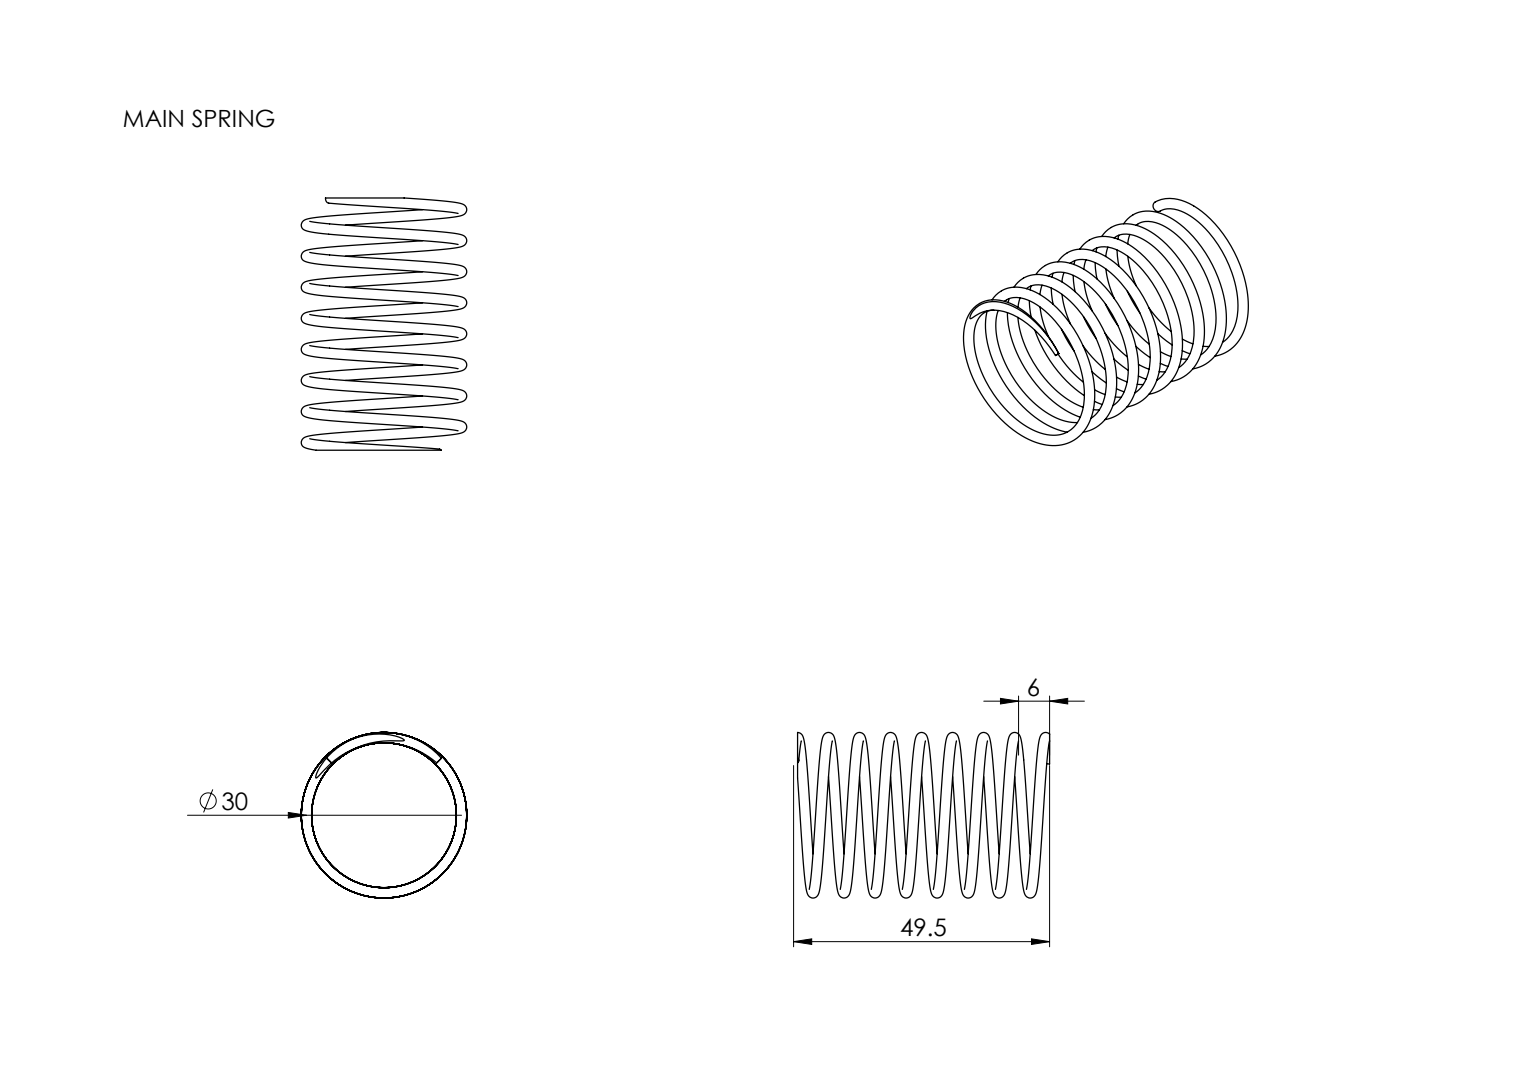
ISO-10303-21;
HEADER;
FILE_DESCRIPTION (('STEP AP214'),
    '1' );
FILE_NAME ('main spring.step',
    '2026-10-08T13:22:57',
    ( '' ),
    ( '' ),
    'SwSTEP 2.0',
    'SolidWorks 2026',
    '' );
FILE_SCHEMA (( 'AUTOMOTIVE_DESIGN' ));
ENDSEC;

DATA;
#2=CARTESIAN_POINT ( 'NONE',  ( 8.512513224245308763, 13.54758718765259040, 13.28571428571429003 ) ) ;
#5=CARTESIAN_POINT ( 'NONE',  ( -14.28433602490915000, 1.478298951650542481, 25.35310228751642470 ) ) ;
#11=CARTESIAN_POINT ( 'NONE',  ( -11.92174236212692051, -7.340858601238089420, 8.718326283912148256 ) ) ;
#12=CARTESIAN_POINT ( 'NONE',  ( 13.17239914596754424, -4.743843029824685864, 18.57546914105500235 ) ) ;
#15=CARTESIAN_POINT ( 'NONE',  ( 15.44746603149413922, 5.543385399275817527, 15.92453085894499409 ) ) ;
#16=COLOUR_RGB ( '', 0.40784314, 0.44705882, 0.49803922) ;
#20=CARTESIAN_POINT ( 'NONE',  ( 11.31370849898482334, -11.31370849898469366, 45.00000000000000711 ) ) ;
#25=CARTESIAN_POINT ( 'NONE',  ( -8.731428362939189114, 13.89598863503036341, 36.21428571428573662 ) ) ;
#28=CARTESIAN_POINT ( 'NONE',  ( -11.22385875690717327, 11.40355824106234550, 28.00404056962643651 ) ) ;
#30=CARTESIAN_POINT ( 'NONE',  ( -1.837501619626328297, 16.30827793483733856, 12.64285714285714235 ) ) ;
#35=CARTESIAN_POINT ( 'NONE',  ( -13.92619789766827054, -1.441234910513399470, 45.14689771248358596 ) ) ;
#36=CARTESIAN_POINT ( 'NONE',  ( 8.512513224245308763, 13.54758718765259040, 19.28571428571428825 ) ) ;
#38=CARTESIAN_POINT ( 'NONE',  ( -7.639999817571786700, 12.15899005565156266, 36.21428571428572951 ) ) ;
#39=CARTESIAN_POINT ( 'NONE',  ( 9.809645194534072132, -9.989344678689256796, 31.00404056962644006 ) ) ;
#43=CARTESIAN_POINT ( 'NONE',  ( 1.441234910513245149, 13.92619789766829008, 50.85310228751642825 ) ) ;
#46=CARTESIAN_POINT ( 'NONE',  ( 11.60466159355861926, 11.60466159355874716, 13.50000000000000355 ) ) ;
#48=CARTESIAN_POINT ( 'NONE',  ( -13.96533075980324234, 8.621071003556515677, 19.78167371608784819 ) ) ;
#53=FILL_AREA_STYLE_COLOUR ( '', #3926 ) ;
#56=CARTESIAN_POINT ( 'NONE',  ( 1.791431617652837316, 15.89939535829188877, 12.85714285714285943 ) ) ;
#59=CARTESIAN_POINT ( 'NONE',  ( 1.441234910513245149, 13.92619789766829008, 26.85310228751642470 ) ) ;
#63=CARTESIAN_POINT ( 'NONE',  ( 13.17239914596754424, -4.743843029824685864, 12.57546914105500768 ) ) ;
#64=CARTESIAN_POINT ( 'NONE',  ( -1.478298951650703019, 14.28433602490913579, 10.64689771248357886 ) ) ;
#68=CARTESIAN_POINT ( 'NONE',  ( 15.89939535829187278, 1.791431617653015174, 44.14285714285714590 ) ) ;
#77=CARTESIAN_POINT ( 'NONE',  ( -5.543385399275643444, -15.44746603149420494, 38.07546914105502367 ) ) ;
#79=CARTESIAN_POINT ( 'NONE',  ( -13.54758718765249625, -8.512513224245459753, 34.71428571428571530 ) ) ;
#80=CARTESIAN_POINT ( 'NONE',  ( 2.336471713481377055, 15.82515143223400145, 48.73000000000002530 ) ) ;
#82=SURFACE_STYLE_USAGE ( .BOTH. , #1640 ) ;
#85=CARTESIAN_POINT ( 'NONE',  ( -1.693770420379220099, -13.89774397934251837, 43.86118342676930126 ) ) ;
#86=CARTESIAN_POINT ( 'NONE',  ( 16.30827793483735633, -1.837501619626142890, 20.35714285714286476 ) ) ;
#87=CARTESIAN_POINT ( 'NONE',  ( -4.742819248065500481, -13.55419868402813499, 34.07142857142857650 ) ) ;
#88=CARTESIAN_POINT ( 'NONE',  ( -5.164528828830334817, 15.14410076328347543, -1.567388001802134223 ) ) ;
#89=CARTESIAN_POINT ( 'NONE',  ( -14.26974319298268767, 1.607813917172874918, 5.357142857142856762 ) ) ;
#93=CARTESIAN_POINT ( 'NONE',  ( -11.85413878919593422, -7.448449071214776396, 4.714285714285712636 ) ) ;
#96=CARTESIAN_POINT ( 'NONE',  ( -8.512513224245306986, -13.54758718765259218, 16.28571428571428470 ) ) ;
#97=CARTESIAN_POINT ( 'NONE',  ( -16.32287076676382398, 1.707986654103809343, 43.35310228751642825 ) ) ;
#101=CARTESIAN_POINT ( 'NONE',  ( 4.742819248065502258, 13.55419868402813499, 1.071428571428570065 ) ) ;
#104=CARTESIAN_POINT ( 'NONE',  ( -10.06191849875405531, -10.24623928997363542, 12.49595943037356349 ) ) ;
#107=CARTESIAN_POINT ( 'NONE',  ( 7.750357176954296712, -12.08964793087877787, 41.21024514465928235 ) ) ;
#112=CARTESIAN_POINT ( 'NONE',  ( -7.556039541191334585, -11.78653521626503320, 2.289754855340722539 ) ) ;
#114=CARTESIAN_POINT ( 'NONE',  ( 7.556039541191335474, 11.78653521626503320, 11.28975485534071943 ) ) ;
#118=CARTESIAN_POINT ( 'NONE',  ( 11.60466159355862104, 11.60466159355875071, 37.50000000000002842 ) ) ;
#124=CARTESIAN_POINT ( 'NONE',  ( 16.29368510291089223, -1.967016585148476882, 30.36118342676929771 ) ) ;
#126=CARTESIAN_POINT ( 'NONE',  ( -11.22385875690717327, 11.40355824106234550, 34.00404056962644006 ) ) ;
#128=CARTESIAN_POINT ( 'NONE',  ( 8.731428362939190890, -13.89598863503036164, 33.21428571428571530 ) ) ;
#130=CARTESIAN_POINT ( 'NONE',  ( 11.60466159355862104, 11.60466159355875071, 1.500000000000003553 ) ) ;
#133=( NAMED_UNIT ( * ) PLANE_ANGLE_UNIT ( ) SI_UNIT ( $, .RADIAN. ) );
#136=CARTESIAN_POINT ( 'NONE',  ( 5.164528828830335705, -15.14410076328347543, 1.432611998197868219 ) ) ;
#137=CARTESIAN_POINT ( 'NONE',  ( -1.791431617652833763, -15.89939535829188877, 21.85714285714286120 ) ) ;
#138=CARTESIAN_POINT ( 'NONE',  ( -11.85413878919593422, -7.448449071214776396, 34.71428571428571530 ) ) ;
#139=CARTESIAN_POINT ( 'NONE',  ( -9.809645194534070356, 9.989344678689256796, 46.00404056962644006 ) ) ;
#140=CARTESIAN_POINT ( 'NONE',  ( -7.639999817571787588, 12.15899005565156266, 12.21428571428571885 ) ) ;
#144=CARTESIAN_POINT ( 'NONE',  ( -11.78653521626494793, -7.556039541191465148, 48.71024514465926814 ) ) ;
#148=CARTESIAN_POINT ( 'NONE',  ( 1.791431617652837316, 15.89939535829188877, 18.85714285714285765 ) ) ;
#149=CARTESIAN_POINT ( 'NONE',  ( -15.14410076328353227, 5.164528828830164287, 31.56738800180213644 ) ) ;
#153=FILL_AREA_STYLE ('',( #53 ) ) ;
#155=CARTESIAN_POINT ( 'NONE',  ( -1.441234910513241818, -13.92619789766829008, 11.85310228751642470 ) ) ;
#158=CARTESIAN_POINT ( 'NONE',  ( 7.340858601237956194, 11.92174236212700045, 45.28167371608785174 ) ) ;
#163=CARTESIAN_POINT ( 'NONE',  ( 4.865839792409144771, 13.51115193377589740, 17.07546914105500591 ) ) ;
#165=CARTESIAN_POINT ( 'NONE',  ( -11.92174236212692051, -7.340858601238089420, 8.718326283912148256 ) ) ;
#168=CARTESIAN_POINT ( 'NONE',  ( -5.404401153735176599, 15.06016580658422477, 14.42453085894499232 ) ) ;
#176=CARTESIAN_POINT ( 'NONE',  ( 8.621071003556677326, -13.96533075980314287, 31.21832628391215536 ) ) ;
#179=CARTESIAN_POINT ( 'NONE',  ( 8.620103694221997515, 13.47998361472160767, 29.28975485534071765 ) ) ;
#184=CARTESIAN_POINT ( 'NONE',  ( -15.89939535829186923, -1.791431617653016062, 29.14285714285714235 ) ) ;
#185=CARTESIAN_POINT ( 'NONE',  ( -1.732852372895761661, 14.17511762181074353, 2.529641460854714575E-15 ) ) ;
#186=CARTESIAN_POINT ( 'NONE',  ( -5.420364854931999155, -15.49051278174644253, 22.07142857142858006 ) ) ;
#194=CARTESIAN_POINT ( 'NONE',  ( 12.08964793087886314, -7.750357176954162597, 42.78975485534072476 ) ) ;
#195=CARTESIAN_POINT ( 'NONE',  ( 8.731428362939190890, -13.89598863503036164, 9.214285714285717077 ) ) ;
#197=CARTESIAN_POINT ( 'NONE',  ( 4.503970704919991519, -13.25633410266674517, 43.43261199819787066 ) ) ;
#198=CARTESIAN_POINT ( 'NONE',  ( -1.567502665446231180, -13.91197093850540334, 9.857142857142855874 ) ) ;
#202=CARTESIAN_POINT ( 'NONE',  ( 4.742819248065503146, 13.55419868402813677, 7.071428571428569398 ) ) ;
#205=CARTESIAN_POINT ( 'NONE',  ( -9.899494936611716867, 9.899494936611610285, 0.000000000000000000 ) ) ;
#207=CARTESIAN_POINT ( 'NONE',  ( 15.10213328493390783, -5.284464991282587398, 14.57142857142856940 ) ) ;
#208=CARTESIAN_POINT ( 'NONE',  ( 5.404401153735178376, -15.06016580658422477, 35.42453085894499765 ) ) ;
#215=CARTESIAN_POINT ( 'NONE',  ( 4.743843029824831525, -13.17239914596749095, 41.42453085894499765 ) ) ;
#219=CARTESIAN_POINT ( 'NONE',  ( -4.503970704919988854, 13.25633410266674517, 22.43261199819786356 ) ) ;
#220=CARTESIAN_POINT ( 'NONE',  ( -13.92619789766827054, -1.441234910513399470, 15.14689771248357708 ) ) ;
#223=CARTESIAN_POINT ( 'NONE',  ( -11.40355824106246807, 11.22385875690704715, 7.995959430373565269 ) ) ;
#229=CARTESIAN_POINT ( 'NONE',  ( 1.917699372585825790, 15.88516839912900203, 34.86118342676929416 ) ) ;
#230=CARTESIAN_POINT ( 'NONE',  ( -14.26974319298268767, 1.607813917172874918, 29.35714285714285765 ) ) ;
#232=CARTESIAN_POINT ( 'NONE',  ( 5.543385399275644332, 15.44746603149420494, 41.07546914105501656 ) ) ;
#234=AXIS2_PLACEMENT_3D ( 'NONE', #895, #1048, #264 ) ;
#235=CARTESIAN_POINT ( 'NONE',  ( 1.791431617652837316, 15.89939535829188877, 24.85714285714285765 ) ) ;
#236=CARTESIAN_POINT ( 'NONE',  ( -0.4153140463578967601, 14.34878908348401971, 2.773985284965652638E-17 ) ) ;
#237=CARTESIAN_POINT ( 'NONE',  ( -1.837501619626328297, 16.30827793483733856, 18.64285714285715656 ) ) ;
#241=CARTESIAN_POINT ( 'NONE',  ( 11.31370849898482334, -11.31370849898469366, 39.00000000000000000 ) ) ;
#243=CARTESIAN_POINT ( 'NONE',  ( 15.91362231745475597, 1.665163862720026255, 0.1468977124835755543 ) ) ;
#244=CARTESIAN_POINT ( 'NONE',  ( 13.54758718765249803, 8.512513224245457977, 31.71428571428571530 ) ) ;
#245=CARTESIAN_POINT ( 'NONE',  ( 0.000000000000000000, 0.000000000000000000, 0.000000000000000000 ) ) ;
#246=CARTESIAN_POINT ( 'NONE',  ( 7.529642458189280241, -12.22833218042435099, 43.21832628391217668 ) ) ;
#247=CARTESIAN_POINT ( 'NONE',  ( -13.91197093850538380, -1.567502665446387278, 17.14285714285713880 ) ) ;
#251=CARTESIAN_POINT ( 'NONE',  ( 10.15407889436379030, 10.15407889436390576, 19.50000000000000355 ) ) ;
#255=CARTESIAN_POINT ( 'NONE',  ( 5.420364854932000931, 15.49051278174644075, 13.07142857142857117 ) ) ;
#256=CARTESIAN_POINT ( 'NONE',  ( 1.665163862719847732, 15.91362231745477374, 38.85310228751641404 ) ) ;
#260=CARTESIAN_POINT ( 'NONE',  ( 10.15407889436379030, 10.15407889436390221, 7.500000000000004441 ) ) ;
#262=CARTESIAN_POINT ( 'NONE',  ( -7.340858601237953529, -11.92174236212700222, 24.28167371608785530 ) ) ;
#264=DIRECTION ( 'NONE',  ( 0.7071067811865432429, 0.7071067811865519026, 0.000000000000000000 ) ) ;
#265=CARTESIAN_POINT ( 'NONE',  ( 12.22833218042443271, -7.529642458189144349, 34.78167371608785885 ) ) ;
#271=CARTESIAN_POINT ( 'NONE',  ( 13.59724543428031573, 4.619798703722006294, 23.93261199819786711 ) ) ;
#275=CARTESIAN_POINT ( 'NONE',  ( 15.44746603149413922, 5.543385399275817527, 3.924530858944990541 ) ) ;
#281=CARTESIAN_POINT ( 'NONE',  ( -11.22385875690717327, 11.40355824106234550, 34.00404056962644006 ) ) ;
#282=CARTESIAN_POINT ( 'NONE',  ( -13.55419868402807992, -4.742819248065651472, 34.92857142857145192 ) ) ;
#284=CARTESIAN_POINT ( 'NONE',  ( -4.742819248065502258, -13.55419868402813677, 34.07142857142859071 ) ) ;
#287=CARTESIAN_POINT ( 'NONE',  ( -5.420364854931999155, -15.49051278174644253, 28.07142857142857295 ) ) ;
#288=CARTESIAN_POINT ( 'NONE',  ( -3.668565799300981034, 13.66277435358085235, 2.529641460854714969E-15 ) ) ;
#289=CARTESIAN_POINT ( 'NONE',  ( -8.512513224245306986, -13.54758718765259218, 10.28571428571428648 ) ) ;
#294=CARTESIAN_POINT ( 'NONE',  ( -8.621071003556675549, 13.96533075980314642, 16.21832628391214470 ) ) ;
#295=CARTESIAN_POINT ( 'NONE',  ( 13.89598863503046111, -8.731428362939032795, 32.78571428571430602 ) ) ;
#298=CARTESIAN_POINT ( 'NONE',  ( -5.543385399275643444, -15.44746603149420494, 8.075469141055007682 ) ) ;
#299=CARTESIAN_POINT ( 'NONE',  ( -14.26974319298268767, 1.607813917172874918, 11.35714285714285943 ) ) ;
#303=CARTESIAN_POINT ( 'NONE',  ( -10.15407889436378852, -10.15407889436390576, 10.50000000000000533 ) ) ;
#305=CARTESIAN_POINT ( 'NONE',  ( 15.89939535829187278, 1.791431617653015174, 32.14285714285714590 ) ) ;
#306=CARTESIAN_POINT ( 'NONE',  ( 11.51250119794888249, 11.69682198916847682, 33.49595943037355994 ) ) ;
#309=CARTESIAN_POINT ( 'NONE',  ( -1.567502665446231180, -13.91197093850540334, 9.857142857142855874 ) ) ;
#312=CARTESIAN_POINT ( 'NONE',  ( 13.89774397934249706, 1.693770420379375308, 22.13881657323070939 ) ) ;
#315=CARTESIAN_POINT ( 'NONE',  ( 4.743843029824831525, -13.17239914596749095, 35.42453085894499765 ) ) ;
#320=CARTESIAN_POINT ( 'NONE',  ( -11.40355824106246807, 11.22385875690704715, 43.99595943037355994 ) ) ;
#322=CARTESIAN_POINT ( 'NONE',  ( -12.95959046474881227, 7.269551181504937176, 48.73000000000000398 ) ) ;
#323=CARTESIAN_POINT ( 'NONE',  ( 15.89939535829187278, 1.791431617653015174, 20.14285714285714235 ) ) ;
#324=CARTESIAN_POINT ( 'NONE',  ( 16.32287076676382043, -1.707986654103810897, 16.35310228751641759 ) ) ;
#332=CARTESIAN_POINT ( 'NONE',  ( 13.82664651025767100, -8.841785722321541030, 36.78975485534072476 ) ) ;
#333=CARTESIAN_POINT ( 'NONE',  ( 7.448449071214646722, 11.85413878919601594, 37.28571428571429180 ) ) ;
#334=CARTESIAN_POINT ( 'NONE',  ( -9.899494936611716867, 9.899494936611610285, 42.00000000000000000 ) ) ;
#337=CARTESIAN_POINT ( 'NONE',  ( -11.60466159355861926, -11.60466159355875249, 40.50000000000000711 ) ) ;
#338=CARTESIAN_POINT ( 'NONE',  ( -5.853818627049699685, 14.80933238498958282, -1.389475189636273717E-15 ) ) ;
#340=CARTESIAN_POINT ( 'NONE',  ( -15.89939535829186923, -1.791431617653016062, 23.14285714285714590 ) ) ;
#344=CARTESIAN_POINT ( 'NONE',  ( -11.69682198916834892, -11.51250119794901394, 8.504040569626438284 ) ) ;
#346=CARTESIAN_POINT ( 'NONE',  ( 15.49051278174638036, 5.420364854932175014, 25.92857142857142705 ) ) ;
#350=CARTESIAN_POINT ( 'NONE',  ( -1.707986654103994528, 16.32287076676380266, 10.64689771248357886 ) ) ;
#351=CARTESIAN_POINT ( 'NONE',  ( 13.91197093850538380, 1.567502665446386390, 26.14285714285714590 ) ) ;
#352=CARTESIAN_POINT ( 'NONE',  ( 16.30827793483735633, -1.837501619626142890, 8.357142857142855874 ) ) ;
#355=CARTESIAN_POINT ( 'NONE',  ( -13.91197093850538380, -1.567502665446387278, 17.14285714285713880 ) ) ;
#359=CARTESIAN_POINT ( 'NONE',  ( 11.31370849898482334, -11.31370849898469366, 27.00000000000000355 ) ) ;
#360=CARTESIAN_POINT ( 'NONE',  ( 1.665163862719847732, 15.91362231745477374, 50.85310228751642825 ) ) ;
#362=CARTESIAN_POINT ( 'NONE',  ( -13.55419868402807992, -4.742819248065651472, 10.92857142857143060 ) ) ;
#363=CARTESIAN_POINT ( 'NONE',  ( 11.78653521626494793, 7.556039541191463371, 33.71024514465927524 ) ) ;
#368=CARTESIAN_POINT ( 'NONE',  ( -1.737328882695368115, 14.25515036105620581, 50.63881657323071295 ) ) ;
#369=AXIS2_PLACEMENT_3D ( 'NONE', #442, #2961, #1373 ) ;
#373=CARTESIAN_POINT ( 'NONE',  ( -12.08964793087886314, 7.750357176954159932, 21.78975485534072476 ) ) ;
#375=CARTESIAN_POINT ( 'NONE',  ( 10.24623928997352884, 10.06191849875416899, 23.50404056962643295 ) ) ;
#377=CARTESIAN_POINT ( 'NONE',  ( 8.404922754268618235, 13.61519076058357491, 45.28167371608785174 ) ) ;
#378=EDGE_LOOP ( 'NONE', ( #1327, #9826 ) ) ;
#379=CARTESIAN_POINT ( 'NONE',  ( -11.25295468363732709, 9.057666965552700233, 48.73000000000003951 ) ) ;
#385=CARTESIAN_POINT ( 'NONE',  ( 4.742819248065503146, 13.55419868402813677, 25.07142857142858361 ) ) ;
#387=CARTESIAN_POINT ( 'NONE',  ( 4.742819248065503146, 13.55419868402813677, 43.07142857142858361 ) ) ;
#389=CARTESIAN_POINT ( 'NONE',  ( -5.284464991282755264, 15.10213328493384743, 42.42857142857143060 ) ) ;
#391=CARTESIAN_POINT ( 'NONE',  ( -11.60466159355861926, -11.60466159355875249, 10.50000000000000533 ) ) ;
#393=PRODUCT_DEFINITION_SHAPE ( 'NONE', 'NONE',  #8011 ) ;
#399=CARTESIAN_POINT ( 'NONE',  ( 1.917699372585825790, 15.88516839912900203, 4.861183426769296823 ) ) ;
#400=CARTESIAN_POINT ( 'NONE',  ( -8.731428362939189114, 13.89598863503036341, 36.21428571428573662 ) ) ;
#403=CARTESIAN_POINT ( 'NONE',  ( 5.543385399275644332, 15.44746603149420494, 11.07546914105500768 ) ) ;
#404=CARTESIAN_POINT ( 'NONE',  ( 7.448449071214646722, 11.85413878919601594, 19.28571428571428825 ) ) ;
#406=CARTESIAN_POINT ( 'NONE',  ( -13.89598863503046111, 8.731428362939027465, 47.78571428571430602 ) ) ;
#408=CARTESIAN_POINT ( 'NONE',  ( -12.15899005565164792, 7.639999817571651697, 17.78571428571428115 ) ) ;
#409=CARTESIAN_POINT ( 'NONE',  ( -11.60466159355861748, -11.60466159355874893, 28.50000000000000000 ) ) ;
#410=CARTESIAN_POINT ( 'NONE',  ( -16.32287076676382398, 1.707986654103809343, 49.35310228751642114 ) ) ;
#412=CARTESIAN_POINT ( 'NONE',  ( 4.742819248065502258, 13.55419868402813499, 7.071428571428569398 ) ) ;
#414=CARTESIAN_POINT ( 'NONE',  ( 13.89774397934249706, 1.693770420379375308, 28.13881657323070939 ) ) ;
#419=CARTESIAN_POINT ( 'NONE',  ( 7.340858601237956194, 11.92174236212700045, 51.28167371608785174 ) ) ;
#423=CARTESIAN_POINT ( 'NONE',  ( 4.865839792409144771, 13.51115193377589740, 29.07546914105501301 ) ) ;
#425=CARTESIAN_POINT ( 'NONE',  ( -16.32287076676382398, 1.707986654103809343, 43.35310228751642825 ) ) ;
#426=CARTESIAN_POINT ( 'NONE',  ( -5.462592421889175043, 15.04626098580285998, 48.73000000000003951 ) ) ;
#427=CARTESIAN_POINT ( 'NONE',  ( 5.420364854932001819, 15.49051278174644430, 25.07142857142858361 ) ) ;
#430=CARTESIAN_POINT ( 'NONE',  ( -9.989344678689363377, 9.809645194533960222, 13.99595943037356527 ) ) ;
#435=CARTESIAN_POINT ( 'NONE',  ( 16.29368510291089223, -1.967016585148476882, 36.36118342676930126 ) ) ;
#436=CARTESIAN_POINT ( 'NONE',  ( -9.899494936611716867, 9.899494936611610285, 24.00000000000000000 ) ) ;
#437=CARTESIAN_POINT ( 'NONE',  ( -4.623906867372410190, 13.21436662431711895, 42.42857142857143060 ) ) ;
#439=CARTESIAN_POINT ( 'NONE',  ( -13.89598863503046111, 8.731428362939027465, 47.78571428571430602 ) ) ;
#441=CARTESIAN_POINT ( 'NONE',  ( -8.731428362939189114, 13.89598863503036341, 36.21428571428573662 ) ) ;
#442=CARTESIAN_POINT ( 'NONE',  ( 0.000000000000000000, 18.00000000000000000, 0.000000000000000000 ) ) ;
#447=CARTESIAN_POINT ( 'NONE',  ( -5.164528828830334817, 15.14410076328347543, 4.432611998197859116 ) ) ;
#448=CARTESIAN_POINT ( 'NONE',  ( 8.512513224245308763, 13.54758718765259040, 25.28571428571428470 ) ) ;
#450=CARTESIAN_POINT ( 'NONE',  ( -15.53355953199861794, -5.297344310588530725, 2.932611998197868886 ) ) ;
#452=CARTESIAN_POINT ( 'NONE',  ( 14.26974319298268767, -1.607813917172876916, 26.35714285714285765 ) ) ;
#453=CARTESIAN_POINT ( 'NONE',  ( 1.791431617652837316, 15.89939535829188877, 6.857142857142860315 ) ) ;
#454=CARTESIAN_POINT ( 'NONE',  ( 1.837501619626330074, -16.30827793483733501, 39.64285714285716722 ) ) ;
#456=CARTESIAN_POINT ( 'NONE',  ( 9.899494936611718643, -9.899494936611608509, 15.00000000000000000 ) ) ;
#460=CARTESIAN_POINT ( 'NONE',  ( 15.89939535829187278, 1.791431617653015174, 38.14285714285714590 ) ) ;
#461=CARTESIAN_POINT ( 'NONE',  ( 8.404922754268618235, 13.61519076058357491, 45.28167371608785174 ) ) ;
#464=CARTESIAN_POINT ( 'NONE',  ( 13.55419868402807992, 4.742819248065649695, 7.928571428571430602 ) ) ;
#466=CARTESIAN_POINT ( 'NONE',  ( 4.743843029824831525, -13.17239914596749095, 23.42453085894499409 ) ) ;
#474=CARTESIAN_POINT ( 'NONE',  ( 13.96533075980324234, -8.621071003556521006, 40.78167371608785885 ) ) ;
#475=CARTESIAN_POINT ( 'NONE',  ( -10.53772368660228231, 9.764597359209851390, 48.73000000000002530 ) ) ;
#476=CARTESIAN_POINT ( 'NONE',  ( 11.31370849898482334, -11.31370849898469366, 21.00000000000000355 ) ) ;
#478=CARTESIAN_POINT ( 'NONE',  ( -9.989344678689363377, 9.809645194533960222, 19.99595943037356349 ) ) ;
#482=CARTESIAN_POINT ( 'NONE',  ( 15.53355953199861794, 5.297344310588528060, 41.93261199819787066 ) ) ;
#483=CARTESIAN_POINT ( 'NONE',  ( 12.15899005565164792, -7.639999817571655250, 44.78571428571428470 ) ) ;
#484=CARTESIAN_POINT ( 'NONE',  ( -7.448449071214644945, -11.85413878919601771, 34.28571428571428470 ) ) ;
#486=CARTESIAN_POINT ( 'NONE',  ( -8.841785722321695573, 13.82664651025757152, 2.210245144659280569 ) ) ;
#488=CARTESIAN_POINT ( 'NONE',  ( -15.49051278174638036, -5.420364854932175902, 28.92857142857143771 ) ) ;
#496=CARTESIAN_POINT ( 'NONE',  ( -16.29368510291090288, 1.967016585148476215, 15.36118342676929771 ) ) ;
#497=CARTESIAN_POINT ( 'NONE',  ( 15.89939535829187278, 1.791431617653015174, 38.14285714285714590 ) ) ;
#498=CARTESIAN_POINT ( 'NONE',  ( -15.53355953199861794, -5.297344310588530725, 8.932611998197868886 ) ) ;
#500=CARTESIAN_POINT ( 'NONE',  ( -13.91197093850538380, -1.567502665446387278, 23.14285714285714590 ) ) ;
#501=CARTESIAN_POINT ( 'NONE',  ( 1.837501619626330074, -16.30827793483733501, 9.642857142857147679 ) ) ;
#502=CARTESIAN_POINT ( 'NONE',  ( 1.791431617652837316, 15.89939535829188877, 48.85714285714286120 ) ) ;
#506=CARTESIAN_POINT ( 'NONE',  ( 5.420364854932000931, 15.49051278174644075, 31.07142857142857295 ) ) ;
#509=CARTESIAN_POINT ( 'NONE',  ( -1.967016585148659846, 16.29368510291087091, 50.63881657323071295 ) ) ;
#511=CARTESIAN_POINT ( 'NONE',  ( -15.10213328493390961, 5.284464991282586510, 5.571428571428574728 ) ) ;
#513=CARTESIAN_POINT ( 'NONE',  ( 11.85413878919593422, 7.448449071214774619, 31.71428571428571530 ) ) ;
#516=CARTESIAN_POINT ( 'NONE',  ( 9.989344678689365153, -9.809645194533958446, 34.99595943037355994 ) ) ;
#519=CARTESIAN_POINT ( 'NONE',  ( -13.96533075980324234, 8.621071003556515677, 7.781673716087849968 ) ) ;
#522=CARTESIAN_POINT ( 'NONE',  ( 11.78653521626494793, 7.556039541191463371, 45.71024514465928235 ) ) ;
#526=CARTESIAN_POINT ( 'NONE',  ( -4.865839792409144771, -13.51115193377589740, 26.07546914105500235 ) ) ;
#528=CARTESIAN_POINT ( 'NONE',  ( 16.32287076676382043, -1.707986654103810897, 40.35310228751642825 ) ) ;
#530=CARTESIAN_POINT ( 'NONE',  ( -8.057929360137700669, 13.68023991280794149, 48.73000000000005372 ) ) ;
#533=CARTESIAN_POINT ( 'NONE',  ( 4.619798703721856192, 13.59724543428036725, 21.06738800180213644 ) ) ;
#537=CARTESIAN_POINT ( 'NONE',  ( -1.707986654103994528, 16.32287076676380266, 40.64689771248358596 ) ) ;
#538=CARTESIAN_POINT ( 'NONE',  ( -14.26974319298268767, 1.607813917172874918, 41.35714285714286120 ) ) ;
#539=CARTESIAN_POINT ( 'NONE',  ( -13.17239914596754424, 4.743843029824683200, 3.575469141055005462 ) ) ;
#541=CARTESIAN_POINT ( 'NONE',  ( -8.512513224245306986, -13.54758718765259218, 40.28571428571428470 ) ) ;
#542=CARTESIAN_POINT ( 'NONE',  ( -11.31370849898482156, 11.31370849898469544, 0.000000000000000000 ) ) ;
#543=CARTESIAN_POINT ( 'NONE',  ( 13.54758718765249803, 8.512513224245457977, 25.71428571428571885 ) ) ;
#551=CARTESIAN_POINT ( 'NONE',  ( 5.543385399275644332, 15.44746603149420494, 17.07546914105500591 ) ) ;
#552=CARTESIAN_POINT ( 'NONE',  ( 11.31370849898482334, -11.31370849898469366, 45.00000000000000711 ) ) ;
#553=CARTESIAN_POINT ( 'NONE',  ( -8.620103694221995738, -13.47998361472161299, 26.28975485534072831 ) ) ;
#554=CARTESIAN_POINT ( 'NONE',  ( 4.742819248065503146, 13.55419868402813677, 19.07142857142856940 ) ) ;
#555=CARTESIAN_POINT ( 'NONE',  ( -13.89598863503046111, 8.731428362939027465, 5.785714285714282035 ) ) ;
#556=CARTESIAN_POINT ( 'NONE',  ( -13.89598863503046111, 8.731428362939027465, 41.78571428571430602 ) ) ;
#560=CARTESIAN_POINT ( 'NONE',  ( 1.837501619626329630, -16.30827793483733501, 39.64285714285715301 ) ) ;
#562=CARTESIAN_POINT ( 'NONE',  ( 15.44746603149413922, 5.543385399275817527, 45.92453085894500475 ) ) ;
#564=CARTESIAN_POINT ( 'NONE',  ( 15.10213328493390783, -5.284464991282587398, 2.571428571428571619 ) ) ;
#565=CARTESIAN_POINT ( 'NONE',  ( 15.10213328493390783, -5.284464991282587398, 8.571428571428569398 ) ) ;
#567=CARTESIAN_POINT ( 'NONE',  ( -13.91197093850538380, -1.567502665446387278, 23.14285714285714590 ) ) ;
#569=CARTESIAN_POINT ( 'NONE',  ( 13.51115193377584589, 4.865839792409294873, 45.92453085894500475 ) ) ;
#573=CARTESIAN_POINT ( 'NONE',  ( 1.665163862719847732, 15.91362231745477374, 20.85310228751641759 ) ) ;
#576=CARTESIAN_POINT ( 'NONE',  ( 1.441234910513245149, 13.92619789766829008, 50.85310228751642825 ) ) ;
#582=CARTESIAN_POINT ( 'NONE',  ( 5.404401153735178376, -15.06016580658422477, 47.42453085894499765 ) ) ;
#584=CARTESIAN_POINT ( 'NONE',  ( 5.284464991282756152, -15.10213328493384743, 27.42857142857143060 ) ) ;
#587=CARTESIAN_POINT ( 'NONE',  ( -7.750357176954294935, 12.08964793087877787, 20.21024514465928235 ) ) ;
#591=CARTESIAN_POINT ( 'NONE',  ( 13.82664651025767100, -8.841785722321541030, 42.78975485534072476 ) ) ;
#592=CARTESIAN_POINT ( 'NONE',  ( -4.742819248065502258, -13.55419868402813677, 46.07142857142856940 ) ) ;
#593=CARTESIAN_POINT ( 'NONE',  ( 13.21436662431716869, -4.623906867372263640, 44.57142857142857650 ) ) ;
#595=CARTESIAN_POINT ( 'NONE',  ( -5.404401153735176599, 15.06016580658422477, 8.424530858944992318 ) ) ;
#597=CARTESIAN_POINT ( 'NONE',  ( -13.54758718765249625, -8.512513224245459753, 28.71428571428571530 ) ) ;
#604=CARTESIAN_POINT ( 'NONE',  ( 8.731428362939190890, -13.89598863503036164, 45.21428571428572951 ) ) ;
#606=CARTESIAN_POINT ( 'NONE',  ( -11.22385875690717327, 11.40355824106234550, 16.00404056962643651 ) ) ;
#608=CARTESIAN_POINT ( 'NONE',  ( -1.607813917173034124, 14.26974319298267524, 30.64285714285715301 ) ) ;
#610=CARTESIAN_POINT ( 'NONE',  ( 11.60466159355862104, 11.60466159355875071, 13.50000000000000178 ) ) ;
#611=CARTESIAN_POINT ( 'NONE',  ( -11.31370849898482156, 11.31370849898469544, 48.00000000000000000 ) ) ;
#615=CARTESIAN_POINT ( 'NONE',  ( -5.284464991282755264, 15.10213328493384743, 48.42857142857143060 ) ) ;
#618=CARTESIAN_POINT ( 'NONE',  ( 13.89598863503046111, -8.731428362939032795, 8.785714285714293581 ) ) ;
#619=CARTESIAN_POINT ( 'NONE',  ( -5.284464991282755264, 15.10213328493384743, 0.4285714285714309346 ) ) ;
#621=CARTESIAN_POINT ( 'NONE',  ( 7.639999817571788476, -12.15899005565156266, 21.21428571428571530 ) ) ;
#622=CARTESIAN_POINT ( 'NONE',  ( 1.478298951650704351, -14.28433602490913579, 25.64689771248357886 ) ) ;
#624=CARTESIAN_POINT ( 'NONE',  ( -7.750357176954294935, 12.08964793087877787, 44.21024514465928235 ) ) ;
#627=CARTESIAN_POINT ( 'NONE',  ( 8.841785722321695573, -13.82664651025757152, 17.21024514465927879 ) ) ;
#628=CARTESIAN_POINT ( 'NONE',  ( -8.731428362939187338, 13.89598863503036164, 0.2142857142857168273 ) ) ;
#630=CARTESIAN_POINT ( 'NONE',  ( -16.32287076676382398, 1.707986654103809343, 19.35310228751642825 ) ) ;
#634=CARTESIAN_POINT ( 'NONE',  ( 14.25515036105622535, -1.737328882695210241, 30.36118342676929771 ) ) ;
#636=CARTESIAN_POINT ( 'NONE',  ( -13.51115193377584589, -4.865839792409295761, 6.924530858944994982 ) ) ;
#638=CARTESIAN_POINT ( 'NONE',  ( -15.10213328493390961, 5.284464991282586510, 29.57142857142857650 ) ) ;
#641=CARTESIAN_POINT ( 'NONE',  ( 7.750357176954296712, -12.08964793087877787, 11.21024514465928235 ) ) ;
#645=CARTESIAN_POINT ( 'NONE',  ( 9.899494936611718643, -9.899494936611608509, 45.00000000000000711 ) ) ;
#646=CARTESIAN_POINT ( 'NONE',  ( -7.556039541191334585, -11.78653521626503320, 2.289754855340722539 ) ) ;
#648=CARTESIAN_POINT ( 'NONE',  ( -15.44746603149413922, -5.543385399275820191, 12.92453085894499587 ) ) ;
#650=CARTESIAN_POINT ( 'NONE',  ( -16.30827793483735988, 1.837501619626141780, 29.35714285714285765 ) ) ;
#657=CARTESIAN_POINT ( 'NONE',  ( -1.837501619626328297, 16.30827793483733856, 48.64285714285716011 ) ) ;
#659=CARTESIAN_POINT ( 'NONE',  ( -8.621071003556675549, 13.96533075980314642, 16.21832628391214470 ) ) ;
#660=CARTESIAN_POINT ( 'NONE',  ( -1.791431617652833763, -15.89939535829188877, 15.85714285714286120 ) ) ;
#665=CARTESIAN_POINT ( 'NONE',  ( -15.89939535829186923, -1.791431617653016062, 41.14285714285714590 ) ) ;
#668=CARTESIAN_POINT ( 'NONE',  ( 8.512513224245308763, 13.54758718765259040, 1.285714285714285809 ) ) ;
#669=CARTESIAN_POINT ( 'NONE',  ( -13.89598863503046111, 8.731428362939027465, 5.785714285714282035 ) ) ;
#670=CARTESIAN_POINT ( 'NONE',  ( -1.567502665446231180, -13.91197093850540334, 27.85714285714285765 ) ) ;
#671=CARTESIAN_POINT ( 'NONE',  ( 7.556039541191335474, 11.78653521626503320, 29.28975485534071765 ) ) ;
#673=ORIENTED_EDGE ( 'NONE', *, *, #6657, .T. ) ;
#674=CARTESIAN_POINT ( 'NONE',  ( -7.340858601237953529, -11.92174236212700222, 42.28167371608785174 ) ) ;
#678=CARTESIAN_POINT ( 'NONE',  ( 15.14410076328353227, -5.164528828830166063, 22.56738800180214000 ) ) ;
#680=CARTESIAN_POINT ( 'NONE',  ( -5.420364854931998266, -15.49051278174643898, 4.071428571428569398 ) ) ;
#682=CARTESIAN_POINT ( 'NONE',  ( -15.44746603149413922, -5.543385399275820191, 24.92453085894499765 ) ) ;
#686=CARTESIAN_POINT ( 'NONE',  ( -4.503970704919988854, 13.25633410266674517, 46.43261199819787066 ) ) ;
#691=CARTESIAN_POINT ( 'NONE',  ( -13.89774397934249706, -1.693770420379375974, 7.138816573230711171 ) ) ;
#693=CARTESIAN_POINT ( 'NONE',  ( -11.31370849898482156, 11.31370849898469544, 30.00000000000000355 ) ) ;
#696=CARTESIAN_POINT ( 'NONE',  ( -13.51115193377584589, -4.865839792409295761, 30.92453085894499765 ) ) ;
#700=CARTESIAN_POINT ( 'NONE',  ( 4.503970704919991519, -13.25633410266674517, 7.432611998197861780 ) ) ;
#701=CARTESIAN_POINT ( 'NONE',  ( 1.693770420379222319, 13.89774397934251837, -1.138816573230706286 ) ) ;
#703=CARTESIAN_POINT ( 'NONE',  ( -11.40355824106246807, 11.22385875690704715, 13.99595943037356527 ) ) ;
#705=CARTESIAN_POINT ( 'NONE',  ( 13.54758718765249803, 8.512513224245457977, 37.71428571428571530 ) ) ;
#711=CARTESIAN_POINT ( 'NONE',  ( 11.31370849898482334, -11.31370849898469366, 39.00000000000000000 ) ) ;
#712=CARTESIAN_POINT ( 'NONE',  ( -5.164528828830334817, 15.14410076328347543, 16.43261199819786356 ) ) ;
#713=CARTESIAN_POINT ( 'NONE',  ( -11.60466159355861926, -11.60466159355875249, 22.50000000000000000 ) ) ;
#718=CARTESIAN_POINT ( 'NONE',  ( -13.89598863503045933, 8.731428362939027465, 47.78571428571429891 ) ) ;
#721=CARTESIAN_POINT ( 'NONE',  ( 5.284464991282756152, -15.10213328493384743, 3.428571428571426605 ) ) ;
#722=CARTESIAN_POINT ( 'NONE',  ( -8.731428362939189114, 13.89598863503036341, 0.2142857142857168273 ) ) ;
#723=CARTESIAN_POINT ( 'NONE',  ( 7.448449071214646722, 11.85413878919601594, 31.28571428571428470 ) ) ;
#724=CARTESIAN_POINT ( 'NONE',  ( 12.08964793087886314, -7.750357176954162597, 36.78975485534072476 ) ) ;
#727=CARTESIAN_POINT ( 'NONE',  ( 13.25633410266679313, -4.503970704919842305, 40.56738800180214355 ) ) ;
#730=CARTESIAN_POINT ( 'NONE',  ( -11.51250119794888072, -11.69682198916848037, 24.49595943037356705 ) ) ;
#731=CARTESIAN_POINT ( 'NONE',  ( 1.791431617652837316, 15.89939535829188877, 0.8571428571428549859 ) ) ;
#733=CARTESIAN_POINT ( 'NONE',  ( 13.47998361472151529, 8.620103694222146729, 21.71024514465928235 ) ) ;
#739=CARTESIAN_POINT ( 'NONE',  ( 11.22385875690704715, 11.40355824106246985, 51.49595943037355994 ) ) ;
#742=CARTESIAN_POINT ( 'NONE',  ( 13.89598863503046111, -8.731428362939032795, 26.78571428571429536 ) ) ;
#747=CARTESIAN_POINT ( 'NONE',  ( 10.13893307789800957, 12.50873118924980609, 47.39553751340654486 ) ) ;
#748=CARTESIAN_POINT ( 'NONE',  ( -14.25515036105622890, 1.737328882695209575, 9.361183426769292382 ) ) ;
#749=CARTESIAN_POINT ( 'NONE',  ( 10.24623928997352884, 10.06191849875416899, -0.4959594303735606058 ) ) ;
#751=CARTESIAN_POINT ( 'NONE',  ( 11.51250119794888249, 11.69682198916847682, 3.495959430373559940 ) ) ;
#753=CARTESIAN_POINT ( 'NONE',  ( 8.512513224245308763, 13.54758718765259040, 43.28571428571429180 ) ) ;
#759=CARTESIAN_POINT ( 'NONE',  ( -8.620103694221995738, -13.47998361472161299, 20.28975485534072121 ) ) ;
#761=CARTESIAN_POINT ( 'NONE',  ( 11.22385875690717683, -11.40355824106234373, 19.00404056962642940 ) ) ;
#762=CARTESIAN_POINT ( 'NONE',  ( 6.903294689124716221, 14.32703841502055830, 48.72999999999998266 ) ) ;
#764=CARTESIAN_POINT ( 'NONE',  ( -15.49051278174637858, -5.420364854932175014, 46.92857142857143060 ) ) ;
#767=CARTESIAN_POINT ( 'NONE',  ( -1.791431617652833763, -15.89939535829188877, 9.857142857142855874 ) ) ;
#768=CARTESIAN_POINT ( 'NONE',  ( 13.91197093850538380, 1.567502665446386390, 32.14285714285714590 ) ) ;
#770=CARTESIAN_POINT ( 'NONE',  ( -13.17239914596754424, 4.743843029824683200, 33.57546914105500946 ) ) ;
#773=CARTESIAN_POINT ( 'NONE',  ( 14.26974319298268767, -1.607813917172876916, 2.357142857142856762 ) ) ;
#776=CARTESIAN_POINT ( 'NONE',  ( -1.665163862719845067, -15.91362231745477374, 23.85310228751642825 ) ) ;
#777=CARTESIAN_POINT ( 'NONE',  ( 5.284464991282756152, -15.10213328493384743, 3.428571428571426605 ) ) ;
#778=CARTESIAN_POINT ( 'NONE',  ( -15.88516839912898071, -1.917699372586004980, 19.13881657323070584 ) ) ;
#783=CARTESIAN_POINT ( 'NONE',  ( -1.791431617652833763, -15.89939535829188877, 33.85714285714285410 ) ) ;
#785=CARTESIAN_POINT ( 'NONE',  ( 7.750357176954296712, -12.08964793087877787, 5.210245144659280569 ) ) ;
#787=CARTESIAN_POINT ( 'NONE',  ( 15.49051278174638036, 5.420364854932175014, 13.92857142857143238 ) ) ;
#793=CARTESIAN_POINT ( 'NONE',  ( 9.809645194534072132, -9.989344678689256796, 7.004040569626434731 ) ) ;
#794=CARTESIAN_POINT ( 'NONE',  ( 13.59724543428031573, 4.619798703722006294, 17.93261199819786711 ) ) ;
#796=CARTESIAN_POINT ( 'NONE',  ( -11.40355824106246807, 11.22385875690704715, 7.995959430373565269 ) ) ;
#798=CARTESIAN_POINT ( 'NONE',  ( 1.791431617652837316, 15.89939535829188877, 42.85714285714285410 ) ) ;
#804=CARTESIAN_POINT ( 'NONE',  ( -15.49051278174638036, -5.420364854932175902, 34.92857142857145192 ) ) ;
#807=CARTESIAN_POINT ( 'NONE',  ( 15.91362231745475597, 1.665163862720026255, 36.14689771248357886 ) ) ;
#809=CARTESIAN_POINT ( 'NONE',  ( 5.420364854932001819, 15.49051278174644430, 19.07142857142856940 ) ) ;
#811=CARTESIAN_POINT ( 'NONE',  ( -1.791431617652833763, -15.89939535829188877, 3.857142857142857650 ) ) ;
#815=CARTESIAN_POINT ( 'NONE',  ( -9.809645194534070356, 9.989344678689256796, 46.00404056962644006 ) ) ;
#816=CARTESIAN_POINT ( 'NONE',  ( 16.30827793483735633, -1.837501619626142890, 14.35714285714285587 ) ) ;
#817=CARTESIAN_POINT ( 'NONE',  ( -7.448449071214644945, -11.85413878919601771, 40.28571428571428470 ) ) ;
#818=CARTESIAN_POINT ( 'NONE',  ( 10.24623928997352884, 10.06191849875416899, 29.50404056962643295 ) ) ;
#822=CARTESIAN_POINT ( 'NONE',  ( -9.989344678689363377, 9.809645194533960222, 49.99595943037357415 ) ) ;
#824=CARTESIAN_POINT ( 'NONE',  ( -8.841785722321695573, 13.82664651025757152, 32.21024514465928235 ) ) ;
#825=CARTESIAN_POINT ( 'NONE',  ( -11.60466159355861748, -11.60466159355874893, 22.50000000000000355 ) ) ;
#827=CARTESIAN_POINT ( 'NONE',  ( -5.297344310588352201, -15.53355953199867301, 18.06738800180213644 ) ) ;
#831=SURFACE_STYLE_USAGE ( .BOTH. , #8689 ) ;
#835=CARTESIAN_POINT ( 'NONE',  ( -13.51115193377584589, -4.865839792409295761, 18.92453085894499409 ) ) ;
#845=CARTESIAN_POINT ( 'NONE',  ( 13.59724543428031573, 4.619798703722006294, 11.93261199819786178 ) ) ;
#846=CARTESIAN_POINT ( 'NONE',  ( -7.556039541191334585, -11.78653521626503320, 8.289754855340721207 ) ) ;
#852=CARTESIAN_POINT ( 'NONE',  ( 5.420364854932001819, 15.49051278174644430, 43.07142857142858361 ) ) ;
#858=CARTESIAN_POINT ( 'NONE',  ( 8.621071003556677326, -13.96533075980314287, 25.21832628391215181 ) ) ;
#861=CARTESIAN_POINT ( 'NONE',  ( 1.707986654103998303, -16.32287076676380266, 31.64689771248358241 ) ) ;
#864=CARTESIAN_POINT ( 'NONE',  ( -11.60466159355861926, -11.60466159355875249, 28.50000000000001066 ) ) ;
#871=CARTESIAN_POINT ( 'NONE',  ( -1.478298951650703019, 14.28433602490913579, 40.64689771248358596 ) ) ;
#872=CARTESIAN_POINT ( 'NONE',  ( -5.420364854931999155, -15.49051278174644253, 16.07142857142857650 ) ) ;
#874=CARTESIAN_POINT ( 'NONE',  ( -12.15899005565164792, 7.639999817571650809, 35.78571428571429180 ) ) ;
#875=CARTESIAN_POINT ( 'NONE',  ( 11.92174236212692229, 7.340858601238088532, 41.71832628391215536 ) ) ;
#876=CARTESIAN_POINT ( 'NONE',  ( -7.529642458189277576, 12.22833218042435455, 34.21832628391215536 ) ) ;
#880=CARTESIAN_POINT ( 'NONE',  ( -1.567502665446231180, -13.91197093850540334, 3.857142857142857650 ) ) ;
#884=CARTESIAN_POINT ( 'NONE',  ( 1.837501619626329630, -16.30827793483733501, 21.64285714285714590 ) ) ;
#886=CARTESIAN_POINT ( 'NONE',  ( -13.47998361472151174, -8.620103694222146729, 42.71024514465928235 ) ) ;
#893=CARTESIAN_POINT ( 'NONE',  ( 13.89774397934249706, 1.693770420379375308, 10.13881657323070762 ) ) ;
#895=CARTESIAN_POINT ( 'NONE',  ( 10.60660171779815464, 10.60660171779826833, 49.50000000000000000 ) ) ;
#896=CARTESIAN_POINT ( 'NONE',  ( 12.22833218042443271, -7.529642458189144349, 28.78167371608785174 ) ) ;
#900=CARTESIAN_POINT ( 'NONE',  ( -13.59724543428031573, -4.619798703722008959, 2.932611998197868886 ) ) ;
#901=CARTESIAN_POINT ( 'NONE',  ( 7.556039541191335474, 11.78653521626503320, 17.28975485534072121 ) ) ;
#904=DIRECTION ( 'NONE',  ( -0.7071067811865431318, -0.7071067811865519026, 0.000000000000000000 ) ) ;
#905=CARTESIAN_POINT ( 'NONE',  ( 1.837501619626330074, -16.30827793483733501, 39.64285714285716722 ) ) ;
#910=CARTESIAN_POINT ( 'NONE',  ( 15.53355953199861794, 5.297344310588528060, 29.93261199819786356 ) ) ;
#912=CARTESIAN_POINT ( 'NONE',  ( -15.91362231745475597, -1.665163862720028254, 27.14689771248358241 ) ) ;
#914=CARTESIAN_POINT ( 'NONE',  ( 8.512513224245308763, 13.54758718765259040, 25.28571428571428470 ) ) ;
#916=CARTESIAN_POINT ( 'NONE',  ( -15.10213328493390961, 5.284464991282586510, 5.571428571428574728 ) ) ;
#921=CARTESIAN_POINT ( 'NONE',  ( -13.61519076058348254, -8.404922754268771001, 2.718326283912150476 ) ) ;
#922=CARTESIAN_POINT ( 'NONE',  ( 5.284464991282756152, -15.10213328493384743, 21.42857142857142705 ) ) ;
#923=CARTESIAN_POINT ( 'NONE',  ( -4.742819248065500481, -13.55419868402813499, 40.07142857142857650 ) ) ;
#924=CARTESIAN_POINT ( 'NONE',  ( 9.809645194534072132, -9.989344678689256796, 37.00404056962644006 ) ) ;
#925=CARTESIAN_POINT ( 'NONE',  ( 1.567502665446232957, 13.91197093850540156, 12.85714285714285943 ) ) ;
#929=CARTESIAN_POINT ( 'NONE',  ( -10.06191849875405531, -10.24623928997363542, 48.49595943037355994 ) ) ;
#933=CARTESIAN_POINT ( 'NONE',  ( 13.89598863503045933, -8.731428362939032795, 14.78571428571429180 ) ) ;
#934=CARTESIAN_POINT ( 'NONE',  ( -11.40355824106246807, 11.22385875690704715, 37.99595943037355994 ) ) ;
#937=CARTESIAN_POINT ( 'NONE',  ( 13.91197093850538380, 1.567502665446386390, 2.142857142857140573 ) ) ;
#939=ADVANCED_BREP_SHAPE_REPRESENTATION ( '', ( #7077, #3995 ), #5075 ) ;
#941=CARTESIAN_POINT ( 'NONE',  ( 14.28433602490915000, -1.478298951650544479, 10.35310228751642292 ) ) ;
#944=CARTESIAN_POINT ( 'NONE',  ( 11.60466159355862104, 11.60466159355875071, 37.50000000000002842 ) ) ;
#945=CARTESIAN_POINT ( 'NONE',  ( 11.78653521626494793, 7.556039541191463371, 33.71024514465927524 ) ) ;
#949=CARTESIAN_POINT ( 'NONE',  ( 12.08964793087886314, -7.750357176954162597, 18.78975485534072121 ) ) ;
#950=CARTESIAN_POINT ( 'NONE',  ( -4.865839792409144771, -13.51115193377589740, 8.075469141055007682 ) ) ;
#953=CARTESIAN_POINT ( 'NONE',  ( 8.404922754268618235, 13.61519076058357491, 3.281673716087854409 ) ) ;
#959=CARTESIAN_POINT ( 'NONE',  ( -8.621071003556675549, 13.96533075980314642, 28.21832628391215181 ) ) ;
#961=CARTESIAN_POINT ( 'NONE',  ( 8.621071003556677326, -13.96533075980314287, 31.21832628391215536 ) ) ;
#963=CARTESIAN_POINT ( 'NONE',  ( 8.512513224245308763, 13.54758718765259040, 37.28571428571429180 ) ) ;
#964=CARTESIAN_POINT ( 'NONE',  ( 3.284785595323101770, 14.94556295727555906, 6.336793937239290789E-15 ) ) ;
#965=CARTESIAN_POINT ( 'NONE',  ( 1.837501619626330074, -16.30827793483733501, 3.642857142857144126 ) ) ;
#971=CARTESIAN_POINT ( 'NONE',  ( 1.693770420379222319, 13.89774397934251837, 40.86118342676929416 ) ) ;
#972=CARTESIAN_POINT ( 'NONE',  ( 1.791431617652837316, 15.89939535829188877, 12.85714285714285943 ) ) ;
#973=CARTESIAN_POINT ( 'NONE',  ( 11.85413878919593422, 7.448449071214774619, 43.71428571428572241 ) ) ;
#974=CARTESIAN_POINT ( 'NONE',  ( 4.865839792409144771, 13.51115193377589740, 47.07546914105501656 ) ) ;
#975=CARTESIAN_POINT ( 'NONE',  ( 7.448449071214646722, 11.85413878919601594, 13.28571428571429003 ) ) ;
#979=CARTESIAN_POINT ( 'NONE',  ( 11.85413878919593422, 7.448449071214774619, 7.714285714285715301 ) ) ;
#982=CARTESIAN_POINT ( 'NONE',  ( -5.284464991282755264, 15.10213328493384743, 12.42857142857142705 ) ) ;
#983=CARTESIAN_POINT ( 'NONE',  ( -15.44746603149413922, -5.543385399275820191, 36.92453085894499765 ) ) ;
#986=CARTESIAN_POINT ( 'NONE',  ( 1.607813917173037899, -14.26974319298267169, 3.642857142857143238 ) ) ;
#988=CARTESIAN_POINT ( 'NONE',  ( -13.25633410266679313, 4.503970704919840529, 13.56738800180213822 ) ) ;
#990=CARTESIAN_POINT ( 'NONE',  ( -13.89598863503046111, 8.731428362939027465, 11.78571428571428115 ) ) ;
#996=CARTESIAN_POINT ( 'NONE',  ( -13.17239914596754424, 4.743843029824683200, 21.57546914105500946 ) ) ;
#998=CARTESIAN_POINT ( 'NONE',  ( 14.25515036105622535, -1.737328882695210241, 12.36118342676929771 ) ) ;
#1001=CARTESIAN_POINT ( 'NONE',  ( 8.404922754268618235, 13.61519076058357491, 15.28167371608785174 ) ) ;
#1009=CARTESIAN_POINT ( 'NONE',  ( 15.06016580658428694, -5.404401153735007846, 36.57546914105501656 ) ) ;
#1010=CARTESIAN_POINT ( 'NONE',  ( 13.55419868402807992, 4.742819248065648807, 25.92857142857142705 ) ) ;
#1011=CARTESIAN_POINT ( 'NONE',  ( -1.707986654103994528, 16.32287076676380266, 40.64689771248358596 ) ) ;
#1015=CARTESIAN_POINT ( 'NONE',  ( -15.10213328493390961, 5.284464991282586510, 35.57142857142857650 ) ) ;
#1016=CARTESIAN_POINT ( 'NONE',  ( -8.918407633172652282, 10.81660888964814049, -5.255698201876050631E-17 ) ) ;
#1017=CARTESIAN_POINT ( 'NONE',  ( -16.30827793483735988, 1.837501619626141780, 11.35714285714285943 ) ) ;
#1023=CARTESIAN_POINT ( 'NONE',  ( 13.17239914596754424, -4.743843029824685864, 42.57546914105501656 ) ) ;
#1024=CARTESIAN_POINT ( 'NONE',  ( -11.31370849898482156, 11.31370849898469544, 36.00000000000000711 ) ) ;
#1025=CARTESIAN_POINT ( 'NONE',  ( -11.85413878919593422, -7.448449071214776396, 46.71428571428571530 ) ) ;
#1026=CARTESIAN_POINT ( 'NONE',  ( 13.59724543428031573, 4.619798703722006294, 35.93261199819787066 ) ) ;
#1029=CARTESIAN_POINT ( 'NONE',  ( 7.639999817571789364, -12.15899005565156266, 15.21428571428571530 ) ) ;
#1033=CARTESIAN_POINT ( 'NONE',  ( 4.623906867372411078, -13.21436662431711717, 21.42857142857142705 ) ) ;
#1034=VECTOR ( 'NONE', #9669, 1000.000000000000114 ) ;
#1038=CARTESIAN_POINT ( 'NONE',  ( -13.54758718765249625, -8.512513224245459753, 22.71428571428571530 ) ) ;
#1039=CARTESIAN_POINT ( 'NONE',  ( -8.404922754268618235, -13.61519076058357491, 36.28167371608785174 ) ) ;
#1042=CARTESIAN_POINT ( 'NONE',  ( 4.742819248065502258, 13.55419868402813499, 13.07142857142857117 ) ) ;
#1043=CARTESIAN_POINT ( 'NONE',  ( -13.89774397934249706, -1.693770420379375974, 13.13881657323070584 ) ) ;
#1048=DIRECTION ( 'NONE',  ( -0.7056782240951974261, 0.7056782240951879892, -0.06353336191096842223 ) ) ;
#1049=CARTESIAN_POINT ( 'NONE',  ( 1.737328882695370558, -14.25515036105620581, 41.63881657323070584 ) ) ;
#1053=CARTESIAN_POINT ( 'NONE',  ( -7.556039541191334585, -11.78653521626503320, 14.28975485534072298 ) ) ;
#1056=CARTESIAN_POINT ( 'NONE',  ( -4.865839792409144771, -13.51115193377589740, 20.07546914105500591 ) ) ;
#1058=CARTESIAN_POINT ( 'NONE',  ( 15.88516839912898071, 1.917699372586004092, 16.13881657323070584 ) ) ;
#1065=CARTESIAN_POINT ( 'NONE',  ( -1.567502665446231180, -13.91197093850540334, 27.85714285714285765 ) ) ;
#1066=CARTESIAN_POINT ( 'NONE',  ( -13.55419868402807992, -4.742819248065651472, 34.92857142857145192 ) ) ;
#1069=CARTESIAN_POINT ( 'NONE',  ( 3.272017905259138715, 14.35386563642104107, 8.096169431371285764E-17 ) ) ;
#1071=CARTESIAN_POINT ( 'NONE',  ( -1.791431617652833763, -15.89939535829188877, 21.85714285714286120 ) ) ;
#1077=CARTESIAN_POINT ( 'NONE',  ( 8.620103694221997515, 13.47998361472160767, 11.28975485534071943 ) ) ;
#1078=CARTESIAN_POINT ( 'NONE',  ( -5.284464991282755264, 15.10213328493384743, 30.42857142857143060 ) ) ;
#1080=CARTESIAN_POINT ( 'NONE',  ( -1.917699372585823570, -15.88516839912900558, 7.861183426769288829 ) ) ;
#1081=CARTESIAN_POINT ( 'NONE',  ( 10.15407889436379030, 10.15407889436390576, 7.500000000000005329 ) ) ;
#1085=CARTESIAN_POINT ( 'NONE',  ( -14.26974319298268767, 1.607813917172874918, 23.35714285714286476 ) ) ;
#1087=CARTESIAN_POINT ( 'NONE',  ( 5.420364854932000931, 15.49051278174644075, 25.07142857142857650 ) ) ;
#1088=CARTESIAN_POINT ( 'NONE',  ( -15.88516839912898071, -1.917699372586004980, 37.13881657323070584 ) ) ;
#1090=CARTESIAN_POINT ( 'NONE',  ( -1.607813917173034124, 14.26974319298267346, 6.642857142857143238 ) ) ;
#1093=CARTESIAN_POINT ( 'NONE',  ( 4.619798703721856192, 13.59724543428036725, 33.06738800180213644 ) ) ;
#1096=CARTESIAN_POINT ( 'NONE',  ( 13.89774397934249706, 1.693770420379375308, 34.13881657323070584 ) ) ;
#1100=CARTESIAN_POINT ( 'NONE',  ( -9.809645194534070356, 9.989344678689256796, 22.00404056962643651 ) ) ;
#1102=CARTESIAN_POINT ( 'NONE',  ( -9.809645194534070356, 9.989344678689256796, 28.00404056962643651 ) ) ;
#1104=CARTESIAN_POINT ( 'NONE',  ( -13.96533075980324234, 8.621071003556515677, 43.78167371608784464 ) ) ;
#1105=CARTESIAN_POINT ( 'NONE',  ( -0.9960085134059654122, 15.98222653422240747, 48.73000000000000398 ) ) ;
#1106=CARTESIAN_POINT ( 'NONE',  ( 13.54758718765249803, 8.512513224245457977, 19.71428571428571175 ) ) ;
#1107=CARTESIAN_POINT ( 'NONE',  ( 11.51250119794888249, 11.69682198916847682, 9.495959430373563492 ) ) ;
#1113=CARTESIAN_POINT ( 'NONE',  ( -1.607813917173034124, 14.26974319298267524, 36.64285714285714590 ) ) ;
#1115=CARTESIAN_POINT ( 'NONE',  ( 13.21436662431716869, -4.623906867372263640, 38.57142857142857650 ) ) ;
#1117=CARTESIAN_POINT ( 'NONE',  ( 11.31370849898469899, 11.31370849898481978, 49.50000000000000711 ) ) ;
#1119=CARTESIAN_POINT ( 'NONE',  ( -5.420364854931999155, -15.49051278174644253, 10.07142857142856940 ) ) ;
#1124=CARTESIAN_POINT ( 'NONE',  ( 8.731428362939190890, -13.89598863503036164, 27.21428571428572241 ) ) ;
#1125=CARTESIAN_POINT ( 'NONE',  ( -8.621071003556675549, 13.96533075980314642, 10.21832628391215358 ) ) ;
#1126=CARTESIAN_POINT ( 'NONE',  ( -14.26974319298268767, 1.607813917172874918, 29.35714285714285765 ) ) ;
#1130=CARTESIAN_POINT ( 'NONE',  ( 11.85413878919593422, 7.448449071214774619, 19.71428571428571175 ) ) ;
#1132=PRODUCT_DEFINITION_FORMATION_WITH_SPECIFIED_SOURCE ( 'ANY', '', #9151, .NOT_KNOWN. ) ;
#1133=CARTESIAN_POINT ( 'NONE',  ( -13.54758718765249625, -8.512513224245459753, 34.71428571428571530 ) ) ;
#1134=CARTESIAN_POINT ( 'NONE',  ( -1.967016585148659846, 16.29368510291087091, 44.63881657323071295 ) ) ;
#1136=CARTESIAN_POINT ( 'NONE',  ( -7.639999817571786700, 12.15899005565156266, 12.21428571428571708 ) ) ;
#1138=CARTESIAN_POINT ( 'NONE',  ( -12.22833218042443271, 7.529642458189139909, 25.78167371608785530 ) ) ;
#1140=CARTESIAN_POINT ( 'NONE',  ( 6.188763155949558836, 12.71101015088858510, 48.72999999999996135 ) ) ;
#1141=CARTESIAN_POINT ( 'NONE',  ( 13.89774397934249706, 1.693770420379375308, 40.13881657323070584 ) ) ;
#1145=CARTESIAN_POINT ( 'NONE',  ( 9.809645194534072132, -9.989344678689256796, 13.00404056962644006 ) ) ;
#1148=CARTESIAN_POINT ( 'NONE',  ( 5.297344310588354865, 15.53355953199867301, 39.06738800180213644 ) ) ;
#1149=CARTESIAN_POINT ( 'NONE',  ( -7.316011149999984475, 12.10800216009354813, 48.73000000000000398 ) ) ;
#1150=CARTESIAN_POINT ( 'NONE',  ( -1.791431617652833763, -15.89939535829188877, 21.85714285714286120 ) ) ;
#1151=CARTESIAN_POINT ( 'NONE',  ( 11.40355824106246985, -11.22385875690704538, 10.99595943037356882 ) ) ;
#1157=CARTESIAN_POINT ( 'NONE',  ( -7.639999817571787588, 12.15899005565156266, 36.21428571428573662 ) ) ;
#1158=CARTESIAN_POINT ( 'NONE',  ( 1.567502665446232957, 13.91197093850540156, 42.85714285714285410 ) ) ;
#1161=CARTESIAN_POINT ( 'NONE',  ( 5.420364854932001819, 15.49051278174644430, 43.07142857142858361 ) ) ;
#1164=CARTESIAN_POINT ( 'NONE',  ( 11.31370849898482334, -11.31370849898469366, 15.00000000000000000 ) ) ;
#1168=CARTESIAN_POINT ( 'NONE',  ( -13.82664651025767100, 8.841785722321537477, 3.789754855340718542 ) ) ;
#1170=CARTESIAN_POINT ( 'NONE',  ( -8.731428362939189114, 13.89598863503036341, 30.21428571428572596 ) ) ;
#1173=CARTESIAN_POINT ( 'NONE',  ( -1.707986654103994528, 16.32287076676380266, 4.646897712483579745 ) ) ;
#1174=CARTESIAN_POINT ( 'NONE',  ( 10.15407889436379030, 10.15407889436390576, 25.50000000000000711 ) ) ;
#1176=CARTESIAN_POINT ( 'NONE',  ( 15.89939535829187278, 1.791431617653015174, 2.142857142857140573 ) ) ;
#1179=CARTESIAN_POINT ( 'NONE',  ( 14.26974319298268767, -1.607813917172876916, 20.35714285714286476 ) ) ;
#1181=CARTESIAN_POINT ( 'NONE',  ( -8.731428362939187338, 13.89598863503036164, 36.21428571428572951 ) ) ;
#1182=CARTESIAN_POINT ( 'NONE',  ( -8.404922754268618235, -13.61519076058357491, 48.28167371608785174 ) ) ;
#1184=CARTESIAN_POINT ( 'NONE',  ( -9.899494936611716867, 9.899494936611610285, 5.999999999999998224 ) ) ;
#1186=CARTESIAN_POINT ( 'NONE',  ( 7.340858601237956194, 11.92174236212700045, 21.28167371608785530 ) ) ;
#1190=CARTESIAN_POINT ( 'NONE',  ( 14.26974319298268767, -1.607813917172876916, 2.357142857142856762 ) ) ;
#1194=CARTESIAN_POINT ( 'NONE',  ( 10.24623928997352884, 10.06191849875416899, 35.50404056962644006 ) ) ;
#1195=CARTESIAN_POINT ( 'NONE',  ( 1.693770420379222319, 13.89774397934251837, 28.86118342676929416 ) ) ;
#1197=CARTESIAN_POINT ( 'NONE',  ( 16.32287076676382043, -1.707986654103810897, 34.35310228751642825 ) ) ;
#1199=CARTESIAN_POINT ( 'NONE',  ( -2.956870951528623337, 13.71658267976582835, 48.73000000000004661 ) ) ;
#1200=CARTESIAN_POINT ( 'NONE',  ( -5.284464991282755264, 15.10213328493384743, 24.42857142857143060 ) ) ;
#1202=CARTESIAN_POINT ( 'NONE',  ( 4.743843029824831525, -13.17239914596749095, 17.42453085894499409 ) ) ;
#1207=CARTESIAN_POINT ( 'NONE',  ( 11.85413878919593422, 7.448449071214774619, 25.71428571428571885 ) ) ;
#1208=CARTESIAN_POINT ( 'NONE',  ( 1.607813917173038121, -14.26974319298267346, 33.64285714285715301 ) ) ;
#1209=ORIENTED_EDGE ( 'NONE', *, *, #6503, .T. ) ;
#1210=CARTESIAN_POINT ( 'NONE',  ( -15.89939535829186923, -1.791431617653016062, 41.14285714285714590 ) ) ;
#1212=CARTESIAN_POINT ( 'NONE',  ( 15.49051278174638036, 5.420364854932175014, 19.92857142857143771 ) ) ;
#1221=CARTESIAN_POINT ( 'NONE',  ( 13.61519076058348254, 8.404922754268771001, 5.718326283912152697 ) ) ;
#1222=CARTESIAN_POINT ( 'NONE',  ( -15.10213328493390961, 5.284464991282586510, 23.57142857142857650 ) ) ;
#1225=CARTESIAN_POINT ( 'NONE',  ( 15.06016580658428694, -5.404401153735007846, 12.57546914105500768 ) ) ;
#1226=CARTESIAN_POINT ( 'NONE',  ( -13.21436662431716869, 4.623906867372262752, 23.57142857142857650 ) ) ;
#1227=CARTESIAN_POINT ( 'NONE',  ( -15.49051278174638036, -5.420364854932175902, 4.928571428571430602 ) ) ;
#1228=CARTESIAN_POINT ( 'NONE',  ( -1.791431617652833763, -15.89939535829188877, 39.85714285714286120 ) ) ;
#1230=CARTESIAN_POINT ( 'NONE',  ( 10.15407889436379030, 10.15407889436390576, 13.50000000000000178 ) ) ;
#1231=CARTESIAN_POINT ( 'NONE',  ( -15.89939535829186923, -1.791431617653016062, 35.14285714285713880 ) ) ;
#1232=CARTESIAN_POINT ( 'NONE',  ( 9.989344678689365153, -9.809645194533958446, 4.995959430373563492 ) ) ;
#1234=CARTESIAN_POINT ( 'NONE',  ( 1.567502665446232957, 13.91197093850540156, 12.85714285714285943 ) ) ;
#1235=ADVANCED_FACE ( 'NONE', ( #3964 ), #2048, .T. ) ;
#1236=CARTESIAN_POINT ( 'NONE',  ( -14.28433602490915000, 1.478298951650542481, 25.35310228751642470 ) ) ;
#1240=CARTESIAN_POINT ( 'NONE',  ( -4.743843029824828861, 13.17239914596749450, 50.42453085894499765 ) ) ;
#1244=CARTESIAN_POINT ( 'NONE',  ( -12.08964793087886314, 7.750357176954159932, 27.78975485534072121 ) ) ;
#1246=CARTESIAN_POINT ( 'NONE',  ( -5.404401153735176599, 15.06016580658422477, 44.42453085894499765 ) ) ;
#1249=CARTESIAN_POINT ( 'NONE',  ( -1.441234910513241818, -13.92619789766829008, 11.85310228751642470 ) ) ;
#1253=CARTESIAN_POINT ( 'NONE',  ( -9.809645194534070356, 9.989344678689256796, -1.995959430373561272 ) ) ;
#1254=CARTESIAN_POINT ( 'NONE',  ( 13.55419868402807992, 4.742819248065648807, 37.92857142857143060 ) ) ;
#1256=CARTESIAN_POINT ( 'NONE',  ( 10.03895970123120307, 12.58845729673829972, 49.39149694378009769 ) ) ;
#1257=CARTESIAN_POINT ( 'NONE',  ( -5.232950123192864567, 15.02148939460208332, -1.389475189636305469E-15 ) ) ;
#1258=CARTESIAN_POINT ( 'NONE',  ( -1.791431617652833763, -15.89939535829188877, 27.85714285714285765 ) ) ;
#1266=CARTESIAN_POINT ( 'NONE',  ( 5.543385399275644332, 15.44746603149420494, 5.075469141055008571 ) ) ;
#1267=CARTESIAN_POINT ( 'NONE',  ( 8.731428362939190890, -13.89598863503036164, 39.21428571428571530 ) ) ;
#1269=CARTESIAN_POINT ( 'NONE',  ( 8.621071003556677326, -13.96533075980314287, 1.218326283912148922 ) ) ;
#1270=CARTESIAN_POINT ( 'NONE',  ( -4.742819248065502258, -13.55419868402813677, 28.07142857142857295 ) ) ;
#1271=CARTESIAN_POINT ( 'NONE',  ( -15.89939535829186923, -1.791431617653016062, 5.142857142857143238 ) ) ;
#1272=CARTESIAN_POINT ( 'NONE',  ( -13.54758718765249625, -8.512513224245459753, 46.71428571428571530 ) ) ;
#1278=CARTESIAN_POINT ( 'NONE',  ( 1.791431617652837316, 15.89939535829188877, 30.85714285714286120 ) ) ;
#1280=CARTESIAN_POINT ( 'NONE',  ( -4.619798703721853528, -13.59724543428036725, 6.067388001802139996 ) ) ;
#1283=CARTESIAN_POINT ( 'NONE',  ( 10.15407889436379030, 10.15407889436390221, 31.50000000000000711 ) ) ;
#1284=CARTESIAN_POINT ( 'NONE',  ( -13.25633410266679313, 4.503970704919840529, 37.56738800180213644 ) ) ;
#1286=ORIENTED_EDGE ( 'NONE', *, *, #4236, .T. ) ;
#1290=CARTESIAN_POINT ( 'NONE',  ( 13.89774397934249706, 1.693770420379375308, 46.13881657323070584 ) ) ;
#1295=CARTESIAN_POINT ( 'NONE',  ( -9.809645194534070356, 9.989344678689256796, 28.00404056962643651 ) ) ;
#1299=CARTESIAN_POINT ( 'NONE',  ( 8.404922754268618235, 13.61519076058357491, 33.28167371608784464 ) ) ;
#1301=CARTESIAN_POINT ( 'NONE',  ( -13.05196022747598050, 7.990434241189387166, 48.73000000000000398 ) ) ;
#1303=CARTESIAN_POINT ( 'NONE',  ( -7.340858601237953529, -11.92174236212700222, 18.28167371608785174 ) ) ;
#1307=CARTESIAN_POINT ( 'NONE',  ( 7.639999817571789364, -12.15899005565156266, 45.21428571428572951 ) ) ;
#1308=CARTESIAN_POINT ( 'NONE',  ( 7.556039541191335474, 11.78653521626503320, -0.7102451446592792372 ) ) ;
#1310=CARTESIAN_POINT ( 'NONE',  ( 15.89939535829187278, 1.791431617653015174, 44.14285714285714590 ) ) ;
#1312=CARTESIAN_POINT ( 'NONE',  ( -10.35053069349207178, 12.21555809740962495, 4.615094676506451939E-15 ) ) ;
#1313=CARTESIAN_POINT ( 'NONE',  ( 11.31370849898482334, -11.31370849898469366, 27.00000000000000355 ) ) ;
#1321=CARTESIAN_POINT ( 'NONE',  ( -1.791431617652833763, -15.89939535829188877, 45.85714285714286120 ) ) ;
#1322=CARTESIAN_POINT ( 'NONE',  ( 1.707986654103998303, -16.32287076676380266, 25.64689771248357886 ) ) ;
#1324=CARTESIAN_POINT ( 'NONE',  ( 11.85413878919593422, 7.448449071214774619, 19.71428571428571175 ) ) ;
#1325=CARTESIAN_POINT ( 'NONE',  ( 16.30827793483735633, -1.837501619626142890, 2.357142857142856762 ) ) ;
#1326=CARTESIAN_POINT ( 'NONE',  ( 13.54758718765249803, 8.512513224245457977, 43.71428571428572241 ) ) ;
#1327=ORIENTED_EDGE ( 'NONE', *, *, #2410, .F. ) ;
#1334=CARTESIAN_POINT ( 'NONE',  ( -13.25633410266679313, 4.503970704919840529, 7.567388001802139108 ) ) ;
#1336=CARTESIAN_POINT ( 'NONE',  ( -15.10213328493390961, 5.284464991282586510, 5.571428571428574728 ) ) ;
#1337=CARTESIAN_POINT ( 'NONE',  ( 15.89939535829187278, 1.791431617653015174, 8.142857142857145902 ) ) ;
#1339=CARTESIAN_POINT ( 'NONE',  ( -13.91197093850538380, -1.567502665446387278, 29.14285714285714235 ) ) ;
#1344=CARTESIAN_POINT ( 'NONE',  ( -14.28433602490915000, 1.478298951650542481, 37.35310228751641404 ) ) ;
#1347=CARTESIAN_POINT ( 'NONE',  ( 15.14410076328353227, -5.164528828830166063, 28.56738800180213644 ) ) ;
#1349=CARTESIAN_POINT ( 'NONE',  ( 4.743843029824831525, -13.17239914596749095, 47.42453085894499765 ) ) ;
#1354=CARTESIAN_POINT ( 'NONE',  ( -13.17239914596754424, 4.743843029824683200, 27.57546914105500946 ) ) ;
#1356=CARTESIAN_POINT ( 'NONE',  ( 12.22833218042443271, -7.529642458189144349, 4.781673716087850856 ) ) ;
#1361=CARTESIAN_POINT ( 'NONE',  ( 7.750357176954296712, -12.08964793087877787, 23.21024514465928235 ) ) ;
#1365=CARTESIAN_POINT ( 'NONE',  ( -1.607813917173034124, 14.26974319298267524, 42.64285714285715301 ) ) ;
#1367=CARTESIAN_POINT ( 'NONE',  ( 9.809645194534072132, -9.989344678689256796, 1.004040569626440726 ) ) ;
#1369=CARTESIAN_POINT ( 'NONE',  ( 8.841785722321695573, -13.82664651025757152, 5.210245144659280569 ) ) ;
#1372=CARTESIAN_POINT ( 'NONE',  ( 1.837501619626330074, -16.30827793483733501, 33.64285714285715301 ) ) ;
#1373=DIRECTION ( 'NONE',  ( -1.000000000000000000, 0.000000000000000000, 0.000000000000000000 ) ) ;
#1375=( BOUNDED_CURVE ( )  B_SPLINE_CURVE ( 2, ( #9572, #5575, #8738, #7185, #7232, #101, #8849, #1658, #3254, #4860, #937, #5680, #9523, #8642, #1759, #4910, #1562, #986, #3361, #6496, #4708, #7857, #3557, #9775, #3510, #4386, #1860, #7537, #1184, #5058, #7486, #1090, #4334, #412, #5010, #260, #5824, #464, #5921, #4281, #5106, #3407, #6685, #2677, #7336, #7433, #309, #3603, #9047, #8204, #9870, #362, #9097, #5773, #4187, #2775, #8157, #1136, #6735, #6640, #1234, #1042, #2010, #8947, #9000, #2583, #1807, #6543, #4231, #9722, #5726, #6591, #7382, #3449, #8894, #5164, #2626, #1910, #9824, #2726, #5869, #1958, #8258, #8316, #4961, #8113, #2265, #7702, #2932, #6074, #9355, #5412, #4551, #8522, #10069, #4441, #1396, #7648, #2059, #621, #9973, #9202, #9305, #9250, #8412, #3870, #8471, #2985, #567, #3713, #2830, #3768, #2112, #5255, #2880, #7587, #2219, #6959, #1494, #1446, #6178, #4596, #6902, #6130, #10121, #5365, #6022, #5212, #7749, #8571, #670, #3823, #6797, #2170, #9152, #6849, #1339, #4647, #4493, #10019, #3038, #8362, #9925, #5313, #5974, #7801, #723, #1283, #513, #3659, #768, #4696, #1747, #1549, #4845, #2464, #9462, #10224, #2365, #87, #7169, #6279, #138, #6229, #3195, #5517, #7946, #874, #7121, #38, #9511, #5614, #2417, #3290, #6331, #3134, #3972, #4071, #9615, #5666, #5466, #8677, #1597, #3242, #6380, #7892, #4747, #923, #817, #5563, #9559, #8725, #1646, #4896, #6432, #4026, #2517, #8834, #4793, #7995, #8782, #1700, #7219, #8044, #973, #7013, #10171, #3085, #9405, #7843, #8628, #2316, #3916, #7061, #2760, #3348, #8097, #7322, #1025, #5909, #8144, #9034, #2614, #2713, #1945, #6529, #1794, #7370, #1998 ),
 .UNSPECIFIED., .F., .F. ) 
 B_SPLINE_CURVE_WITH_KNOTS ( ( 3, 2, 2, 2, 2, 2, 2, 2, 2, 2, 2, 2, 2, 2, 2, 2, 2, 2, 2, 2, 2, 2, 2, 2, 2, 2, 2, 2, 2, 2, 2, 2, 2, 2, 2, 2, 2, 2, 2, 2, 2, 2, 2, 2, 2, 2, 2, 2, 2, 2, 2, 2, 2, 2, 2, 2, 2, 2, 2, 2, 2, 2, 2, 2, 2, 2, 2, 2, 2, 2, 2, 2, 2, 2, 2, 2, 2, 2, 2, 2, 2, 2, 2, 2, 2, 2, 2, 2, 2, 2, 2, 2, 2, 2, 2, 2, 2, 2, 2, 2, 2, 2, 2, 2, 2, 2, 2, 2, 2, 2, 2, 2, 2, 2, 3 ),
 ( 0.000000000000000000, 0.007936507936507936067, 0.01587301587301587213, 0.02380952380952380820, 0.03174603174603174427, 0.03968253968253968034, 0.04761904761904761640, 0.05555555555555555247, 0.06349206349206348854, 0.07142857142857142461, 0.07936507936507936067, 0.08730158730158729674, 0.09523809523809523281, 0.1031746031746031689, 0.1111111111111111049, 0.1190476190476190410, 0.1269841269841269771, 0.1349206349206349131, 0.1428571428571428492, 0.1507936507936508130, 0.1587301587301587213, 0.1666666666666666574, 0.1746031746031745935, 0.1825396825396825295, 0.1904761904761904656, 0.1984126984126984017, 0.2063492063492063378, 0.2142857142857142738, 0.2222222222222222099, 0.2301587301587301460, 0.2380952380952380820, 0.2460317460317460181, 0.2539682539682539542, 0.2619047619047619180, 0.2698412698412698263, 0.2777777777777777901, 0.2857142857142856984, 0.2936507936507936622, 0.3015873015873016261, 0.3095238095238095344, 0.3174603174603174427, 0.3253968253968254065, 0.3333333333333333148, 0.3412698412698412787, 0.3492063492063491870, 0.3571428571428571508, 0.3650793650793650591, 0.3730158730158730229, 0.3809523809523809312, 0.3888888888888889506, 0.3968253968253968034, 0.4047619047619047117, 0.4126984126984126755, 0.4206349206349206393, 0.4285714285714285476, 0.4365079365079365115, 0.4444444444444444198, 0.4523809523809523836, 0.4603174603174602919, 0.4682539682539682557, 0.4761904761904761640, 0.4841269841269841279, 0.4920634920634920362, 0.5000000000000000000, 0.5079365079365079083, 0.5158730158730159276, 0.5238095238095238360, 0.5317460317460317443, 0.5396825396825396526, 0.5476190476190476719, 0.5555555555555555802, 0.5634920634920634885, 0.5714285714285713969, 0.5793650793650794162, 0.5873015873015873245, 0.5952380952380952328, 0.6031746031746032521, 0.6111111111111111605, 0.6190476190476190688, 0.6269841269841269771, 0.6349206349206348854, 0.6428571428571429047, 0.6507936507936508130, 0.6587301587301587213, 0.6666666666666666297, 0.6746031746031747600, 0.6825396825396825573, 0.6904761904761904656, 0.6984126984126983739, 0.7063492063492063933, 0.7142857142857143016, 0.7222222222222222099, 0.7301587301587301182, 0.7380952380952381375, 0.7460317460317460458, 0.7539682539682539542, 0.7619047619047618625, 0.7698412698412698818, 0.7777777777777779011, 0.7857142857142856984, 0.7936507936507936067, 0.8015873015873016261, 0.8095238095238094234, 0.8174603174603174427, 0.8253968253968253510, 0.8333333333333333703, 0.8412698412698412787, 0.8492063492063491870, 0.8571428571428570953, 0.8650793650793651146, 0.8730158730158730229, 0.8809523809523809312, 0.8888888888888888395, 0.8968253968253968589, 0.9023904529665215390 ),
 .UNSPECIFIED. ) 
 CURVE ( )  GEOMETRIC_REPRESENTATION_ITEM ( )  RATIONAL_B_SPLINE_CURVE ( ( 1.000000000000000000, 0.9749279121818236193, 1.000000000000000000, 0.9749279121818236193, 1.000000000000000000, 0.9749279121818236193, 1.000000000000000000, 0.9749279121818236193, 1.000000000000000000, 0.9749279121818236193, 1.000000000000000000, 0.9749279121818236193, 1.000000000000000000, 0.9749279121818236193, 1.000000000000000000, 0.9749279121818236193, 1.000000000000000000, 0.9749279121818236193, 1.000000000000000000, 0.9749279121818236193, 1.000000000000000000, 0.9749279121818236193, 1.000000000000000000, 0.9749279121818236193, 1.000000000000000000, 0.9749279121818236193, 1.000000000000000000, 0.9749279121818236193, 1.000000000000000000, 0.9749279121818236193, 1.000000000000000000, 0.9749279121818236193, 1.000000000000000000, 0.9749279121818236193, 1.000000000000000000, 0.9749279121818236193, 1.000000000000000000, 0.9749279121818236193, 1.000000000000000000, 0.9749279121818236193, 1.000000000000000000, 0.9749279121818236193, 1.000000000000000000, 0.9749279121818236193, 1.000000000000000000, 0.9749279121818236193, 1.000000000000000000, 0.9749279121818236193, 1.000000000000000000, 0.9749279121818236193, 1.000000000000000000, 0.9749279121818236193, 1.000000000000000000, 0.9749279121818236193, 1.000000000000000000, 0.9749279121818236193, 1.000000000000000000, 0.9749279121818236193, 1.000000000000000000, 0.9749279121818236193, 1.000000000000000000, 0.9749279121818236193, 1.000000000000000000, 0.9749279121818236193, 1.000000000000000000, 0.9749279121818236193, 1.000000000000000000, 0.9749279121818236193, 1.000000000000000000, 0.9749279121818236193, 1.000000000000000000, 0.9749279121818236193, 1.000000000000000000, 0.9749279121818236193, 1.000000000000000000, 0.9749279121818236193, 1.000000000000000000, 0.9749279121818236193, 1.000000000000000000, 0.9749279121818236193, 1.000000000000000000, 0.9749279121818236193, 1.000000000000000000, 0.9749279121818236193, 1.000000000000000000, 0.9749279121818236193, 1.000000000000000000, 0.9749279121818236193, 1.000000000000000000, 0.9749279121818236193, 1.000000000000000000, 0.9749279121818236193, 1.000000000000000000, 0.9749279121818236193, 1.000000000000000000, 0.9749279121818236193, 1.000000000000000000, 0.9749279121818236193, 1.000000000000000000, 0.9749279121818236193, 1.000000000000000000, 0.9749279121818236193, 1.000000000000000000, 0.9749279121818236193, 1.000000000000000000, 0.9749279121818236193, 1.000000000000000000, 0.9749279121818236193, 1.000000000000000000, 0.9749279121818236193, 1.000000000000000000, 0.9749279121818236193, 1.000000000000000000, 0.9749279121818236193, 1.000000000000000000, 0.9749279121818236193, 1.000000000000000000, 0.9749279121818236193, 1.000000000000000000, 0.9749279121818236193, 1.000000000000000000, 0.9749279121818236193, 1.000000000000000000, 0.9749279121818236193, 1.000000000000000000, 0.9749279121818236193, 1.000000000000000000, 0.9749279121818236193, 1.000000000000000000, 0.9749279121818236193, 1.000000000000000000, 0.9749279121818236193, 1.000000000000000000, 0.9749279121818236193, 1.000000000000000000, 0.9749279121818236193, 1.000000000000000000, 0.9749279121818236193, 1.000000000000000000, 0.9749279121818236193, 1.000000000000000000, 0.9749279121818236193, 1.000000000000000000, 0.9749279121818236193, 1.000000000000000000, 0.9749279121818236193, 1.000000000000000000, 0.9749279121818236193, 1.000000000000000000, 0.9749279121818236193, 1.000000000000000000, 0.9749279121818236193, 1.000000000000000000, 0.9749279121818236193, 1.000000000000000000, 0.9749279121818236193, 1.000000000000000000, 0.9749279121818236193, 1.000000000000000000, 0.9749279121818236193, 1.000000000000000000, 0.9749279121818236193, 1.000000000000000000, 0.9749279121818236193, 1.000000000000000000, 0.9749279121818236193, 1.000000000000000000, 0.9749279121818236193, 1.000000000000000000, 0.9749279121818236193, 1.000000000000000000, 0.9749279121818236193, 1.000000000000000000, 0.9749279121818236193, 1.000000000000000000, 0.9749279121818236193, 1.000000000000000000, 0.9749279121818236193, 1.000000000000000000, 0.9749279121818236193, 1.000000000000000000, 0.9749279121818236193, 1.000000000000000000, 0.9749279121818236193, 1.000000000000000000, 0.9749279121818236193, 1.000000000000000000, 0.9749279121818236193, 1.000000000000000000, 0.9749279121818236193, 1.000000000000000000, 0.9749279121818236193, 1.000000000000000000, 0.9749279121818236193, 1.000000000000000000, 0.9749279121818236193, 1.000000000000000000, 0.9749279121818236193, 1.000000000000000000, 0.9749279121818236193, 1.000000000000000000, 0.9749279121818236193, 1.000000000000000000, 0.9749279121818236193, 1.000000000000000000, 0.9749279121818236193, 1.000000000000000000, 0.9749279121818236193, 1.000000000000000000, 0.9749279121818236193, 1.000000000000000000, 0.9749279121818236193, 1.000000000000000000, 0.9749279121818236193, 1.000000000000000000, 0.9749279121818236193, 1.000000000000000000, 0.9749279121818236193, 1.000000000000000000, 0.9749279121818236193, 1.000000000000000000, 0.9749279121818236193, 1.000000000000000000, 0.9749279121818236193, 1.000000000000000000, 0.9749279121818236193, 1.000000000000000000, 0.9824195253882965773, 0.9894938054834332419 ) ) 
 REPRESENTATION_ITEM ( '' )  );
#1380=CARTESIAN_POINT ( 'NONE',  ( 11.22385875690717683, -11.40355824106234373, 19.00404056962642940 ) ) ;
#1381=CARTESIAN_POINT ( 'NONE',  ( 13.54758718765249803, 8.512513224245457977, 43.71428571428572241 ) ) ;
#1382=CARTESIAN_POINT ( 'NONE',  ( 8.620103694221997515, 13.47998361472160767, 17.28975485534072121 ) ) ;
#1383=CARTESIAN_POINT ( 'NONE',  ( 4.742819248065503146, 13.55419868402813677, 31.07142857142857295 ) ) ;
#1384=CARTESIAN_POINT ( 'NONE',  ( -5.420364854931999155, -15.49051278174644253, 16.07142857142857650 ) ) ;
#1385=CARTESIAN_POINT ( 'NONE',  ( -8.512513224245306986, -13.54758718765259218, 46.28571428571429180 ) ) ;
#1389=CARTESIAN_POINT ( 'NONE',  ( 5.284464991282756152, -15.10213328493384743, 45.42857142857143060 ) ) ;
#1391=CARTESIAN_POINT ( 'NONE',  ( -1.737328882695368115, 14.25515036105620581, 8.638816573230704066 ) ) ;
#1393=CARTESIAN_POINT ( 'NONE',  ( -11.31370849898482156, 11.31370849898469544, 0.000000000000000000 ) ) ;
#1394=CARTESIAN_POINT ( 'NONE',  ( 16.30827793483735633, -1.837501619626142890, 2.357142857142856762 ) ) ;
#1396=CARTESIAN_POINT ( 'NONE',  ( 13.21436662431716869, -4.623906867372263640, 20.57142857142857295 ) ) ;
#1398=CARTESIAN_POINT ( 'NONE',  ( 9.989344678689365153, -9.809645194533958446, 46.99595943037356705 ) ) ;
#1402=CARTESIAN_POINT ( 'NONE',  ( -1.665163862719845067, -15.91362231745477374, 17.85310228751642114 ) ) ;
#1403=CARTESIAN_POINT ( 'NONE',  ( -5.284464991282755264, 15.10213328493384743, 0.4285714285714309346 ) ) ;
#1405=CARTESIAN_POINT ( 'NONE',  ( 9.989344678689365153, -9.809645194533958446, 46.99595943037356705 ) ) ;
#1409=CARTESIAN_POINT ( 'NONE',  ( -7.529642458189277576, 12.22833218042435455, 28.21832628391215181 ) ) ;
#1411=CARTESIAN_POINT ( 'NONE',  ( -1.441234910513241818, -13.92619789766829008, 5.853102287516418478 ) ) ;
#1412=B_SPLINE_CURVE_WITH_KNOTS ( 'NONE', 3,
 ( #2256, #5357, #8715, #3863, #80, #9297, #2408, #7003, #762, #6949, #2211, #7055, #6170, #6122, #10216, #6321 ),
 .UNSPECIFIED., .F., .F.,
 ( 4, 2, 2, 2, 2, 2, 2, 4 ),
 ( 0.04369022279437502487, 0.04534324305125501248, 0.04699626330813499314, 0.05030230382189496835, 0.05195532407877494901, 0.05360834433565493662, 0.05526136459253491728, 0.05691438484941489795 ),
 .UNSPECIFIED. ) ;
#1415=CARTESIAN_POINT ( 'NONE',  ( 11.31370849898482334, -11.31370849898469366, 27.00000000000000355 ) ) ;
#1417=CARTESIAN_POINT ( 'NONE',  ( 10.06191849875406064, 10.24623928997363187, 15.49595943037356882 ) ) ;
#1421=CARTESIAN_POINT ( 'NONE',  ( 10.15407889436379030, 10.15407889436390576, 43.50000000000000711 ) ) ;
#1422=CARTESIAN_POINT ( 'NONE',  ( -4.865839792409144771, -13.51115193377589740, 2.075469141055009015 ) ) ;
#1424=CARTESIAN_POINT ( 'NONE',  ( -5.297344310588352201, -15.53355953199867301, 12.06738800180214000 ) ) ;
#1426=CARTESIAN_POINT ( 'NONE',  ( 1.837501619626330074, -16.30827793483733501, 27.64285714285714590 ) ) ;
#1432=CARTESIAN_POINT ( 'NONE',  ( -5.420364854931999155, -15.49051278174644253, 46.07142857142856940 ) ) ;
#1434=CARTESIAN_POINT ( 'NONE',  ( 15.53355953199861794, 5.297344310588528060, 23.93261199819786711 ) ) ;
#1439=CARTESIAN_POINT ( 'NONE',  ( 15.10213328493390783, -5.284464991282587398, 44.57142857142857650 ) ) ;
#1440=( NAMED_UNIT ( * ) SI_UNIT ( $, .STERADIAN. ) SOLID_ANGLE_UNIT ( ) );
#1443=CARTESIAN_POINT ( 'NONE',  ( 1.837501619626330074, -16.30827793483733501, 3.642857142857144126 ) ) ;
#1444=CARTESIAN_POINT ( 'NONE',  ( -1.917699372585823570, -15.88516839912900558, 43.86118342676930126 ) ) ;
#1446=CARTESIAN_POINT ( 'NONE',  ( 10.15407889436379030, 10.15407889436390221, 25.50000000000000355 ) ) ;
#1447=CARTESIAN_POINT ( 'NONE',  ( 4.503970704919991519, -13.25633410266674517, 31.43261199819787421 ) ) ;
#1450=CARTESIAN_POINT ( 'NONE',  ( 9.989344678689365153, -9.809645194533958446, 40.99595943037355994 ) ) ;
#1453=CARTESIAN_POINT ( 'NONE',  ( 11.40355824106246985, -11.22385875690704538, 22.99595943037356705 ) ) ;
#1456=CARTESIAN_POINT ( 'NONE',  ( -1.665163862719845067, -15.91362231745477374, 23.85310228751642825 ) ) ;
#1460=CARTESIAN_POINT ( 'NONE',  ( -14.25515036105622890, 1.737328882695209575, 45.36118342676930837 ) ) ;
#1462=CARTESIAN_POINT ( 'NONE',  ( -9.989344678689363377, 9.809645194533960222, 1.995959430373561272 ) ) ;
#1465=CARTESIAN_POINT ( 'NONE',  ( 4.743843029824831525, -13.17239914596749095, 29.42453085894499765 ) ) ;
#1469=CARTESIAN_POINT ( 'NONE',  ( -5.164528828830334817, 15.14410076328347543, 40.43261199819787066 ) ) ;
#1470=CARTESIAN_POINT ( 'NONE',  ( 1.607813917173038121, -14.26974319298267346, 39.64285714285716722 ) ) ;
#1471=CARTESIAN_POINT ( 'NONE',  ( -1.478298951650703019, 14.28433602490913579, 4.646897712483579745 ) ) ;
#1474=CARTESIAN_POINT ( 'NONE',  ( -15.14410076328353227, 5.164528828830164287, 13.56738800180213822 ) ) ;
#1477=CARTESIAN_POINT ( 'NONE',  ( 15.10213328493390783, -5.284464991282587398, 38.57142857142857650 ) ) ;
#1483=CARTESIAN_POINT ( 'NONE',  ( -15.89939535829186923, -1.791431617653016062, 41.14285714285714590 ) ) ;
#1484=CARTESIAN_POINT ( 'NONE',  ( -16.29368510291090288, 1.967016585148476215, 15.36118342676929771 ) ) ;
#1485=CARTESIAN_POINT ( 'NONE',  ( 15.49051278174638036, 5.420364854932175014, 19.92857142857143771 ) ) ;
#1488=CARTESIAN_POINT ( 'NONE',  ( -16.30827793483735988, 1.837501619626141558, 47.35714285714286120 ) ) ;
#1492=CARTESIAN_POINT ( 'NONE',  ( 5.164528828830335705, -15.14410076328347543, 43.43261199819787066 ) ) ;
#1494=CARTESIAN_POINT ( 'NONE',  ( 7.448449071214646722, 11.85413878919601594, 25.28571428571428470 ) ) ;
#1498=CARTESIAN_POINT ( 'NONE',  ( -7.750357176954294935, 12.08964793087877787, 38.21024514465928235 ) ) ;
#1501=CARTESIAN_POINT ( 'NONE',  ( -1.967016585148659846, 16.29368510291087091, 26.63881657323070939 ) ) ;
#1502=CARTESIAN_POINT ( 'NONE',  ( 13.89598863503045933, -8.731428362939032795, 2.785714285714283367 ) ) ;
#1503=CARTESIAN_POINT ( 'NONE',  ( 5.404401153735178376, -15.06016580658422477, 17.42453085894499409 ) ) ;
#1511=CARTESIAN_POINT ( 'NONE',  ( -1.737328882695368115, 14.25515036105620581, 8.638816573230704066 ) ) ;
#1515=CARTESIAN_POINT ( 'NONE',  ( 13.54758718765249803, 8.512513224245457977, 31.71428571428571530 ) ) ;
#1518=CARTESIAN_POINT ( 'NONE',  ( 7.340858601237956194, 11.92174236212700045, 27.28167371608785174 ) ) ;
#1522=CARTESIAN_POINT ( 'NONE',  ( 5.543385399275644332, 15.44746603149420494, 47.07546914105501656 ) ) ;
#1523=CARTESIAN_POINT ( 'NONE',  ( 10.24623928997352884, 10.06191849875416899, 5.504040569626439172 ) ) ;
#1524=CARTESIAN_POINT ( 'NONE',  ( -12.08964793087886314, 7.750357176954159932, 3.789754855340718542 ) ) ;
#1528=CARTESIAN_POINT ( 'NONE',  ( -8.512513224245306986, -13.54758718765259218, 40.28571428571428470 ) ) ;
#1533=CARTESIAN_POINT ( 'NONE',  ( -16.30827793483735988, 1.837501619626141780, 35.35714285714285410 ) ) ;
#1536=CARTESIAN_POINT ( 'NONE',  ( -5.543385399275643444, -15.44746603149420494, 20.07546914105500591 ) ) ;
#1538=CARTESIAN_POINT ( 'NONE',  ( -13.82664651025767100, 8.841785722321537477, 21.78975485534072476 ) ) ;
#1539=CARTESIAN_POINT ( 'NONE',  ( 11.60466159355862104, 11.60466159355875071, 19.50000000000000355 ) ) ;
#1543=CARTESIAN_POINT ( 'NONE',  ( 13.89598863503045933, -8.731428362939032795, 38.78571428571429180 ) ) ;
#1546=CARTESIAN_POINT ( 'NONE',  ( -8.512513224245306986, -13.54758718765259218, 4.285714285714288252 ) ) ;
#1547=CARTESIAN_POINT ( 'NONE',  ( -11.60466159355861926, -11.60466159355875249, 4.500000000000005329 ) ) ;
#1549=CARTESIAN_POINT ( 'NONE',  ( 12.15899005565164792, -7.639999817571654361, 32.78571428571429180 ) ) ;
#1550=CARTESIAN_POINT ( 'NONE',  ( -10.24623928997352351, -10.06191849875416899, 32.50404056962644006 ) ) ;
#1554=CARTESIAN_POINT ( 'NONE',  ( -4.742819248065502258, -13.55419868402813677, 4.071428571428569398 ) ) ;
#1557=CARTESIAN_POINT ( 'NONE',  ( -5.404401153735176599, 15.06016580658422477, 26.42453085894499765 ) ) ;
#1558=CARTESIAN_POINT ( 'NONE',  ( 13.54758718765249803, 8.512513224245457977, 1.714285714285716855 ) ) ;
#1559=CARTESIAN_POINT ( 'NONE',  ( -5.297344310588352201, -15.53355953199867301, 30.06738800180214355 ) ) ;
#1562=CARTESIAN_POINT ( 'NONE',  ( 4.623906867372411078, -13.21436662431711717, 3.428571428571426605 ) ) ;
#1564=CARTESIAN_POINT ( 'NONE',  ( 8.731428362939190890, -13.89598863503036164, 33.21428571428571530 ) ) ;
#1566=CARTESIAN_POINT ( 'NONE',  ( -11.40355824106246807, 11.22385875690704715, 49.99595943037357415 ) ) ;
#1568=CARTESIAN_POINT ( 'NONE',  ( 5.420364854932001819, 15.49051278174644430, 13.07142857142857295 ) ) ;
#1570=CARTESIAN_POINT ( 'NONE',  ( -4.743843029824828861, 13.17239914596749450, 26.42453085894499765 ) ) ;
#1574=CARTESIAN_POINT ( 'NONE',  ( 10.24623928997352884, 10.06191849875416899, -0.4959594303735606058 ) ) ;
#1575=CARTESIAN_POINT ( 'NONE',  ( 1.693770420379222319, 13.89774397934251837, 16.86118342676929061 ) ) ;
#1578=CARTESIAN_POINT ( 'NONE',  ( 8.512513224245308763, 13.54758718765259040, 37.28571428571429180 ) ) ;
#1583=CARTESIAN_POINT ( 'NONE',  ( -15.89939535829186923, -1.791431617653016062, 35.14285714285713880 ) ) ;
#1585=CARTESIAN_POINT ( 'NONE',  ( -13.61519076058348254, -8.404922754268771001, 32.71832628391215536 ) ) ;
#1587=CARTESIAN_POINT ( 'NONE',  ( 15.53355953199861794, 5.297344310588528060, 29.93261199819786356 ) ) ;
#1588=CARTESIAN_POINT ( 'NONE',  ( -13.54758718765249625, -8.512513224245459753, 16.71428571428571530 ) ) ;
#1590=CARTESIAN_POINT ( 'NONE',  ( 5.284464991282756152, -15.10213328493384743, 3.428571428571426605 ) ) ;
#1594=CARTESIAN_POINT ( 'NONE',  ( 10.24623928997352884, 10.06191849875416899, 41.50404056962644006 ) ) ;
#1595=CARTESIAN_POINT ( 'NONE',  ( 15.49051278174638036, 5.420364854932175014, 13.92857142857143238 ) ) ;
#1597=CARTESIAN_POINT ( 'NONE',  ( 9.899494936611718643, -9.899494936611608509, 39.00000000000000000 ) ) ;
#1599=CARTESIAN_POINT ( 'NONE',  ( -13.17239914596754424, 4.743843029824683200, 39.57546914105500946 ) ) ;
#1603=CARTESIAN_POINT ( 'NONE',  ( -1.567502665446231180, -13.91197093850540334, 9.857142857142855874 ) ) ;
#1605=CARTESIAN_POINT ( 'NONE',  ( -13.96533075980324234, 8.621071003556515677, 31.78167371608784819 ) ) ;
#1606=CARTESIAN_POINT ( 'NONE',  ( 16.30827793483735633, -1.837501619626142890, 20.35714285714285765 ) ) ;
#1607=CARTESIAN_POINT ( 'NONE',  ( 1.967016585148662289, -16.29368510291087091, 23.63881657323070939 ) ) ;
#1611=( LENGTH_UNIT ( ) NAMED_UNIT ( * ) SI_UNIT ( .MILLI., .METRE. ) );
#1612=CARTESIAN_POINT ( 'NONE',  ( 1.837501619626330074, -16.30827793483733501, 33.64285714285715301 ) ) ;
#1615=CARTESIAN_POINT ( 'NONE',  ( -8.512513224245306986, -13.54758718765259218, 10.28571428571428648 ) ) ;
#1617=CARTESIAN_POINT ( 'NONE',  ( -4.743843029824828861, 13.17239914596749450, 32.42453085894499054 ) ) ;
#1621=CARTESIAN_POINT ( 'NONE',  ( -11.92174236212692051, -7.340858601238089420, 2.718326283912150476 ) ) ;
#1625=CARTESIAN_POINT ( 'NONE',  ( 10.03895970123120307, 12.58845729673829972, 49.39149694378009769 ) ) ;
#1632=CARTESIAN_POINT ( 'NONE',  ( -15.06016580658428694, 5.404401153735006957, 27.57546914105500946 ) ) ;
#1634=CARTESIAN_POINT ( 'NONE',  ( -1.707986654103994528, 16.32287076676380266, 28.64689771248357886 ) ) ;
#1636=CARTESIAN_POINT ( 'NONE',  ( -5.284464991282755264, 15.10213328493384743, 30.42857142857143060 ) ) ;
#1638=CARTESIAN_POINT ( 'NONE',  ( -5.284464991282755264, 15.10213328493384743, 6.428571428571429713 ) ) ;
#1640=SURFACE_SIDE_STYLE ('',( #8718 ) ) ;
#1644=CARTESIAN_POINT ( 'NONE',  ( -1.917699372585823570, -15.88516839912900558, 1.861183426769295490 ) ) ;
#1645=CARTESIAN_POINT ( 'NONE',  ( -11.31370849898482156, 11.31370849898469544, 18.00000000000000355 ) ) ;
#1646=CARTESIAN_POINT ( 'NONE',  ( -13.91197093850538380, -1.567502665446387278, 41.14285714285714590 ) ) ;
#1647=CARTESIAN_POINT ( 'NONE',  ( -10.24623928997352351, -10.06191849875416899, 38.50404056962644006 ) ) ;
#1648=CARTESIAN_POINT ( 'NONE',  ( -4.503970704919988854, 13.25633410266674517, 34.43261199819786356 ) ) ;
#1652=CARTESIAN_POINT ( 'NONE',  ( 4.623906867372411078, -13.21436662431711717, 3.428571428571426605 ) ) ;
#1654=CARTESIAN_POINT ( 'NONE',  ( -11.31370849898482156, 11.31370849898469544, 11.99999999999999645 ) ) ;
#1655=CARTESIAN_POINT ( 'NONE',  ( -1.665163862719845067, -15.91362231745477374, 41.85310228751642825 ) ) ;
#1658=CARTESIAN_POINT ( 'NONE',  ( 10.15407889436379030, 10.15407889436390221, 1.500000000000003553 ) ) ;
#1659=ADVANCED_FACE ( 'NONE', ( #2101 ), #7385, .T. ) ;
#1664=CARTESIAN_POINT ( 'NONE',  ( 4.743843029824831525, -13.17239914596749095, 11.42453085894499587 ) ) ;
#1667=CARTESIAN_POINT ( 'NONE',  ( -1.441234910513241818, -13.92619789766829008, 23.85310228751642825 ) ) ;
#1674=CARTESIAN_POINT ( 'NONE',  ( 13.17239914596754424, -4.743843029824685864, 0.5754691410550027975 ) ) ;
#1675=CARTESIAN_POINT ( 'NONE',  ( -1.693770420379220099, -13.89774397934251837, 7.861183426769288829 ) ) ;
#1681=CARTESIAN_POINT ( 'NONE',  ( -16.30827793483735988, 1.837501619626141780, 41.35714285714286120 ) ) ;
#1688=CARTESIAN_POINT ( 'NONE',  ( 8.620103694221997515, 13.47998361472160767, 29.28975485534071765 ) ) ;
#1691=CARTESIAN_POINT ( 'NONE',  ( -5.164528828830334817, 15.14410076328347543, 40.43261199819787066 ) ) ;
#1693=CARTESIAN_POINT ( 'NONE',  ( 5.420364854932001819, 15.49051278174644430, 31.07142857142857295 ) ) ;
#1694=CARTESIAN_POINT ( 'NONE',  ( 3.926188687689436296, 14.48606370741319083, 1.336143574210037107E-16 ) ) ;
#1698=CARTESIAN_POINT ( 'NONE',  ( -15.53355953199861794, -5.297344310588530725, 2.932611998197868886 ) ) ;
#1699=CARTESIAN_POINT ( 'NONE',  ( -13.89598863503046111, 8.731428362939027465, 11.78571428571428115 ) ) ;
#1700=CARTESIAN_POINT ( 'NONE',  ( 4.742819248065502258, 13.55419868402813499, 43.07142857142857650 ) ) ;
#1701=CARTESIAN_POINT ( 'NONE',  ( -13.17239914596754424, 4.743843029824683200, 45.57546914105501656 ) ) ;
#1702=CARTESIAN_POINT ( 'NONE',  ( -10.15407889436378852, -10.15407889436390576, 4.500000000000005329 ) ) ;
#1706=CARTESIAN_POINT ( 'NONE',  ( 1.567502665446232957, 13.91197093850540156, 6.857142857142860315 ) ) ;
#1709=CARTESIAN_POINT ( 'NONE',  ( -15.49051278174637858, -5.420364854932175014, 10.92857142857143060 ) ) ;
#1711=CARTESIAN_POINT ( 'NONE',  ( -8.841785722321695573, 13.82664651025757152, 44.21024514465928235 ) ) ;
#1718=CARTESIAN_POINT ( 'NONE',  ( -4.619798703721853528, -13.59724543428036725, 18.06738800180213644 ) ) ;
#1721=CARTESIAN_POINT ( 'NONE',  ( 1.791431617652837316, 15.89939535829188877, 36.85714285714286120 ) ) ;
#1722=CARTESIAN_POINT ( 'NONE',  ( 1.441234910513245149, 13.92619789766829008, 38.85310228751641404 ) ) ;
#1727=CARTESIAN_POINT ( 'NONE',  ( -13.59724543428031573, -4.619798703722008959, 8.932611998197868886 ) ) ;
#1728=CARTESIAN_POINT ( 'NONE',  ( -7.556039541191334585, -11.78653521626503320, 14.28975485534072298 ) ) ;
#1730=CARTESIAN_POINT ( 'NONE',  ( 1.967016585148662289, -16.29368510291087091, 5.638816573230711171 ) ) ;
#1736=CARTESIAN_POINT ( 'NONE',  ( -15.53355953199861794, -5.297344310588530725, 32.93261199819787777 ) ) ;
#1738=CARTESIAN_POINT ( 'NONE',  ( 15.89939535829187278, 1.791431617653015174, 26.14285714285714590 ) ) ;
#1739=CARTESIAN_POINT ( 'NONE',  ( 3.523512929767037338, 14.36041041362159554, 8.096169431371280833E-17 ) ) ;
#1740=CARTESIAN_POINT ( 'NONE',  ( 11.60466159355862104, 11.60466159355875071, 7.500000000000005329 ) ) ;
#1744=CARTESIAN_POINT ( 'NONE',  ( -11.22385875690717327, 11.40355824106234550, -1.995959430373561272 ) ) ;
#1746=CARTESIAN_POINT ( 'NONE',  ( -1.837501619626328297, 16.30827793483733856, 12.64285714285714235 ) ) ;
#1747=CARTESIAN_POINT ( 'NONE',  ( 13.21436662431716869, -4.623906867372263640, 32.57142857142856940 ) ) ;
#1748=CARTESIAN_POINT ( 'NONE',  ( 5.543385399275644332, 15.44746603149420494, -0.9245308589449906522 ) ) ;
#1749=CARTESIAN_POINT ( 'NONE',  ( -4.623906867372410190, 13.21436662431711895, 12.42857142857142705 ) ) ;
#1753=CARTESIAN_POINT ( 'NONE',  ( 7.448449071214646722, 11.85413878919601594, 1.285714285714285809 ) ) ;
#1755=CARTESIAN_POINT ( 'NONE',  ( -11.31370849898482156, 11.31370849898469544, 24.00000000000000000 ) ) ;
#1756=CARTESIAN_POINT ( 'NONE',  ( 15.44746603149413922, 5.543385399275817527, 39.92453085894499054 ) ) ;
#1759=CARTESIAN_POINT ( 'NONE',  ( 9.899494936611718643, -9.899494936611608509, 3.000000000000002665 ) ) ;
#1761=CARTESIAN_POINT ( 'NONE',  ( 7.750357176954296712, -12.08964793087877787, 11.21024514465928235 ) ) ;
#1764=CARTESIAN_POINT ( 'NONE',  ( 7.340858601237956194, 11.92174236212700045, 39.28167371608785174 ) ) ;
#1769=CARTESIAN_POINT ( 'NONE',  ( -4.865839792409144771, -13.51115193377589740, 14.07546914105500768 ) ) ;
#1771=CARTESIAN_POINT ( 'NONE',  ( -9.809645194534070356, 9.989344678689256796, 16.00404056962643651 ) ) ;
#1774=CARTESIAN_POINT ( 'NONE',  ( -1.665163862719845067, -15.91362231745477374, 5.853102287516418478 ) ) ;
#1780=CARTESIAN_POINT ( 'NONE',  ( 11.69682198916835070, 11.51250119794901394, 23.50404056962643295 ) ) ;
#1781=CARTESIAN_POINT ( 'NONE',  ( 4.623906867372411078, -13.21436662431711717, 33.42857142857143060 ) ) ;
#1782=CARTESIAN_POINT ( 'NONE',  ( 16.29368510291089223, -1.967016585148476882, 36.36118342676930126 ) ) ;
#1785=CARTESIAN_POINT ( 'NONE',  ( 11.60466159355862104, 11.60466159355875071, 25.50000000000000711 ) ) ;
#1787=CARTESIAN_POINT ( 'NONE',  ( 1.791431617652837316, 15.89939535829188877, 12.85714285714285943 ) ) ;
#1792=CARTESIAN_POINT ( 'NONE',  ( -1.707986654103994528, 16.32287076676380266, -1.353102287516420921 ) ) ;
#1793=CARTESIAN_POINT ( 'NONE',  ( 1.837501619626330074, -16.30827793483733501, 9.642857142857147679 ) ) ;
#1794=CARTESIAN_POINT ( 'NONE',  ( -4.623906867372410190, 13.21436662431711895, 48.42857142857143060 ) ) ;
#1795=CARTESIAN_POINT ( 'NONE',  ( -7.556039541191334585, -11.78653521626503320, 38.28975485534072476 ) ) ;
#1796=CARTESIAN_POINT ( 'NONE',  ( 13.21436662431716869, -4.623906867372263640, 14.57142857142856940 ) ) ;
#1799=CARTESIAN_POINT ( 'NONE',  ( -9.899494936611716867, 9.899494936611610285, 18.00000000000000355 ) ) ;
#1800=EDGE_LOOP ( 'NONE', ( #7175, #1286 ) ) ;
#1802=CARTESIAN_POINT ( 'NONE',  ( 8.512513224245308763, 13.54758718765259040, 13.28571428571429003 ) ) ;
#1803=CARTESIAN_POINT ( 'NONE',  ( -11.40355824106246807, 11.22385875690704715, 31.99595943037357060 ) ) ;
#1807=CARTESIAN_POINT ( 'NONE',  ( 13.91197093850538380, 1.567502665446386390, 14.14285714285714413 ) ) ;
#1809=CARTESIAN_POINT ( 'NONE',  ( -4.743843029824828861, 13.17239914596749450, 14.42453085894499232 ) ) ;
#1813=CARTESIAN_POINT ( 'NONE',  ( 13.51115193377584589, 4.865839792409294873, 39.92453085894499054 ) ) ;
#1817=CARTESIAN_POINT ( 'NONE',  ( -14.25515036105622890, 1.737328882695209575, 15.36118342676929771 ) ) ;
#1819=CARTESIAN_POINT ( 'NONE',  ( -14.25515036105622890, 1.737328882695209575, 21.36118342676929771 ) ) ;
#1821=CARTESIAN_POINT ( 'NONE',  ( -5.297344310588352201, -15.53355953199867301, 12.06738800180214000 ) ) ;
#1830=CARTESIAN_POINT ( 'NONE',  ( -10.15407889436378852, -10.15407889436390576, 28.50000000000001066 ) ) ;
#1831=CARTESIAN_POINT ( 'NONE',  ( 8.620103694221997515, 13.47998361472160767, 41.28975485534072476 ) ) ;
#1835=CARTESIAN_POINT ( 'NONE',  ( 8.512513224245308763, 13.54758718765259040, 31.28571428571428470 ) ) ;
#1837=CARTESIAN_POINT ( 'NONE',  ( 13.54758718765249803, 8.512513224245457977, 19.71428571428571175 ) ) ;
#1838=EDGE_CURVE ( 'NONE', #7160, #3093, #1412, .T. ) ;
#1845=CARTESIAN_POINT ( 'NONE',  ( 15.06016580658428694, -5.404401153735007846, 12.57546914105500768 ) ) ;
#1846=CARTESIAN_POINT ( 'NONE',  ( -16.30827793483735988, 1.837501619626141780, 29.35714285714285765 ) ) ;
#1848=CARTESIAN_POINT ( 'NONE',  ( 11.22385875690717683, -11.40355824106234373, 1.004040569626440726 ) ) ;
#1850=CARTESIAN_POINT ( 'NONE',  ( -4.742819248065502258, -13.55419868402813677, 16.07142857142857650 ) ) ;
#1854=CARTESIAN_POINT ( 'NONE',  ( 7.639999817571789364, -12.15899005565156266, 21.21428571428571885 ) ) ;
#1856=CARTESIAN_POINT ( 'NONE',  ( 8.512513224245308763, 13.54758718765259040, 31.28571428571428470 ) ) ;
#1857=CARTESIAN_POINT ( 'NONE',  ( 1.665163862719847732, 15.91362231745477374, 32.85310228751642114 ) ) ;
#1860=CARTESIAN_POINT ( 'NONE',  ( -13.21436662431716869, 4.623906867372262752, 5.571428571428574728 ) ) ;
#1862=CARTESIAN_POINT ( 'NONE',  ( -4.619798703721853528, -13.59724543428036725, 24.06738800180213644 ) ) ;
#1867=CARTESIAN_POINT ( 'NONE',  ( -7.340858601237953529, -11.92174236212700222, 36.28167371608785174 ) ) ;
#1872=CARTESIAN_POINT ( 'NONE',  ( -7.556039541191334585, -11.78653521626503320, 20.28975485534072121 ) ) ;
#1876=CARTESIAN_POINT ( 'NONE',  ( -13.47998361472151174, -8.620103694222146729, 42.71024514465928235 ) ) ;
#1878=CARTESIAN_POINT ( 'NONE',  ( -6.655197264005453306, 14.52795920839829513, 48.73000000000004661 ) ) ;
#1879=CARTESIAN_POINT ( 'NONE',  ( -5.284464991282755264, 15.10213328493384743, 18.42857142857143415 ) ) ;
#1880=CARTESIAN_POINT ( 'NONE',  ( 16.32287076676382043, -1.707986654103810897, 10.35310228751642292 ) ) ;
#1886=CARTESIAN_POINT ( 'NONE',  ( 13.21436662431716869, -4.623906867372263640, 26.57142857142857295 ) ) ;
#1887=CARTESIAN_POINT ( 'NONE',  ( 14.26974319298268767, -1.607813917172876916, 32.35714285714286120 ) ) ;
#1890=CARTESIAN_POINT ( 'NONE',  ( -16.30827793483735988, 1.837501619626141780, 47.35714285714286120 ) ) ;
#1892=CARTESIAN_POINT ( 'NONE',  ( -13.54758718765249625, -8.512513224245459753, 10.71428571428571708 ) ) ;
#1896=CARTESIAN_POINT ( 'NONE',  ( 11.22385875690717683, -11.40355824106234373, 7.004040569626434731 ) ) ;
#1897=CARTESIAN_POINT ( 'NONE',  ( -15.49051278174638036, -5.420364854932175902, 22.92857142857142705 ) ) ;
#1899=CARTESIAN_POINT ( 'NONE',  ( 5.164528828830335705, -15.14410076328347543, 1.432611998197868219 ) ) ;
#1900=CARTESIAN_POINT ( 'NONE',  ( -12.15899005565164792, 7.639999817571651697, 11.78571428571428115 ) ) ;
#1904=CARTESIAN_POINT ( 'NONE',  ( -1.567502665446231180, -13.91197093850540334, 15.85714285714286120 ) ) ;
#1906=CARTESIAN_POINT ( 'NONE',  ( -1.791431617652833763, -15.89939535829188877, 33.85714285714285410 ) ) ;
#1907=CARTESIAN_POINT ( 'NONE',  ( 15.14410076328353227, -5.164528828830166063, 46.56738800180214355 ) ) ;
#1910=CARTESIAN_POINT ( 'NONE',  ( -10.15407889436378852, -10.15407889436390398, 16.50000000000000000 ) ) ;
#1911=CARTESIAN_POINT ( 'NONE',  ( 12.22833218042443271, -7.529642458189144349, 22.78167371608784464 ) ) ;
#1915=CARTESIAN_POINT ( 'NONE',  ( 4.619798703721856192, 13.59724543428036725, 39.06738800180213644 ) ) ;
#1919=CARTESIAN_POINT ( 'NONE',  ( -12.08964793087886314, 7.750357176954159932, 15.78975485534072121 ) ) ;
#1920=CARTESIAN_POINT ( 'NONE',  ( -4.503970704919988854, 13.25633410266674517, 28.43261199819786356 ) ) ;
#1922=CARTESIAN_POINT ( 'NONE',  ( -1.665163862719845067, -15.91362231745477374, 35.85310228751641404 ) ) ;
#1923=CARTESIAN_POINT ( 'NONE',  ( -8.870817433266022789, 13.12422867397192583, 48.72999999999998266 ) ) ;
#1924=CARTESIAN_POINT ( 'NONE',  ( 15.10213328493390783, -5.284464991282587398, 20.57142857142857295 ) ) ;
#1925=CARTESIAN_POINT ( 'NONE',  ( -5.297344310588352201, -15.53355953199867301, 6.067388001802139996 ) ) ;
#1931=CARTESIAN_POINT ( 'NONE',  ( -9.899494936611716867, 9.899494936611610285, 36.00000000000000711 ) ) ;
#1934=CARTESIAN_POINT ( 'NONE',  ( -14.26974319298268767, 1.607813917172874918, 35.35714285714285410 ) ) ;
#1936=CARTESIAN_POINT ( 'NONE',  ( 1.665163862719847732, 15.91362231745477374, 2.853102287516426916 ) ) ;
#1938=CARTESIAN_POINT ( 'NONE',  ( 1.837501619626330074, -16.30827793483733501, 21.64285714285714590 ) ) ;
#1942=CARTESIAN_POINT ( 'NONE',  ( 15.53355953199861794, 5.297344310588528060, 5.932611998197868886 ) ) ;
#1943=CARTESIAN_POINT ( 'NONE',  ( -1.791431617652833763, -15.89939535829188877, 33.85714285714285410 ) ) ;
#1945=CARTESIAN_POINT ( 'NONE',  ( -9.899494936611716867, 9.899494936611610285, 48.00000000000000000 ) ) ;
#1946=CARTESIAN_POINT ( 'NONE',  ( -13.82664651025767100, 8.841785722321537477, 9.789754855340722983 ) ) ;
#1947=CARTESIAN_POINT ( 'NONE',  ( 9.899494936611718643, -9.899494936611608509, 27.00000000000000355 ) ) ;
#1948=CARTESIAN_POINT ( 'NONE',  ( -15.49051278174638036, -5.420364854932175902, 10.92857142857142883 ) ) ;
#1951=CARTESIAN_POINT ( 'NONE',  ( 7.448449071214646722, 11.85413878919601594, 19.28571428571428825 ) ) ;
#1953=CARTESIAN_POINT ( 'NONE',  ( 8.512513224245308763, 13.54758718765259040, 25.28571428571428470 ) ) ;
#1954=CARTESIAN_POINT ( 'NONE',  ( 8.841785722321695573, -13.82664651025757152, 47.21024514465928235 ) ) ;
#1958=CARTESIAN_POINT ( 'NONE',  ( -14.26974319298268767, 1.607813917172874696, 17.35714285714286120 ) ) ;
#1960=CARTESIAN_POINT ( 'NONE',  ( 14.28433602490915000, -1.478298951650544479, 34.35310228751642825 ) ) ;
#1967=CARTESIAN_POINT ( 'NONE',  ( -1.478298951650703019, 14.28433602490913579, 22.64689771248357530 ) ) ;
#1969=CARTESIAN_POINT ( 'NONE',  ( -14.25515036105622890, 1.737328882695209575, 27.36118342676929416 ) ) ;
#1971=CARTESIAN_POINT ( 'NONE',  ( -15.44746603149413922, -5.543385399275820191, 42.92453085894499054 ) ) ;
#1972=CARTESIAN_POINT ( 'NONE',  ( -13.10871455524824292, 7.195040570839012162, 48.73000000000001819 ) ) ;
#1973=CARTESIAN_POINT ( 'NONE',  ( -11.31370849898482156, 11.31370849898469544, 24.00000000000000000 ) ) ;
#1975=CARTESIAN_POINT ( 'NONE',  ( 13.89774397934249706, 1.693770420379375308, 10.13881657323070762 ) ) ;
#1980=CARTESIAN_POINT ( 'NONE',  ( -13.21436662431716869, 4.623906867372262752, 29.57142857142857650 ) ) ;
#1981=CARTESIAN_POINT ( 'NONE',  ( 1.567502665446232957, 13.91197093850540156, 36.85714285714286120 ) ) ;
#1986=CARTESIAN_POINT ( 'NONE',  ( 13.89598863503046111, -8.731428362939032795, 20.78571428571429180 ) ) ;
#1992=CARTESIAN_POINT ( 'NONE',  ( 11.69682198916835070, 11.51250119794901394, 5.504040569626439172 ) ) ;
#1994=CARTESIAN_POINT ( 'NONE',  ( -15.89939535829186923, -1.791431617653016062, 29.14285714285714235 ) ) ;
#1998=CARTESIAN_POINT ( 'NONE',  ( -0.3021515714675195863, 13.99673906407701729, 48.73000000000003951 ) ) ;
#1999=CARTESIAN_POINT ( 'NONE',  ( 15.91362231745475597, 1.665163862720026255, 12.14689771248358063 ) ) ;
#2000=CARTESIAN_POINT ( 'NONE',  ( 4.742819248065503146, 13.55419868402813677, 25.07142857142858361 ) ) ;
#2002=CARTESIAN_POINT ( 'NONE',  ( 5.284464991282756152, -15.10213328493384743, 39.42857142857143060 ) ) ;
#2004=CARTESIAN_POINT ( 'NONE',  ( -13.55419868402807992, -4.742819248065651472, 16.92857142857143771 ) ) ;
#2006=CARTESIAN_POINT ( 'NONE',  ( 13.54758718765249803, 8.512513224245457977, 37.71428571428571530 ) ) ;
#2007=CARTESIAN_POINT ( 'NONE',  ( -14.28433602490915000, 1.478298951650542481, 7.353102287516419366 ) ) ;
#2010=CARTESIAN_POINT ( 'NONE',  ( 7.448449071214646722, 11.85413878919601594, 13.28571428571429003 ) ) ;
#2012=CARTESIAN_POINT ( 'NONE',  ( 4.619798703721856192, 13.59724543428036725, 27.06738800180213644 ) ) ;
#2019=CARTESIAN_POINT ( 'NONE',  ( -11.92174236212692051, -7.340858601238089420, 26.71832628391215536 ) ) ;
#2021=CARTESIAN_POINT ( 'NONE',  ( 11.51250119794888249, 11.69682198916847682, 45.49595943037356705 ) ) ;
#2022=CARTESIAN_POINT ( 'NONE',  ( -1.642834855697749452, 15.92644139018836746, 48.73000000000002530 ) ) ;
#2024=CARTESIAN_POINT ( 'NONE',  ( 9.989344678689365153, -9.809645194533958446, 16.99595943037355994 ) ) ;
#2028=CARTESIAN_POINT ( 'NONE',  ( -15.53355953199861794, -5.297344310588530725, 38.93261199819787777 ) ) ;
#2029=CARTESIAN_POINT ( 'NONE',  ( 9.899494936611610285, 9.899494936611718643, 49.50000000000000711 ) ) ;
#2030=CARTESIAN_POINT ( 'NONE',  ( 11.85413878919593422, 7.448449071214774619, 37.71428571428571530 ) ) ;
#2031=ORIENTED_EDGE ( 'NONE', *, *, #3459, .F. ) ;
#2032=CARTESIAN_POINT ( 'NONE',  ( 8.512513224245308763, 13.54758718765259040, 43.28571428571429180 ) ) ;
#2034=CARTESIAN_POINT ( 'NONE',  ( 11.31370849898482334, -11.31370849898469366, 33.00000000000000000 ) ) ;
#2043=CARTESIAN_POINT ( 'NONE',  ( -15.91362231745475597, -1.665163862720028254, 9.146897712483580634 ) ) ;
#2044=CARTESIAN_POINT ( 'NONE',  ( 11.60466159355862104, 11.60466159355875071, 37.50000000000002842 ) ) ;
#2047=CARTESIAN_POINT ( 'NONE',  ( 13.82664651025767100, -8.841785722321541030, 6.789754855340717654 ) ) ;
#2048=( BOUNDED_SURFACE ( )  B_SPLINE_SURFACE ( 3, 2, ( 
 ( #6323, #9552, #9454, #6223, #5660, #7110, #4837, #130, #3282, #8038, #8716, #6271, #7885, #2311, #8619, #4688, #1590, #965, #811, #9504, #2409, #3079, #7163, #5457, #7989, #7835, #916, #2458, #5557, #6425, #1638, #9606, #8827, #4890, #2360, #1740, #4785, #6374, #5510, #4115, #5605, #3910, #10165, #7056, #10218, #8186, #7465, #1119, #289, #391, #1892, #9804, #8236, #1017, #4212, #2658, #9027, #4315, #4167, #5752, #1787, #5899, #3489, #3388, #7364, #3541, #9850, #5085, #8291, #2561, #1164, #8136, #9656, #7314, #6521, #6667, #6476, #3432, #9700, #6569, #8086, #5705, #8873, #9753, #5850, #5804, #2754, #237, #2608, #5143, #8920, #9075, #1837, #1212, #8981, #2708, #7261, #1986, #4992, #6619, #5040, #1938, #1071, #186, #3341, #4939, #4263, #7412, #340, #2908, #6768, #10105, #7623, #5953, #6826, #3799, #3635, #5289, #4576, #8446, #543, #7731, #9226, #6878, #5347, #8340, #1313, #10000, #6109, #1426, #1258, #2857, #9132, #3015, #597, #488, #4468, #650, #6935, #2199, #5392, #9899, #8500, #5235, #6715, #4417, #9953, #6159, #3583, #3692, #6002, #6051, #5192, #2806, #2034, #2142, #2960, #1372, #9336, #7566, #9181, #2245, #2087, #8551, #8390, #4363, #4524, #10048, #7516, #441, #7681, #3743, #9286, #7826, #1578, #118, #705, #5444, #4676, #7783, #1477, #3852, #3270, #3900, #6411, #905, #9385, #7044, #1528, #8753, #2445, #4726, #10153, #1681, #4824, #5591, #7872, #6210, #3174, #8605, #798, #852, #753, #6991, #7199, #5498, #68, #7977, #4052, #9588, #20, #10203, #9441, #3067, #2299, #3117, #6258, #2497, #2348, #8657, #3948, #4624, #9491, #7093, #3223, #6310, #6361, #2396, #5545, #9538, #8704, #1625, #4773 ),
 ( #5646, #7920, #4005, #7152, #4299, #6607, #953, #7301, #6558, #275, #9687, #3665, #6801, #8908, #2697, #4978, #9794, #1730, #1774, #1925, #5839, #3420, #2596, #8074, #3470, #2884, #5738, #519, #223, #7400, #9739, #8967, #3328, #4200, #8173, #1107, #5793, #7594, #9016, #1880, #4926, #8022, #1151, #6509, #8815, #4878, #5073, #1821, #2642, #6464, #4102, #5028, #8861, #7247, #4250, #8224, #9978, #8125, #168, #9643, #2549, #5693, #1001, #4152, #3376, #7352, #1058, #324, #9361, #6185, #6907, #627, #10179, #4555, #1402, #2273, #7807, #3095, #6855, #6235, #3044, #8635, #4703, #8527, #5371, #9412, #5259, #7653, #573, #2325, #7706, #4603, #3925, #7755, #7851, #5420, #678, #3775, #1453, #7020, #2993, #6966, #776, #5321, #8577, #730, #3828, #4654, #10076, #3878, #5475, #8477, #6136, #10128, #1557, #1501, #9312, #2117, #7070, #2225, #6396, #6027, #9207, #8418, #1347, #2179, #4501, #3718, #10027, #2937, #6079, #9257, #2373, #5524, #8683, #3145, #4755, #6286, #3980, #1605, #7130, #824, #7900, #9470, #3528, #2073, #1299, #7608, #5836, #3616, #5124, #1197, #5070, #8377, #5884, #4246, #8276, #5223, #1922, #6699, #2844, #9885, #9063, #5987, #7501, #5179, #6751, #6604, #9836, #4348, #4401, #9939, #9791, #1148, #7398, #4452, #9115, #9013, #2739, #528, #3678, #474, #6811, #8168, #2640, #6653, #5024, #2694, #8221, #5789, #1876, #1971, #4296, #425, #3467, #1104, #320, #2787, #1246, #5936, #8964, #7450, #377, #2021, #8328, #7550, #4563, #3936, #10089, #2283, #9988, #10189, #582, #8430, #7030, #6091, #3001, #8644, #9214, #3728, #2947, #6038, #2894, #2128, #1566, #2186, #4711, #9423, #7666, #5332, #10035, #3105, #739 ),
 ( #1462, #6863, #6145, #3887, #9268, #6244, #6975, #2335, #7860, #5380, #9323, #5486, #5269, #1356, #4511, #785, #8487, #8537, #1411, #4611, #7715, #9371, #7765, #636, #691, #3786, #6916, #3838, #10138, #3052, #5428, #1511, #6196, #8587, #4662, #7813, #4913, #9526, #893, #941, #8851, #8741, #3990, #1761, #1664, #2432, #155, #9675, #4863, #104, #8009, #3157, #1043, #5729, #988, #4041, #4086, #8060, #1809, #7289, #9480, #5578, #7236, #8799, #7962, #4965, #8115, #7187, #3362, #3257, #6497, #6296, #3212, #2383, #5532, #1718, #6398, #6348, #8691, #835, #9575, #4812, #2479, #5633, #3312, #6451, #9630, #2533, #3559, #6688, #1186, #2832, #9102, #7488, #312, #3409, #6736, #1911, #8363, #7338, #466, #5059, #9049, #1862, #262, #5108, #4232, #4188, #8263, #1236, #4388, #1138, #8317, #7539, #5011, #9153, #8949, #2012, #8158, #9825, #5166, #3606, #414, #4335, #8206, #9001, #9928, #2680, #9779, #9872, #5923, #7383, #5976, #2062, #5872, #4283, #3452, #5214, #6544, #7437, #9725, #5825, #2778, #2627, #5777, #1093, #2727, #6595, #363, #3512, #6641, #1960, #4598, #7650, #516, #3875, #9253, #5473, #4442, #7804, #2176, #6133, #9204, #7590, #2222, #1344, #1284, #5368, #8574, #1498, #8475, #5416, #4651, #2113, #6232, #6024, #9359, #5256, #6904, #2270, #727, #7752, #1450, #5318, #6076, #7017, #10024, #6852, #674, #3041, #10176, #8414, #3092, #8524, #9410, #2320, #3771, #624, #3662, #6798, #2881, #4498, #9974, #2934, #10072, #569, #2990, #3715, #3825, #9309, #1398, #6963, #4552, #7703, #10125, #6182, #7897, #929, #144, #7952, #7226, #7127, #3297, #6438, #822, #2422, #2469, #9621, #43, #5522, #2523, #3201, #3976 ),
 ( #6336, #4701, #4127, #5569, #5672, #8840, #1753, #6489, #7176, #4752, #9516, #773, #7066, #8214, #8731, #9667, #1652, #4799, #880, #1554, #4902, #4032, #93, #2575, #3248, #7276, #8001, #6386, #9565, #5620, #8050, #8789, #1706, #202, #4851, #4076, #979, #3354, #8632, #7848, #3922, #3139, #6283, #9467, #2370, #8681, #1603, #2620, #7479, #303, #8150, #9040, #8308, #3503, #8993, #6634, #5717, #9917, #4380, #9862, #2672, #9818, #6678, #1230, #3551, #8104, #4227, #2719, #7427, #6584, #456, #3597, #5818, #2767, #1904, #5916, #8886, #8937, #9089, #2004, #355, #9768, #5004, #408, #1799, #5053, #7531, #7376, #4328, #5863, #1951, #251, #1130, #5100, #8250, #1179, #6729, #5158, #4953, #1854, #1033, #4179, #3444, #7328, #3400, #6535, #8198, #9715, #5765, #1085, #4276, #6516, #436, #7407, #3536, #6662, #3427, #385, #9845, #4160, #1207, #1010, #4307, #7308, #1886, #7459, #2748, #9799, #6613, #7359, #1065, #5892, #4987, #1830, #2703, #8231, #9071, #230, #1980, #3481, #5137, #8285, #8976, #5800, #4358, #5700, #8080, #3383, #7511, #6471, #6564, #9649, #2556, #9694, #8867, #2603, #1781, #5745, #5035, #4934, #8914, #5845, #9023, #282, #4206, #8131, #9745, #2652, #1931, #1157, #8180, #1113, #4257, #5079, #333, #2241, #6047, #2902, #6927, #2798, #5186, #8335, #3794, #9176, #2137, #1470, #5280, #5386, #2955, #8441, #8385, #9221, #4571, #538, #4518, #8546, #2852, #6101, #5341, #1365, #2194, #2082, #8495, #1421, #5997, #7616, #7676, #7725, #5230, #483, #645, #1307, #4459, #6873, #6154, #592, #6821, #3737, #3576, #7776, #4619, #10100, #3687, #10043, #3010, #9330, #6709, #5947, #9995, #9280, #9893, #9127, #2029 ),
 ( #1253, #4411, #7560, #3625, #6762, #9947, #9534, #1574, #7195, #9582, #5641, #3894, #1674, #3166, #9487, #3113, #6406, #3943, #2294, #6304, #112, #10198, #1621, #900, #4769, #7087, #4048, #5540, #3219, #4820, #4670, #7866, #2391, #2441, #7970, #1523, #6253, #8809, #9432, #8748, #5493, #4872, #793, #6356, #700, #3265, #7821, #9380, #2490, #7038, #11, #1727, #10148, #748, #2341, #6985, #3847, #3061, #6205, #8651, #5437, #8598, #4721, #8700, #7915, #845, #4000, #7145, #63, #5585, #1145, #9008, #8123, #2544, #9735, #1769, #1053, #7393, #7296, #4097, #3523, #1817, #9788, #1919, #5067, #5882, #2636, #4147, #8903, #163, #6459, #5688, #4975, #5786, #8069, #4197, #7346, #949, #8960, #3322, #2690, #9638, #8216, #3461, #1872, #4291, #5020, #7448, #2735, #9060, #996, #373, #1100, #4243, #219, #1967, #8017, #8858, #7244, #4923, #3371, #6505, #2592, #2125, #8374, #5329, #9985, #7662, #6087, #9111, #5221, #526, #6861, #8485, #2019, #3614, #9881, #3782, #1354, #1244, #1295, #1409, #7713, #2944, #6143, #423, #4562, #5985, #7497, #5176, #4398, #634, #4344, #4450, #7547, #7601, #5933, #3566, #6696, #3674, #3725, #6808, #6914, #8326, #9164, #2891, #8272, #6033, #6745, #10084, #5265, #3000, #4508, #9319, #5117, #1194, #8881, #1026, #7323, #5564, #3349, #4846, #924, #4794, #8098, #5615, #3835, #7996, #1795, #1647, #3291, #2570, #6433, #8783, #5711, #7220, #4897, #6483, #6194, #9560, #4072, #4122, #9662, #9368, #875, #6973, #4173, #8835, #8726, #2465, #4947, #246, #197, #3395, #7761, #6530, #3243, #4610, #2280, #7947, #2232, #1460, #1701, #4027, #139, #3051, #686, #10135, #9616, #974, #2518, #5378, #7170 ),
 ( #8045, #8534, #88, #6381, #5667, #1748, #7270, #9813, #8351, #8931, #3439, #2666, #5760, #9709, #1848, #1269, #1899, #4428, #9141, #7371, #5048, #9763, #6724, #450, #2714, #8145, #9911, #2818, #3592, #5858, #4221, #1173, #6578, #9035, #9084, #8988, #4998, #5202, #3497, #8302, #5963, #2047, #7576, #8245, #5811, #7420, #1080, #298, #8193, #6627, #5095, #498, #6673, #3645, #2615, #1946, #4323, #1125, #4271, #350, #7473, #403, #3546, #9857, #2762, #5910, #1999, #5152, #1225, #4375, #7526, #7793, #3754, #7740, #8615, #6062, #9344, #8559, #6119, #5401, #5300, #1484, #4633, #9236, #606, #659, #712, #8457, #3702, #3861, #1382, #2152, #10113, #9395, #4586, #10058, #3808, #6782, #761, #5451, #7001, #6888, #6947, #10161, #2307, #3075, #9190, #4535, #3027, #8509, #7689, #1538, #4685, #2968, #9295, #9962, #6219, #2867, #10007, #7832, #6011, #1434, #2209, #5355, #2098, #5243, #6169, #8398, #2254, #1322, #4479, #7633, #553, #6834, #2917, #6420, #912, #2557, #8823, #7207, #28, #3125, #6472, #1634, #8081, #7053, #179, #4780, #8762, #1587, #10213, #4832, #3957, #3907, #7985, #961, #4111, #861, #8031, #7256, #4734, #8868, #8665, #1736, #7881, #9546, #4886, #3336, #126, #4061, #7931, #8712, #9650, #2405, #9499, #3278, #5654, #5701, #807, #1782, #4935, #9598, #2506, #4012, #7159, #6264, #5553, #77, #9451, #2356, #5507, #7101, #3182, #6317, #3230, #6368, #2454, #5599, #1691, #1011, #7309, #232, #1831, #3384, #2604, #4162, #4988, #6517, #9695, #5746, #8915, #10067, #1492, #7700, #1444, #2314, #10017, #3036, #2263, #2984, #9353, #9248, #5411, #8569, #2930, #4547, #4594, #4645, #2168, #7645, #7800, #5311, #6073 ),
 ( #9403, #722, #619, #8520, #3868, #6227, #7011, #2879, #8469, #7748, #2218, #1394, #5465, #8626, #3766, #6900, #3657, #10169, #6794, #3712, #3084, #1547, #5364, #6129, #9303, #4694, #511, #669, #9971, #3822, #6021, #6957, #10120, #5254, #6176, #9200, #2110, #8411, #1337, #4491, #565, #6847, #7060, #195, #5562, #1793, #767, #4121, #8723, #2463, #5516, #3914, #8781, #7891, #7841, #1699, #4895, #8043, #4790, #1746, #972, #8676, #2568, #2363, #5665, #1595, #3241, #816, #7267, #8833, #7944, #6278, #3347, #6481, #9660, #872, #4745, #9558, #3970, #4024, #7218, #7120, #10222, #5709, #1645, #6431, #8880, #3132, #9461, #6379, #36, #7168, #3193, #6329, #9510, #86, #5612, #2416, #4844, #7994, #922, #4070, #137, #9614, #3289, #2516, #4322, #1897, #3545, #5810, #1222, #3590, #9908, #8143, #5907, #7418, #3496, #7369, #448, #8191, #6527, #346, #4373, #4218, #5856, #5150, #9032, #1124, #8300, #9811, #7471, #9082, #8927, #5046, #6625, #6672, #1994, #1846, #3438, #9706, #6723, #1170, #1078, #4269, #7525, #2815, #2759, #5961, #244, #9140, #8986, #7321, #4997, #295, #4945, #4172, #2712, #6576, #1943, #5758, #3393, #2613, #5093, #9855, #8242, #8094, #9759, #2665, #1024, #400, #10112, #6833, #6217, #2150, #4583, #2044, #2253, #2865, #497, #5400, #8396, #5297, #711, #1267, #6010, #5242, #8350, #5200, #4426, #3858, #4475, #6999, #1483, #9961, #7632, #2206, #3806, #6167, #9189, #8557, #9294, #4631, #10160, #4532, #1381, #7791, #7575, #3642, #6780, #3073, #552, #604, #2094, #3751, #1321, #1432, #6886, #10006, #7688, #3025, #9234, #2967, #3699, #2915, #7739, #6943, #10057, #657, #6059, #8454, #6116, #5354, #8507 ) ),
 .UNSPECIFIED., .T., .F., .F. ) 
 B_SPLINE_SURFACE_WITH_KNOTS ( ( 4, 3, 4 ),
 ( 3, 2, 2, 2, 2, 2, 2, 2, 2, 2, 2, 2, 2, 2, 2, 2, 2, 2, 2, 2, 2, 2, 2, 2, 2, 2, 2, 2, 2, 2, 2, 2, 2, 2, 2, 2, 2, 2, 2, 2, 2, 2, 2, 2, 2, 2, 2, 2, 2, 2, 2, 2, 2, 2, 2, 2, 2, 2, 2, 2, 2, 2, 2, 2, 2, 2, 2, 2, 2, 2, 2, 2, 2, 2, 2, 2, 2, 2, 2, 2, 2, 2, 2, 2, 2, 2, 2, 2, 2, 2, 2, 2, 2, 2, 2, 2, 2, 2, 2, 2, 2, 2, 2, 2, 2, 2, 2, 2, 2, 2, 2, 2, 2, 2, 2, 2, 3 ),
 ( 0.000000000000000000, 0.5000000000000000000, 1.000000000000000000 ),
 ( 0.000000000000000000, 0.007936507936507936067, 0.01587301587301587213, 0.02380952380952380820, 0.03174603174603174427, 0.03968253968253968034, 0.04761904761904761640, 0.05555555555555555247, 0.06349206349206348854, 0.07142857142857142461, 0.07936507936507936067, 0.08730158730158729674, 0.09523809523809523281, 0.1031746031746031689, 0.1111111111111111049, 0.1190476190476190410, 0.1269841269841269771, 0.1349206349206349131, 0.1428571428571428492, 0.1507936507936507853, 0.1587301587301587213, 0.1666666666666666574, 0.1746031746031745935, 0.1825396825396825295, 0.1904761904761904656, 0.1984126984126984017, 0.2063492063492063378, 0.2142857142857142738, 0.2222222222222222099, 0.2301587301587301460, 0.2380952380952380820, 0.2460317460317460181, 0.2539682539682539542, 0.2619047619047619180, 0.2698412698412698263, 0.2777777777777777901, 0.2857142857142856984, 0.2936507936507936622, 0.3015873015873015706, 0.3095238095238095344, 0.3174603174603174427, 0.3253968253968254065, 0.3333333333333333148, 0.3412698412698412787, 0.3492063492063491870, 0.3571428571428571508, 0.3650793650793650591, 0.3730158730158730229, 0.3809523809523809312, 0.3888888888888888951, 0.3968253968253968034, 0.4047619047619047672, 0.4126984126984126755, 0.4206349206349206393, 0.4285714285714285476, 0.4365079365079365115, 0.4444444444444444198, 0.4523809523809523836, 0.4603174603174602919, 0.4682539682539682557, 0.4761904761904761640, 0.4841269841269841279, 0.4920634920634920362, 0.5000000000000000000, 0.5079365079365079083, 0.5158730158730159276, 0.5238095238095238360, 0.5317460317460317443, 0.5396825396825396526, 0.5476190476190476719, 0.5555555555555555802, 0.5634920634920634885, 0.5714285714285713969, 0.5793650793650794162, 0.5873015873015873245, 0.5952380952380952328, 0.6031746031746031411, 0.6111111111111111605, 0.6190476190476190688, 0.6269841269841269771, 0.6349206349206348854, 0.6428571428571429047, 0.6507936507936508130, 0.6587301587301587213, 0.6666666666666666297, 0.6746031746031746490, 0.6825396825396825573, 0.6904761904761904656, 0.6984126984126983739, 0.7063492063492063933, 0.7142857142857143016, 0.7222222222222222099, 0.7301587301587301182, 0.7380952380952381375, 0.7460317460317460458, 0.7539682539682539542, 0.7619047619047618625, 0.7698412698412698818, 0.7777777777777777901, 0.7857142857142856984, 0.7936507936507936067, 0.8015873015873016261, 0.8095238095238095344, 0.8174603174603174427, 0.8253968253968253510, 0.8333333333333333703, 0.8412698412698412787, 0.8492063492063491870, 0.8571428571428570953, 0.8650793650793651146, 0.8730158730158730229, 0.8809523809523809312, 0.8888888888888888395, 0.8968253968253968589, 0.9047619047619047672, 0.9126984126984126755, 0.9166666666666666297 ),
 .UNSPECIFIED. ) 
 GEOMETRIC_REPRESENTATION_ITEM ( )  RATIONAL_B_SPLINE_SURFACE ( (
 ( 1.000000000000000000, 0.9749279121818236193, 1.000000000000000000, 0.9749279121818236193, 1.000000000000000000, 0.9749279121818236193, 1.000000000000000000, 0.9749279121818236193, 1.000000000000000000, 0.9749279121818236193, 1.000000000000000000, 0.9749279121818236193, 1.000000000000000000, 0.9749279121818236193, 1.000000000000000000, 0.9749279121818236193, 1.000000000000000000, 0.9749279121818236193, 1.000000000000000000, 0.9749279121818236193, 1.000000000000000000, 0.9749279121818236193, 1.000000000000000000, 0.9749279121818236193, 1.000000000000000000, 0.9749279121818236193, 1.000000000000000000, 0.9749279121818236193, 1.000000000000000000, 0.9749279121818236193, 1.000000000000000000, 0.9749279121818236193, 1.000000000000000000, 0.9749279121818236193, 1.000000000000000000, 0.9749279121818236193, 1.000000000000000000, 0.9749279121818236193, 1.000000000000000000, 0.9749279121818236193, 1.000000000000000000, 0.9749279121818236193, 1.000000000000000000, 0.9749279121818236193, 1.000000000000000000, 0.9749279121818236193, 1.000000000000000000, 0.9749279121818236193, 1.000000000000000000, 0.9749279121818236193, 1.000000000000000000, 0.9749279121818236193, 1.000000000000000000, 0.9749279121818236193, 1.000000000000000000, 0.9749279121818236193, 1.000000000000000000, 0.9749279121818236193, 1.000000000000000000, 0.9749279121818236193, 1.000000000000000000, 0.9749279121818236193, 1.000000000000000000, 0.9749279121818236193, 1.000000000000000000, 0.9749279121818236193, 1.000000000000000000, 0.9749279121818236193, 1.000000000000000000, 0.9749279121818236193, 1.000000000000000000, 0.9749279121818236193, 1.000000000000000000, 0.9749279121818236193, 1.000000000000000000, 0.9749279121818236193, 1.000000000000000000, 0.9749279121818236193, 1.000000000000000000, 0.9749279121818236193, 1.000000000000000000, 0.9749279121818236193, 1.000000000000000000, 0.9749279121818236193, 1.000000000000000000, 0.9749279121818236193, 1.000000000000000000, 0.9749279121818236193, 1.000000000000000000, 0.9749279121818236193, 1.000000000000000000, 0.9749279121818236193, 1.000000000000000000, 0.9749279121818236193, 1.000000000000000000, 0.9749279121818236193, 1.000000000000000000, 0.9749279121818236193, 1.000000000000000000, 0.9749279121818236193, 1.000000000000000000, 0.9749279121818236193, 1.000000000000000000, 0.9749279121818236193, 1.000000000000000000, 0.9749279121818236193, 1.000000000000000000, 0.9749279121818236193, 1.000000000000000000, 0.9749279121818236193, 1.000000000000000000, 0.9749279121818236193, 1.000000000000000000, 0.9749279121818236193, 1.000000000000000000, 0.9749279121818236193, 1.000000000000000000, 0.9749279121818236193, 1.000000000000000000, 0.9749279121818236193, 1.000000000000000000, 0.9749279121818236193, 1.000000000000000000, 0.9749279121818236193, 1.000000000000000000, 0.9749279121818236193, 1.000000000000000000, 0.9749279121818236193, 1.000000000000000000, 0.9749279121818236193, 1.000000000000000000, 0.9749279121818236193, 1.000000000000000000, 0.9749279121818236193, 1.000000000000000000, 0.9749279121818236193, 1.000000000000000000, 0.9749279121818236193, 1.000000000000000000, 0.9749279121818236193, 1.000000000000000000, 0.9749279121818236193, 1.000000000000000000, 0.9749279121818236193, 1.000000000000000000, 0.9749279121818236193, 1.000000000000000000, 0.9749279121818236193, 1.000000000000000000, 0.9749279121818236193, 1.000000000000000000, 0.9749279121818236193, 1.000000000000000000, 0.9749279121818236193, 1.000000000000000000, 0.9749279121818236193, 1.000000000000000000, 0.9749279121818236193, 1.000000000000000000, 0.9749279121818236193, 1.000000000000000000, 0.9749279121818236193, 1.000000000000000000, 0.9749279121818236193, 1.000000000000000000, 0.9749279121818236193, 1.000000000000000000, 0.9749279121818236193, 1.000000000000000000, 0.9749279121818236193, 1.000000000000000000, 0.9749279121818236193, 1.000000000000000000, 0.9749279121818236193, 1.000000000000000000, 0.9749279121818236193, 1.000000000000000000, 0.9749279121818236193, 1.000000000000000000, 0.9749279121818236193, 1.000000000000000000, 0.9749279121818236193, 1.000000000000000000, 0.9749279121818236193, 1.000000000000000000, 0.9749279121818236193, 1.000000000000000000, 0.9749279121818236193, 1.000000000000000000, 0.9749279121818236193, 1.000000000000000000, 0.9749279121818236193, 1.000000000000000000, 0.9749279121818236193, 1.000000000000000000, 0.9749279121818236193, 1.000000000000000000, 0.9749279121818236193, 1.000000000000000000, 0.9749279121818236193, 1.000000000000000000, 0.9749279121818236193, 1.000000000000000000, 0.9749279121818236193, 1.000000000000000000, 0.9749279121818236193, 1.000000000000000000, 0.9749279121818236193, 1.000000000000000000, 0.9749279121818236193, 1.000000000000000000, 0.9749279121818236193, 1.000000000000000000, 0.9749279121818236193, 1.000000000000000000, 0.9749279121818236193, 1.000000000000000000, 0.9749279121818236193, 1.000000000000000000, 0.9749279121818236193, 1.000000000000000000, 0.9749279121818236193, 1.000000000000000000, 0.9749279121818236193, 1.000000000000000000, 0.9749279121818236193, 1.000000000000000000, 0.9749279121818236193, 1.000000000000000000, 0.9749279121818236193, 1.000000000000000000, 0.9874639560909117542, 0.9874639560909117542),
 ( 0.3333333333333333703, 0.3249759707272745768, 0.3333333333333333703, 0.3249759707272745768, 0.3333333333333333703, 0.3249759707272745768, 0.3333333333333333703, 0.3249759707272745768, 0.3333333333333333703, 0.3249759707272745768, 0.3333333333333333703, 0.3249759707272745768, 0.3333333333333333703, 0.3249759707272745768, 0.3333333333333333703, 0.3249759707272745768, 0.3333333333333333703, 0.3249759707272745768, 0.3333333333333333703, 0.3249759707272745768, 0.3333333333333333703, 0.3249759707272745768, 0.3333333333333333703, 0.3249759707272745768, 0.3333333333333333703, 0.3249759707272745768, 0.3333333333333333703, 0.3249759707272745768, 0.3333333333333333703, 0.3249759707272745768, 0.3333333333333333703, 0.3249759707272745768, 0.3333333333333333703, 0.3249759707272745768, 0.3333333333333333703, 0.3249759707272745768, 0.3333333333333333703, 0.3249759707272745768, 0.3333333333333333703, 0.3249759707272745768, 0.3333333333333333703, 0.3249759707272745768, 0.3333333333333333703, 0.3249759707272745768, 0.3333333333333333703, 0.3249759707272745768, 0.3333333333333333703, 0.3249759707272745768, 0.3333333333333333703, 0.3249759707272745768, 0.3333333333333333703, 0.3249759707272745768, 0.3333333333333333703, 0.3249759707272745768, 0.3333333333333333703, 0.3249759707272745768, 0.3333333333333333703, 0.3249759707272745768, 0.3333333333333333703, 0.3249759707272745768, 0.3333333333333333703, 0.3249759707272745768, 0.3333333333333333703, 0.3249759707272745768, 0.3333333333333333703, 0.3249759707272745768, 0.3333333333333333703, 0.3249759707272745768, 0.3333333333333333703, 0.3249759707272745768, 0.3333333333333333703, 0.3249759707272745768, 0.3333333333333333703, 0.3249759707272745768, 0.3333333333333333703, 0.3249759707272745768, 0.3333333333333333703, 0.3249759707272745768, 0.3333333333333333703, 0.3249759707272745768, 0.3333333333333333703, 0.3249759707272745768, 0.3333333333333333703, 0.3249759707272745768, 0.3333333333333333703, 0.3249759707272745768, 0.3333333333333333703, 0.3249759707272745768, 0.3333333333333333703, 0.3249759707272745768, 0.3333333333333333703, 0.3249759707272745768, 0.3333333333333333703, 0.3249759707272745768, 0.3333333333333333703, 0.3249759707272745768, 0.3333333333333333703, 0.3249759707272745768, 0.3333333333333333703, 0.3249759707272745768, 0.3333333333333333703, 0.3249759707272745768, 0.3333333333333333703, 0.3249759707272745768, 0.3333333333333333703, 0.3249759707272745768, 0.3333333333333333703, 0.3249759707272745768, 0.3333333333333333703, 0.3249759707272745768, 0.3333333333333333703, 0.3249759707272745768, 0.3333333333333333703, 0.3249759707272745768, 0.3333333333333333703, 0.3249759707272745768, 0.3333333333333333703, 0.3249759707272745768, 0.3333333333333333703, 0.3249759707272745768, 0.3333333333333333703, 0.3249759707272745768, 0.3333333333333333703, 0.3249759707272745768, 0.3333333333333333703, 0.3249759707272745768, 0.3333333333333333703, 0.3249759707272745768, 0.3333333333333333703, 0.3249759707272745768, 0.3333333333333333703, 0.3249759707272745768, 0.3333333333333333703, 0.3249759707272745768, 0.3333333333333333703, 0.3249759707272745768, 0.3333333333333333703, 0.3249759707272745768, 0.3333333333333333703, 0.3249759707272745768, 0.3333333333333333703, 0.3249759707272745768, 0.3333333333333333703, 0.3249759707272745768, 0.3333333333333333703, 0.3249759707272745768, 0.3333333333333333703, 0.3249759707272745768, 0.3333333333333333703, 0.3249759707272745768, 0.3333333333333333703, 0.3249759707272745768, 0.3333333333333333703, 0.3249759707272745768, 0.3333333333333333703, 0.3249759707272745768, 0.3333333333333333703, 0.3249759707272745768, 0.3333333333333333703, 0.3249759707272745768, 0.3333333333333333703, 0.3249759707272745768, 0.3333333333333333703, 0.3249759707272745768, 0.3333333333333333703, 0.3249759707272745768, 0.3333333333333333703, 0.3249759707272745768, 0.3333333333333333703, 0.3249759707272745768, 0.3333333333333333703, 0.3249759707272745768, 0.3333333333333333703, 0.3249759707272745768, 0.3333333333333333703, 0.3249759707272745768, 0.3333333333333333703, 0.3249759707272745768, 0.3333333333333333703, 0.3249759707272745768, 0.3333333333333333703, 0.3249759707272745768, 0.3333333333333333703, 0.3249759707272745768, 0.3333333333333333703, 0.3249759707272745768, 0.3333333333333333703, 0.3249759707272745768, 0.3333333333333333703, 0.3249759707272745768, 0.3333333333333333703, 0.3249759707272745768, 0.3333333333333333703, 0.3249759707272745768, 0.3333333333333333703, 0.3249759707272745768, 0.3333333333333333703, 0.3249759707272745768, 0.3333333333333333703, 0.3249759707272745768, 0.3333333333333333703, 0.3249759707272745768, 0.3333333333333333703, 0.3249759707272745768, 0.3333333333333333703, 0.3249759707272745768, 0.3333333333333333703, 0.3249759707272745768, 0.3333333333333333703, 0.3249759707272745768, 0.3333333333333333703, 0.3249759707272745768, 0.3333333333333333703, 0.3249759707272745768, 0.3333333333333333703, 0.3249759707272745768, 0.3333333333333333703, 0.3249759707272745768, 0.3333333333333333703, 0.3249759707272745768, 0.3333333333333333703, 0.3249759707272745768, 0.3333333333333333703, 0.3249759707272745768, 0.3333333333333333703, 0.3249759707272745768, 0.3333333333333333703, 0.3249759707272745768, 0.3333333333333333703, 0.3249759707272745768, 0.3333333333333333703, 0.3291546520303039736, 0.3291546520303039736),
 ( 0.3333333333333333703, 0.3249759707272745768, 0.3333333333333333703, 0.3249759707272745768, 0.3333333333333333703, 0.3249759707272745768, 0.3333333333333333703, 0.3249759707272745768, 0.3333333333333333703, 0.3249759707272745768, 0.3333333333333333703, 0.3249759707272745768, 0.3333333333333333703, 0.3249759707272745768, 0.3333333333333333703, 0.3249759707272745768, 0.3333333333333333703, 0.3249759707272745768, 0.3333333333333333703, 0.3249759707272745768, 0.3333333333333333703, 0.3249759707272745768, 0.3333333333333333703, 0.3249759707272745768, 0.3333333333333333703, 0.3249759707272745768, 0.3333333333333333703, 0.3249759707272745768, 0.3333333333333333703, 0.3249759707272745768, 0.3333333333333333703, 0.3249759707272745768, 0.3333333333333333703, 0.3249759707272745768, 0.3333333333333333703, 0.3249759707272745768, 0.3333333333333333703, 0.3249759707272745768, 0.3333333333333333703, 0.3249759707272745768, 0.3333333333333333703, 0.3249759707272745768, 0.3333333333333333703, 0.3249759707272745768, 0.3333333333333333703, 0.3249759707272745768, 0.3333333333333333703, 0.3249759707272745768, 0.3333333333333333703, 0.3249759707272745768, 0.3333333333333333703, 0.3249759707272745768, 0.3333333333333333703, 0.3249759707272745768, 0.3333333333333333703, 0.3249759707272745768, 0.3333333333333333703, 0.3249759707272745768, 0.3333333333333333703, 0.3249759707272745768, 0.3333333333333333703, 0.3249759707272745768, 0.3333333333333333703, 0.3249759707272745768, 0.3333333333333333703, 0.3249759707272745768, 0.3333333333333333703, 0.3249759707272745768, 0.3333333333333333703, 0.3249759707272745768, 0.3333333333333333703, 0.3249759707272745768, 0.3333333333333333703, 0.3249759707272745768, 0.3333333333333333703, 0.3249759707272745768, 0.3333333333333333703, 0.3249759707272745768, 0.3333333333333333703, 0.3249759707272745768, 0.3333333333333333703, 0.3249759707272745768, 0.3333333333333333703, 0.3249759707272745768, 0.3333333333333333703, 0.3249759707272745768, 0.3333333333333333703, 0.3249759707272745768, 0.3333333333333333703, 0.3249759707272745768, 0.3333333333333333703, 0.3249759707272745768, 0.3333333333333333703, 0.3249759707272745768, 0.3333333333333333703, 0.3249759707272745768, 0.3333333333333333703, 0.3249759707272745768, 0.3333333333333333703, 0.3249759707272745768, 0.3333333333333333703, 0.3249759707272745768, 0.3333333333333333703, 0.3249759707272745768, 0.3333333333333333703, 0.3249759707272745768, 0.3333333333333333703, 0.3249759707272745768, 0.3333333333333333703, 0.3249759707272745768, 0.3333333333333333703, 0.3249759707272745768, 0.3333333333333333703, 0.3249759707272745768, 0.3333333333333333703, 0.3249759707272745768, 0.3333333333333333703, 0.3249759707272745768, 0.3333333333333333703, 0.3249759707272745768, 0.3333333333333333703, 0.3249759707272745768, 0.3333333333333333703, 0.3249759707272745768, 0.3333333333333333703, 0.3249759707272745768, 0.3333333333333333703, 0.3249759707272745768, 0.3333333333333333703, 0.3249759707272745768, 0.3333333333333333703, 0.3249759707272745768, 0.3333333333333333703, 0.3249759707272745768, 0.3333333333333333703, 0.3249759707272745768, 0.3333333333333333703, 0.3249759707272745768, 0.3333333333333333703, 0.3249759707272745768, 0.3333333333333333703, 0.3249759707272745768, 0.3333333333333333703, 0.3249759707272745768, 0.3333333333333333703, 0.3249759707272745768, 0.3333333333333333703, 0.3249759707272745768, 0.3333333333333333703, 0.3249759707272745768, 0.3333333333333333703, 0.3249759707272745768, 0.3333333333333333703, 0.3249759707272745768, 0.3333333333333333703, 0.3249759707272745768, 0.3333333333333333703, 0.3249759707272745768, 0.3333333333333333703, 0.3249759707272745768, 0.3333333333333333703, 0.3249759707272745768, 0.3333333333333333703, 0.3249759707272745768, 0.3333333333333333703, 0.3249759707272745768, 0.3333333333333333703, 0.3249759707272745768, 0.3333333333333333703, 0.3249759707272745768, 0.3333333333333333703, 0.3249759707272745768, 0.3333333333333333703, 0.3249759707272745768, 0.3333333333333333703, 0.3249759707272745768, 0.3333333333333333703, 0.3249759707272745768, 0.3333333333333333703, 0.3249759707272745768, 0.3333333333333333703, 0.3249759707272745768, 0.3333333333333333703, 0.3249759707272745768, 0.3333333333333333703, 0.3249759707272745768, 0.3333333333333333703, 0.3249759707272745768, 0.3333333333333333703, 0.3249759707272745768, 0.3333333333333333703, 0.3249759707272745768, 0.3333333333333333703, 0.3249759707272745768, 0.3333333333333333703, 0.3249759707272745768, 0.3333333333333333703, 0.3249759707272745768, 0.3333333333333333703, 0.3249759707272745768, 0.3333333333333333703, 0.3249759707272745768, 0.3333333333333333703, 0.3249759707272745768, 0.3333333333333333703, 0.3249759707272745768, 0.3333333333333333703, 0.3249759707272745768, 0.3333333333333333703, 0.3249759707272745768, 0.3333333333333333703, 0.3249759707272745768, 0.3333333333333333703, 0.3249759707272745768, 0.3333333333333333703, 0.3249759707272745768, 0.3333333333333333703, 0.3249759707272745768, 0.3333333333333333703, 0.3249759707272745768, 0.3333333333333333703, 0.3249759707272745768, 0.3333333333333333703, 0.3249759707272745768, 0.3333333333333333703, 0.3249759707272745768, 0.3333333333333333703, 0.3249759707272745768, 0.3333333333333333703, 0.3249759707272745768, 0.3333333333333333703, 0.3291546520303039736, 0.3291546520303039736),
 ( 1.000000000000000000, 0.9749279121818236193, 1.000000000000000000, 0.9749279121818236193, 1.000000000000000000, 0.9749279121818236193, 1.000000000000000000, 0.9749279121818236193, 1.000000000000000000, 0.9749279121818236193, 1.000000000000000000, 0.9749279121818236193, 1.000000000000000000, 0.9749279121818236193, 1.000000000000000000, 0.9749279121818236193, 1.000000000000000000, 0.9749279121818236193, 1.000000000000000000, 0.9749279121818236193, 1.000000000000000000, 0.9749279121818236193, 1.000000000000000000, 0.9749279121818236193, 1.000000000000000000, 0.9749279121818236193, 1.000000000000000000, 0.9749279121818236193, 1.000000000000000000, 0.9749279121818236193, 1.000000000000000000, 0.9749279121818236193, 1.000000000000000000, 0.9749279121818236193, 1.000000000000000000, 0.9749279121818236193, 1.000000000000000000, 0.9749279121818236193, 1.000000000000000000, 0.9749279121818236193, 1.000000000000000000, 0.9749279121818236193, 1.000000000000000000, 0.9749279121818236193, 1.000000000000000000, 0.9749279121818236193, 1.000000000000000000, 0.9749279121818236193, 1.000000000000000000, 0.9749279121818236193, 1.000000000000000000, 0.9749279121818236193, 1.000000000000000000, 0.9749279121818236193, 1.000000000000000000, 0.9749279121818236193, 1.000000000000000000, 0.9749279121818236193, 1.000000000000000000, 0.9749279121818236193, 1.000000000000000000, 0.9749279121818236193, 1.000000000000000000, 0.9749279121818236193, 1.000000000000000000, 0.9749279121818236193, 1.000000000000000000, 0.9749279121818236193, 1.000000000000000000, 0.9749279121818236193, 1.000000000000000000, 0.9749279121818236193, 1.000000000000000000, 0.9749279121818236193, 1.000000000000000000, 0.9749279121818236193, 1.000000000000000000, 0.9749279121818236193, 1.000000000000000000, 0.9749279121818236193, 1.000000000000000000, 0.9749279121818236193, 1.000000000000000000, 0.9749279121818236193, 1.000000000000000000, 0.9749279121818236193, 1.000000000000000000, 0.9749279121818236193, 1.000000000000000000, 0.9749279121818236193, 1.000000000000000000, 0.9749279121818236193, 1.000000000000000000, 0.9749279121818236193, 1.000000000000000000, 0.9749279121818236193, 1.000000000000000000, 0.9749279121818236193, 1.000000000000000000, 0.9749279121818236193, 1.000000000000000000, 0.9749279121818236193, 1.000000000000000000, 0.9749279121818236193, 1.000000000000000000, 0.9749279121818236193, 1.000000000000000000, 0.9749279121818236193, 1.000000000000000000, 0.9749279121818236193, 1.000000000000000000, 0.9749279121818236193, 1.000000000000000000, 0.9749279121818236193, 1.000000000000000000, 0.9749279121818236193, 1.000000000000000000, 0.9749279121818236193, 1.000000000000000000, 0.9749279121818236193, 1.000000000000000000, 0.9749279121818236193, 1.000000000000000000, 0.9749279121818236193, 1.000000000000000000, 0.9749279121818236193, 1.000000000000000000, 0.9749279121818236193, 1.000000000000000000, 0.9749279121818236193, 1.000000000000000000, 0.9749279121818236193, 1.000000000000000000, 0.9749279121818236193, 1.000000000000000000, 0.9749279121818236193, 1.000000000000000000, 0.9749279121818236193, 1.000000000000000000, 0.9749279121818236193, 1.000000000000000000, 0.9749279121818236193, 1.000000000000000000, 0.9749279121818236193, 1.000000000000000000, 0.9749279121818236193, 1.000000000000000000, 0.9749279121818236193, 1.000000000000000000, 0.9749279121818236193, 1.000000000000000000, 0.9749279121818236193, 1.000000000000000000, 0.9749279121818236193, 1.000000000000000000, 0.9749279121818236193, 1.000000000000000000, 0.9749279121818236193, 1.000000000000000000, 0.9749279121818236193, 1.000000000000000000, 0.9749279121818236193, 1.000000000000000000, 0.9749279121818236193, 1.000000000000000000, 0.9749279121818236193, 1.000000000000000000, 0.9749279121818236193, 1.000000000000000000, 0.9749279121818236193, 1.000000000000000000, 0.9749279121818236193, 1.000000000000000000, 0.9749279121818236193, 1.000000000000000000, 0.9749279121818236193, 1.000000000000000000, 0.9749279121818236193, 1.000000000000000000, 0.9749279121818236193, 1.000000000000000000, 0.9749279121818236193, 1.000000000000000000, 0.9749279121818236193, 1.000000000000000000, 0.9749279121818236193, 1.000000000000000000, 0.9749279121818236193, 1.000000000000000000, 0.9749279121818236193, 1.000000000000000000, 0.9749279121818236193, 1.000000000000000000, 0.9749279121818236193, 1.000000000000000000, 0.9749279121818236193, 1.000000000000000000, 0.9749279121818236193, 1.000000000000000000, 0.9749279121818236193, 1.000000000000000000, 0.9749279121818236193, 1.000000000000000000, 0.9749279121818236193, 1.000000000000000000, 0.9749279121818236193, 1.000000000000000000, 0.9749279121818236193, 1.000000000000000000, 0.9749279121818236193, 1.000000000000000000, 0.9749279121818236193, 1.000000000000000000, 0.9749279121818236193, 1.000000000000000000, 0.9749279121818236193, 1.000000000000000000, 0.9749279121818236193, 1.000000000000000000, 0.9749279121818236193, 1.000000000000000000, 0.9749279121818236193, 1.000000000000000000, 0.9749279121818236193, 1.000000000000000000, 0.9749279121818236193, 1.000000000000000000, 0.9749279121818236193, 1.000000000000000000, 0.9749279121818236193, 1.000000000000000000, 0.9874639560909117542, 0.9874639560909117542),
 ( 0.3333333333333333703, 0.3249759707272745768, 0.3333333333333333703, 0.3249759707272745768, 0.3333333333333333703, 0.3249759707272745768, 0.3333333333333333703, 0.3249759707272745768, 0.3333333333333333703, 0.3249759707272745768, 0.3333333333333333703, 0.3249759707272745768, 0.3333333333333333703, 0.3249759707272745768, 0.3333333333333333703, 0.3249759707272745768, 0.3333333333333333703, 0.3249759707272745768, 0.3333333333333333703, 0.3249759707272745768, 0.3333333333333333703, 0.3249759707272745768, 0.3333333333333333703, 0.3249759707272745768, 0.3333333333333333703, 0.3249759707272745768, 0.3333333333333333703, 0.3249759707272745768, 0.3333333333333333703, 0.3249759707272745768, 0.3333333333333333703, 0.3249759707272745768, 0.3333333333333333703, 0.3249759707272745768, 0.3333333333333333703, 0.3249759707272745768, 0.3333333333333333703, 0.3249759707272745768, 0.3333333333333333703, 0.3249759707272745768, 0.3333333333333333703, 0.3249759707272745768, 0.3333333333333333703, 0.3249759707272745768, 0.3333333333333333703, 0.3249759707272745768, 0.3333333333333333703, 0.3249759707272745768, 0.3333333333333333703, 0.3249759707272745768, 0.3333333333333333703, 0.3249759707272745768, 0.3333333333333333703, 0.3249759707272745768, 0.3333333333333333703, 0.3249759707272745768, 0.3333333333333333703, 0.3249759707272745768, 0.3333333333333333703, 0.3249759707272745768, 0.3333333333333333703, 0.3249759707272745768, 0.3333333333333333703, 0.3249759707272745768, 0.3333333333333333703, 0.3249759707272745768, 0.3333333333333333703, 0.3249759707272745768, 0.3333333333333333703, 0.3249759707272745768, 0.3333333333333333703, 0.3249759707272745768, 0.3333333333333333703, 0.3249759707272745768, 0.3333333333333333703, 0.3249759707272745768, 0.3333333333333333703, 0.3249759707272745768, 0.3333333333333333703, 0.3249759707272745768, 0.3333333333333333703, 0.3249759707272745768, 0.3333333333333333703, 0.3249759707272745768, 0.3333333333333333703, 0.3249759707272745768, 0.3333333333333333703, 0.3249759707272745768, 0.3333333333333333703, 0.3249759707272745768, 0.3333333333333333703, 0.3249759707272745768, 0.3333333333333333703, 0.3249759707272745768, 0.3333333333333333703, 0.3249759707272745768, 0.3333333333333333703, 0.3249759707272745768, 0.3333333333333333703, 0.3249759707272745768, 0.3333333333333333703, 0.3249759707272745768, 0.3333333333333333703, 0.3249759707272745768, 0.3333333333333333703, 0.3249759707272745768, 0.3333333333333333703, 0.3249759707272745768, 0.3333333333333333703, 0.3249759707272745768, 0.3333333333333333703, 0.3249759707272745768, 0.3333333333333333703, 0.3249759707272745768, 0.3333333333333333703, 0.3249759707272745768, 0.3333333333333333703, 0.3249759707272745768, 0.3333333333333333703, 0.3249759707272745768, 0.3333333333333333703, 0.3249759707272745768, 0.3333333333333333703, 0.3249759707272745768, 0.3333333333333333703, 0.3249759707272745768, 0.3333333333333333703, 0.3249759707272745768, 0.3333333333333333703, 0.3249759707272745768, 0.3333333333333333703, 0.3249759707272745768, 0.3333333333333333703, 0.3249759707272745768, 0.3333333333333333703, 0.3249759707272745768, 0.3333333333333333703, 0.3249759707272745768, 0.3333333333333333703, 0.3249759707272745768, 0.3333333333333333703, 0.3249759707272745768, 0.3333333333333333703, 0.3249759707272745768, 0.3333333333333333703, 0.3249759707272745768, 0.3333333333333333703, 0.3249759707272745768, 0.3333333333333333703, 0.3249759707272745768, 0.3333333333333333703, 0.3249759707272745768, 0.3333333333333333703, 0.3249759707272745768, 0.3333333333333333703, 0.3249759707272745768, 0.3333333333333333703, 0.3249759707272745768, 0.3333333333333333703, 0.3249759707272745768, 0.3333333333333333703, 0.3249759707272745768, 0.3333333333333333703, 0.3249759707272745768, 0.3333333333333333703, 0.3249759707272745768, 0.3333333333333333703, 0.3249759707272745768, 0.3333333333333333703, 0.3249759707272745768, 0.3333333333333333703, 0.3249759707272745768, 0.3333333333333333703, 0.3249759707272745768, 0.3333333333333333703, 0.3249759707272745768, 0.3333333333333333703, 0.3249759707272745768, 0.3333333333333333703, 0.3249759707272745768, 0.3333333333333333703, 0.3249759707272745768, 0.3333333333333333703, 0.3249759707272745768, 0.3333333333333333703, 0.3249759707272745768, 0.3333333333333333703, 0.3249759707272745768, 0.3333333333333333703, 0.3249759707272745768, 0.3333333333333333703, 0.3249759707272745768, 0.3333333333333333703, 0.3249759707272745768, 0.3333333333333333703, 0.3249759707272745768, 0.3333333333333333703, 0.3249759707272745768, 0.3333333333333333703, 0.3249759707272745768, 0.3333333333333333703, 0.3249759707272745768, 0.3333333333333333703, 0.3249759707272745768, 0.3333333333333333703, 0.3249759707272745768, 0.3333333333333333703, 0.3249759707272745768, 0.3333333333333333703, 0.3249759707272745768, 0.3333333333333333703, 0.3249759707272745768, 0.3333333333333333703, 0.3249759707272745768, 0.3333333333333333703, 0.3249759707272745768, 0.3333333333333333703, 0.3249759707272745768, 0.3333333333333333703, 0.3249759707272745768, 0.3333333333333333703, 0.3249759707272745768, 0.3333333333333333703, 0.3249759707272745768, 0.3333333333333333703, 0.3249759707272745768, 0.3333333333333333703, 0.3249759707272745768, 0.3333333333333333703, 0.3249759707272745768, 0.3333333333333333703, 0.3291546520303039736, 0.3291546520303039736),
 ( 0.3333333333333333703, 0.3249759707272745768, 0.3333333333333333703, 0.3249759707272745768, 0.3333333333333333703, 0.3249759707272745768, 0.3333333333333333703, 0.3249759707272745768, 0.3333333333333333703, 0.3249759707272745768, 0.3333333333333333703, 0.3249759707272745768, 0.3333333333333333703, 0.3249759707272745768, 0.3333333333333333703, 0.3249759707272745768, 0.3333333333333333703, 0.3249759707272745768, 0.3333333333333333703, 0.3249759707272745768, 0.3333333333333333703, 0.3249759707272745768, 0.3333333333333333703, 0.3249759707272745768, 0.3333333333333333703, 0.3249759707272745768, 0.3333333333333333703, 0.3249759707272745768, 0.3333333333333333703, 0.3249759707272745768, 0.3333333333333333703, 0.3249759707272745768, 0.3333333333333333703, 0.3249759707272745768, 0.3333333333333333703, 0.3249759707272745768, 0.3333333333333333703, 0.3249759707272745768, 0.3333333333333333703, 0.3249759707272745768, 0.3333333333333333703, 0.3249759707272745768, 0.3333333333333333703, 0.3249759707272745768, 0.3333333333333333703, 0.3249759707272745768, 0.3333333333333333703, 0.3249759707272745768, 0.3333333333333333703, 0.3249759707272745768, 0.3333333333333333703, 0.3249759707272745768, 0.3333333333333333703, 0.3249759707272745768, 0.3333333333333333703, 0.3249759707272745768, 0.3333333333333333703, 0.3249759707272745768, 0.3333333333333333703, 0.3249759707272745768, 0.3333333333333333703, 0.3249759707272745768, 0.3333333333333333703, 0.3249759707272745768, 0.3333333333333333703, 0.3249759707272745768, 0.3333333333333333703, 0.3249759707272745768, 0.3333333333333333703, 0.3249759707272745768, 0.3333333333333333703, 0.3249759707272745768, 0.3333333333333333703, 0.3249759707272745768, 0.3333333333333333703, 0.3249759707272745768, 0.3333333333333333703, 0.3249759707272745768, 0.3333333333333333703, 0.3249759707272745768, 0.3333333333333333703, 0.3249759707272745768, 0.3333333333333333703, 0.3249759707272745768, 0.3333333333333333703, 0.3249759707272745768, 0.3333333333333333703, 0.3249759707272745768, 0.3333333333333333703, 0.3249759707272745768, 0.3333333333333333703, 0.3249759707272745768, 0.3333333333333333703, 0.3249759707272745768, 0.3333333333333333703, 0.3249759707272745768, 0.3333333333333333703, 0.3249759707272745768, 0.3333333333333333703, 0.3249759707272745768, 0.3333333333333333703, 0.3249759707272745768, 0.3333333333333333703, 0.3249759707272745768, 0.3333333333333333703, 0.3249759707272745768, 0.3333333333333333703, 0.3249759707272745768, 0.3333333333333333703, 0.3249759707272745768, 0.3333333333333333703, 0.3249759707272745768, 0.3333333333333333703, 0.3249759707272745768, 0.3333333333333333703, 0.3249759707272745768, 0.3333333333333333703, 0.3249759707272745768, 0.3333333333333333703, 0.3249759707272745768, 0.3333333333333333703, 0.3249759707272745768, 0.3333333333333333703, 0.3249759707272745768, 0.3333333333333333703, 0.3249759707272745768, 0.3333333333333333703, 0.3249759707272745768, 0.3333333333333333703, 0.3249759707272745768, 0.3333333333333333703, 0.3249759707272745768, 0.3333333333333333703, 0.3249759707272745768, 0.3333333333333333703, 0.3249759707272745768, 0.3333333333333333703, 0.3249759707272745768, 0.3333333333333333703, 0.3249759707272745768, 0.3333333333333333703, 0.3249759707272745768, 0.3333333333333333703, 0.3249759707272745768, 0.3333333333333333703, 0.3249759707272745768, 0.3333333333333333703, 0.3249759707272745768, 0.3333333333333333703, 0.3249759707272745768, 0.3333333333333333703, 0.3249759707272745768, 0.3333333333333333703, 0.3249759707272745768, 0.3333333333333333703, 0.3249759707272745768, 0.3333333333333333703, 0.3249759707272745768, 0.3333333333333333703, 0.3249759707272745768, 0.3333333333333333703, 0.3249759707272745768, 0.3333333333333333703, 0.3249759707272745768, 0.3333333333333333703, 0.3249759707272745768, 0.3333333333333333703, 0.3249759707272745768, 0.3333333333333333703, 0.3249759707272745768, 0.3333333333333333703, 0.3249759707272745768, 0.3333333333333333703, 0.3249759707272745768, 0.3333333333333333703, 0.3249759707272745768, 0.3333333333333333703, 0.3249759707272745768, 0.3333333333333333703, 0.3249759707272745768, 0.3333333333333333703, 0.3249759707272745768, 0.3333333333333333703, 0.3249759707272745768, 0.3333333333333333703, 0.3249759707272745768, 0.3333333333333333703, 0.3249759707272745768, 0.3333333333333333703, 0.3249759707272745768, 0.3333333333333333703, 0.3249759707272745768, 0.3333333333333333703, 0.3249759707272745768, 0.3333333333333333703, 0.3249759707272745768, 0.3333333333333333703, 0.3249759707272745768, 0.3333333333333333703, 0.3249759707272745768, 0.3333333333333333703, 0.3249759707272745768, 0.3333333333333333703, 0.3249759707272745768, 0.3333333333333333703, 0.3249759707272745768, 0.3333333333333333703, 0.3249759707272745768, 0.3333333333333333703, 0.3249759707272745768, 0.3333333333333333703, 0.3249759707272745768, 0.3333333333333333703, 0.3249759707272745768, 0.3333333333333333703, 0.3249759707272745768, 0.3333333333333333703, 0.3249759707272745768, 0.3333333333333333703, 0.3249759707272745768, 0.3333333333333333703, 0.3249759707272745768, 0.3333333333333333703, 0.3249759707272745768, 0.3333333333333333703, 0.3249759707272745768, 0.3333333333333333703, 0.3249759707272745768, 0.3333333333333333703, 0.3249759707272745768, 0.3333333333333333703, 0.3291546520303039736, 0.3291546520303039736),
 ( 1.000000000000000000, 0.9749279121818236193, 1.000000000000000000, 0.9749279121818236193, 1.000000000000000000, 0.9749279121818236193, 1.000000000000000000, 0.9749279121818236193, 1.000000000000000000, 0.9749279121818236193, 1.000000000000000000, 0.9749279121818236193, 1.000000000000000000, 0.9749279121818236193, 1.000000000000000000, 0.9749279121818236193, 1.000000000000000000, 0.9749279121818236193, 1.000000000000000000, 0.9749279121818236193, 1.000000000000000000, 0.9749279121818236193, 1.000000000000000000, 0.9749279121818236193, 1.000000000000000000, 0.9749279121818236193, 1.000000000000000000, 0.9749279121818236193, 1.000000000000000000, 0.9749279121818236193, 1.000000000000000000, 0.9749279121818236193, 1.000000000000000000, 0.9749279121818236193, 1.000000000000000000, 0.9749279121818236193, 1.000000000000000000, 0.9749279121818236193, 1.000000000000000000, 0.9749279121818236193, 1.000000000000000000, 0.9749279121818236193, 1.000000000000000000, 0.9749279121818236193, 1.000000000000000000, 0.9749279121818236193, 1.000000000000000000, 0.9749279121818236193, 1.000000000000000000, 0.9749279121818236193, 1.000000000000000000, 0.9749279121818236193, 1.000000000000000000, 0.9749279121818236193, 1.000000000000000000, 0.9749279121818236193, 1.000000000000000000, 0.9749279121818236193, 1.000000000000000000, 0.9749279121818236193, 1.000000000000000000, 0.9749279121818236193, 1.000000000000000000, 0.9749279121818236193, 1.000000000000000000, 0.9749279121818236193, 1.000000000000000000, 0.9749279121818236193, 1.000000000000000000, 0.9749279121818236193, 1.000000000000000000, 0.9749279121818236193, 1.000000000000000000, 0.9749279121818236193, 1.000000000000000000, 0.9749279121818236193, 1.000000000000000000, 0.9749279121818236193, 1.000000000000000000, 0.9749279121818236193, 1.000000000000000000, 0.9749279121818236193, 1.000000000000000000, 0.9749279121818236193, 1.000000000000000000, 0.9749279121818236193, 1.000000000000000000, 0.9749279121818236193, 1.000000000000000000, 0.9749279121818236193, 1.000000000000000000, 0.9749279121818236193, 1.000000000000000000, 0.9749279121818236193, 1.000000000000000000, 0.9749279121818236193, 1.000000000000000000, 0.9749279121818236193, 1.000000000000000000, 0.9749279121818236193, 1.000000000000000000, 0.9749279121818236193, 1.000000000000000000, 0.9749279121818236193, 1.000000000000000000, 0.9749279121818236193, 1.000000000000000000, 0.9749279121818236193, 1.000000000000000000, 0.9749279121818236193, 1.000000000000000000, 0.9749279121818236193, 1.000000000000000000, 0.9749279121818236193, 1.000000000000000000, 0.9749279121818236193, 1.000000000000000000, 0.9749279121818236193, 1.000000000000000000, 0.9749279121818236193, 1.000000000000000000, 0.9749279121818236193, 1.000000000000000000, 0.9749279121818236193, 1.000000000000000000, 0.9749279121818236193, 1.000000000000000000, 0.9749279121818236193, 1.000000000000000000, 0.9749279121818236193, 1.000000000000000000, 0.9749279121818236193, 1.000000000000000000, 0.9749279121818236193, 1.000000000000000000, 0.9749279121818236193, 1.000000000000000000, 0.9749279121818236193, 1.000000000000000000, 0.9749279121818236193, 1.000000000000000000, 0.9749279121818236193, 1.000000000000000000, 0.9749279121818236193, 1.000000000000000000, 0.9749279121818236193, 1.000000000000000000, 0.9749279121818236193, 1.000000000000000000, 0.9749279121818236193, 1.000000000000000000, 0.9749279121818236193, 1.000000000000000000, 0.9749279121818236193, 1.000000000000000000, 0.9749279121818236193, 1.000000000000000000, 0.9749279121818236193, 1.000000000000000000, 0.9749279121818236193, 1.000000000000000000, 0.9749279121818236193, 1.000000000000000000, 0.9749279121818236193, 1.000000000000000000, 0.9749279121818236193, 1.000000000000000000, 0.9749279121818236193, 1.000000000000000000, 0.9749279121818236193, 1.000000000000000000, 0.9749279121818236193, 1.000000000000000000, 0.9749279121818236193, 1.000000000000000000, 0.9749279121818236193, 1.000000000000000000, 0.9749279121818236193, 1.000000000000000000, 0.9749279121818236193, 1.000000000000000000, 0.9749279121818236193, 1.000000000000000000, 0.9749279121818236193, 1.000000000000000000, 0.9749279121818236193, 1.000000000000000000, 0.9749279121818236193, 1.000000000000000000, 0.9749279121818236193, 1.000000000000000000, 0.9749279121818236193, 1.000000000000000000, 0.9749279121818236193, 1.000000000000000000, 0.9749279121818236193, 1.000000000000000000, 0.9749279121818236193, 1.000000000000000000, 0.9749279121818236193, 1.000000000000000000, 0.9749279121818236193, 1.000000000000000000, 0.9749279121818236193, 1.000000000000000000, 0.9749279121818236193, 1.000000000000000000, 0.9749279121818236193, 1.000000000000000000, 0.9749279121818236193, 1.000000000000000000, 0.9749279121818236193, 1.000000000000000000, 0.9749279121818236193, 1.000000000000000000, 0.9749279121818236193, 1.000000000000000000, 0.9749279121818236193, 1.000000000000000000, 0.9749279121818236193, 1.000000000000000000, 0.9749279121818236193, 1.000000000000000000, 0.9749279121818236193, 1.000000000000000000, 0.9749279121818236193, 1.000000000000000000, 0.9749279121818236193, 1.000000000000000000, 0.9749279121818236193, 1.000000000000000000, 0.9874639560909117542, 0.9874639560909117542) ) ) 
 REPRESENTATION_ITEM ( '' )  SURFACE ( )  );
#2049=CARTESIAN_POINT ( 'NONE',  ( 10.15407889436379030, 10.15407889436390576, 19.50000000000000355 ) ) ;
#2050=CARTESIAN_POINT ( 'NONE',  ( 5.284464991282756152, -15.10213328493384743, 3.428571428571426605 ) ) ;
#2051=CARTESIAN_POINT ( 'NONE',  ( 15.10213328493390783, -5.284464991282587398, 44.57142857142857650 ) ) ;
#2055=CARTESIAN_POINT ( 'NONE',  ( -8.731428362939187338, 13.89598863503036164, 30.21428571428572241 ) ) ;
#2056=CARTESIAN_POINT ( 'NONE',  ( 11.22385875690704715, 11.40355824106246985, 51.49595943037355994 ) ) ;
#2059=CARTESIAN_POINT ( 'NONE',  ( 9.899494936611718643, -9.899494936611608509, 21.00000000000000355 ) ) ;
#2062=CARTESIAN_POINT ( 'NONE',  ( -10.06191849875405531, -10.24623928997363542, 30.49595943037356349 ) ) ;
#2067=CARTESIAN_POINT ( 'NONE',  ( -4.742819248065502258, -13.55419868402813677, 4.071428571428569398 ) ) ;
#2071=EDGE_LOOP ( 'NONE', ( #9101, #6799, #2031, #8766 ) ) ;
#2073=CARTESIAN_POINT ( 'NONE',  ( 5.297344310588354865, 15.53355953199867301, 33.06738800180213644 ) ) ;
#2075=CARTESIAN_POINT ( 'NONE',  ( -12.99366168247997955, 7.244709680106955041, 48.73000000000001819 ) ) ;
#2076=CARTESIAN_POINT ( 'NONE',  ( 15.49051278174638036, 5.420364854932175014, 31.92857142857143415 ) ) ;
#2078=CARTESIAN_POINT ( 'NONE',  ( -1.737328882695368115, 14.25515036105620581, 14.63881657323070939 ) ) ;
#2082=CARTESIAN_POINT ( 'NONE',  ( 4.742819248065503146, 13.55419868402813677, 43.07142857142858361 ) ) ;
#2083=CARTESIAN_POINT ( 'NONE',  ( -11.85413878919593422, -7.448449071214776396, 34.71428571428571530 ) ) ;
#2084=EDGE_LOOP ( 'NONE', ( #7589, #5189 ) ) ;
#2085=CARTESIAN_POINT ( 'NONE',  ( -15.10213328493390961, 5.284464991282586510, 41.57142857142856940 ) ) ;
#2087=CARTESIAN_POINT ( 'NONE',  ( -13.54758718765249625, -8.512513224245459753, 34.71428571428571530 ) ) ;
#2094=CARTESIAN_POINT ( 'NONE',  ( 5.284464991282756152, -15.10213328493384743, 45.42857142857143060 ) ) ;
#2098=CARTESIAN_POINT ( 'NONE',  ( 15.06016580658428694, -5.404401153735007846, 24.57546914105500946 ) ) ;
#2099=CARTESIAN_POINT ( 'NONE',  ( 9.899494936611718643, -9.899494936611608509, 21.00000000000000355 ) ) ;
#2101=FACE_OUTER_BOUND ( 'NONE', #7126, .T. ) ;
#2102=CARTESIAN_POINT ( 'NONE',  ( -5.420364854931999155, -15.49051278174644253, 40.07142857142857650 ) ) ;
#2108=CARTESIAN_POINT ( 'NONE',  ( 5.404401153735178376, -15.06016580658422477, 47.42453085894499765 ) ) ;
#2110=CARTESIAN_POINT ( 'NONE',  ( 13.54758718765249803, 8.512513224245457977, 7.714285714285715301 ) ) ;
#2112=CARTESIAN_POINT ( 'NONE',  ( -9.899494936611716867, 9.899494936611610285, 24.00000000000000000 ) ) ;
#2113=CARTESIAN_POINT ( 'NONE',  ( 4.619798703721856192, 13.59724543428036725, 39.06738800180213644 ) ) ;
#2117=CARTESIAN_POINT ( 'NONE',  ( 5.297344310588354865, 15.53355953199867301, 27.06738800180213644 ) ) ;
#2121=CARTESIAN_POINT ( 'NONE',  ( -7.639999817571787588, 12.15899005565156266, 0.2142857142857168273 ) ) ;
#2125=CARTESIAN_POINT ( 'NONE',  ( 14.25515036105622535, -1.737328882695210241, 24.36118342676929416 ) ) ;
#2128=CARTESIAN_POINT ( 'NONE',  ( -13.96533075980324234, 8.621071003556515677, 49.78167371608785885 ) ) ;
#2130=CARTESIAN_POINT ( 'NONE',  ( 8.512513224245308763, 13.54758718765259040, 25.28571428571428470 ) ) ;
#2132=CARTESIAN_POINT ( 'NONE',  ( 14.28433602490915000, -1.478298951650544479, 22.35310228751642114 ) ) ;
#2136=CARTESIAN_POINT ( 'NONE',  ( 15.06016580658428694, -5.404401153735007846, 42.57546914105501656 ) ) ;
#2137=CARTESIAN_POINT ( 'NONE',  ( 4.623906867372411078, -13.21436662431711717, 39.42857142857143060 ) ) ;
#2138=CARTESIAN_POINT ( 'NONE',  ( 13.92619789766827587, 1.441234910513398582, 6.146897712483580634 ) ) ;
#2139=ORIENTED_EDGE ( 'NONE', *, *, #6893, .F. ) ;
#2140=CARTESIAN_POINT ( 'NONE',  ( -8.404922754268618235, -13.61519076058357491, 6.281673716087846415 ) ) ;
#2141=CARTESIAN_POINT ( 'NONE',  ( -10.84757329356279598, 11.77984370440671569, -1.110223024625157803E-13 ) ) ;
#2142=CARTESIAN_POINT ( 'NONE',  ( 8.731428362939190890, -13.89598863503036164, 33.21428571428571530 ) ) ;
#2149=CARTESIAN_POINT ( 'NONE',  ( 1.707986654103998303, -16.32287076676380266, 19.64689771248358596 ) ) ;
#2150=CARTESIAN_POINT ( 'NONE',  ( 5.420364854932001819, 15.49051278174644430, 37.07142857142857650 ) ) ;
#2152=CARTESIAN_POINT ( 'NONE',  ( 11.69682198916835070, 11.51250119794901394, 17.50404056962643651 ) ) ;
#2155=CARTESIAN_POINT ( 'NONE',  ( -4.623906867372410190, 13.21436662431711895, 24.42857142857143060 ) ) ;
#2156=CARTESIAN_POINT ( 'NONE',  ( 8.512513224245308763, 13.54758718765259040, 7.285714285714284699 ) ) ;
#2157=CARTESIAN_POINT ( 'NONE',  ( 16.30827793483735633, -1.837501619626142890, 44.35714285714287541 ) ) ;
#2161=CARTESIAN_POINT ( 'NONE',  ( 15.49051278174637858, 5.420364854932174126, 43.92857142857143771 ) ) ;
#2165=CARTESIAN_POINT ( 'NONE',  ( 1.441234910513245149, 13.92619789766829008, 8.853102287516419366 ) ) ;
#2167=CARTESIAN_POINT ( 'NONE',  ( 15.10213328493390783, -5.284464991282587398, 8.571428571428569398 ) ) ;
#2168=CARTESIAN_POINT ( 'NONE',  ( 1.917699372585825790, 15.88516839912900203, 46.86118342676930126 ) ) ;
#2170=CARTESIAN_POINT ( 'NONE',  ( -10.15407889436378852, -10.15407889436390398, 28.50000000000000000 ) ) ;
#2173=CARTESIAN_POINT ( 'NONE',  ( -13.17239914596754424, 4.743843029824683200, 21.57546914105500946 ) ) ;
#2176=CARTESIAN_POINT ( 'NONE',  ( -7.340858601237953529, -11.92174236212700222, 36.28167371608785174 ) ) ;
#2179=CARTESIAN_POINT ( 'NONE',  ( 13.96533075980324234, -8.621071003556521006, 28.78167371608785174 ) ) ;
#2180=CARTESIAN_POINT ( 'NONE',  ( -15.49051278174637858, -5.420364854932175014, 4.928571428571430602 ) ) ;
#2182=CARTESIAN_POINT ( 'NONE',  ( -12.22833218042443271, 7.529642458189139909, 49.78167371608785885 ) ) ;
#2186=CARTESIAN_POINT ( 'NONE',  ( -8.841785722321695573, 13.82664651025757152, 50.21024514465927524 ) ) ;
#2189=CARTESIAN_POINT ( 'NONE',  ( 13.89774397934249706, 1.693770420379375308, 16.13881657323070584 ) ) ;
#2193=CARTESIAN_POINT ( 'NONE',  ( -16.29368510291090288, 1.967016585148476215, 45.36118342676930837 ) ) ;
#2194=CARTESIAN_POINT ( 'NONE',  ( 1.567502665446232957, 13.91197093850540156, 42.85714285714285410 ) ) ;
#2195=CARTESIAN_POINT ( 'NONE',  ( -11.85413878919593422, -7.448449071214776396, 46.71428571428571530 ) ) ;
#2197=CARTESIAN_POINT ( 'NONE',  ( -1.665163862719845067, -15.91362231745477374, 11.85310228751642470 ) ) ;
#2199=CARTESIAN_POINT ( 'NONE',  ( -13.89598863503046111, 8.731428362939027465, 29.78571428571428825 ) ) ;
#2206=CARTESIAN_POINT ( 'NONE',  ( -13.89598863503046111, 8.731428362939027465, 41.78571428571430602 ) ) ;
#2209=CARTESIAN_POINT ( 'NONE',  ( 15.91362231745475597, 1.665163862720026255, 24.14689771248357530 ) ) ;
#2210=CARTESIAN_POINT ( 'NONE',  ( -15.10213328493390961, 5.284464991282586510, 17.57142857142856940 ) ) ;
#2211=CARTESIAN_POINT ( 'NONE',  ( 8.282355133173227912, 13.51256563640100872, 48.73000000000003240 ) ) ;
#2215=CARTESIAN_POINT ( 'NONE',  ( -8.731428362939187338, 13.89598863503036164, 42.21428571428571530 ) ) ;
#2217=CARTESIAN_POINT ( 'NONE',  ( 5.420364854932001819, 15.49051278174644430, 1.071428571428570287 ) ) ;
#2218=CARTESIAN_POINT ( 'NONE',  ( 15.89939535829187278, 1.791431617653015174, 2.142857142857140573 ) ) ;
#2219=CARTESIAN_POINT ( 'NONE',  ( 1.567502665446232957, 13.91197093850540156, 24.85714285714285765 ) ) ;
#2220=CARTESIAN_POINT ( 'NONE',  ( 7.529642458189280241, -12.22833218042435099, 37.21832628391215536 ) ) ;
#2222=CARTESIAN_POINT ( 'NONE',  ( -13.89774397934249706, -1.693770420379375974, 37.13881657323070584 ) ) ;
#2225=CARTESIAN_POINT ( 'NONE',  ( 11.51250119794888249, 11.69682198916847682, 27.49595943037356705 ) ) ;
#2226=CARTESIAN_POINT ( 'NONE',  ( -11.31370849898482156, 11.31370849898469544, 5.999999999999998224 ) ) ;
#2229=CARTESIAN_POINT ( 'NONE',  ( 15.14410076328353227, -5.164528828830166063, 28.56738800180213644 ) ) ;
#2232=CARTESIAN_POINT ( 'NONE',  ( -13.92619789766827054, -1.441234910513399470, 45.14689771248358596 ) ) ;
#2236=CARTESIAN_POINT ( 'NONE',  ( -11.78653521626494793, -7.556039541191465148, 30.71024514465928235 ) ) ;
#2240=CARTESIAN_POINT ( 'NONE',  ( -15.53355953199861794, -5.297344310588530725, 44.93261199819787777 ) ) ;
#2241=CARTESIAN_POINT ( 'NONE',  ( 10.15407889436379030, 10.15407889436390576, 37.50000000000002842 ) ) ;
#2242=CARTESIAN_POINT ( 'NONE',  ( 12.08964793087886314, -7.750357176954162597, 0.7897548553407187644 ) ) ;
#2245=CARTESIAN_POINT ( 'NONE',  ( -11.60466159355861926, -11.60466159355875249, 34.50000000000000000 ) ) ;
#2253=CARTESIAN_POINT ( 'NONE',  ( 13.54758718765249803, 8.512513224245457977, 37.71428571428571530 ) ) ;
#2254=CARTESIAN_POINT ( 'NONE',  ( 5.164528828830335705, -15.14410076328347543, 25.43261199819786711 ) ) ;
#2255=CARTESIAN_POINT ( 'NONE',  ( 13.89598863503046111, -8.731428362939032795, 14.78571428571429358 ) ) ;
#2256=CARTESIAN_POINT ( 'NONE',  ( -0.3453160816774686892, 15.99627321608801367, 48.73000000000002530 ) ) ;
#2259=CARTESIAN_POINT ( 'NONE',  ( 15.10213328493390783, -5.284464991282587398, 38.57142857142857650 ) ) ;
#2262=CARTESIAN_POINT ( 'NONE',  ( -1.837501619626328297, 16.30827793483733856, 6.642857142857143238 ) ) ;
#2263=CARTESIAN_POINT ( 'NONE',  ( -13.61519076058348254, -8.404922754268771001, 44.71832628391215536 ) ) ;
#2265=CARTESIAN_POINT ( 'NONE',  ( -4.623906867372410190, 13.21436662431711895, 18.42857142857143415 ) ) ;
#2266=CARTESIAN_POINT ( 'NONE',  ( -1.693770420379220099, -13.89774397934251837, 31.86118342676929416 ) ) ;
#2270=CARTESIAN_POINT ( 'NONE',  ( 14.28433602490915000, -1.478298951650544479, 40.35310228751642825 ) ) ;
#2273=CARTESIAN_POINT ( 'NONE',  ( -5.297344310588352201, -15.53355953199867301, 18.06738800180213644 ) ) ;
#2274=CARTESIAN_POINT ( 'NONE',  ( 15.89939535829187278, 1.791431617653015174, 8.142857142857145902 ) ) ;
#2276=CARTESIAN_POINT ( 'NONE',  ( 5.404401153735178376, -15.06016580658422477, 29.42453085894499765 ) ) ;
#2280=CARTESIAN_POINT ( 'NONE',  ( -11.92174236212692051, -7.340858601238089420, 44.71832628391215536 ) ) ;
#2283=CARTESIAN_POINT ( 'NONE',  ( 13.96533075980324234, -8.621071003556521006, 46.78167371608785885 ) ) ;
#2285=CARTESIAN_POINT ( 'NONE',  ( 11.60466159355862104, 11.60466159355875071, 31.50000000000001421 ) ) ;
#2289=CARTESIAN_POINT ( 'NONE',  ( -4.619798703721853528, -13.59724543428036725, 24.06738800180213644 ) ) ;
#2293=CARTESIAN_POINT ( 'NONE',  ( -13.82664651025767100, 8.841785722321537477, 45.78975485534073897 ) ) ;
#2294=CARTESIAN_POINT ( 'NONE',  ( -1.693770420379220099, -13.89774397934251837, 1.861183426769295490 ) ) ;
#2295=CARTESIAN_POINT ( 'NONE',  ( 13.59724543428031573, 4.619798703722006294, -0.06738800180213055935 ) ) ;
#2297=CARTESIAN_POINT ( 'NONE',  ( 1.967016585148662289, -16.29368510291087091, 11.63881657323070939 ) ) ;
#2299=CARTESIAN_POINT ( 'NONE',  ( -1.791431617652833763, -15.89939535829188877, 45.85714285714286120 ) ) ;
#2305=CARTESIAN_POINT ( 'NONE',  ( 15.91362231745475597, 1.665163862720026255, 18.14689771248357530 ) ) ;
#2307=CARTESIAN_POINT ( 'NONE',  ( -8.620103694221995738, -13.47998361472161299, 20.28975485534072121 ) ) ;
#2309=CARTESIAN_POINT ( 'NONE',  ( 1.837501619626330074, -16.30827793483733501, 15.64285714285714235 ) ) ;
#2311=CARTESIAN_POINT ( 'NONE',  ( 13.89598863503046111, -8.731428362939032795, 2.785714285714284255 ) ) ;
#2314=CARTESIAN_POINT ( 'NONE',  ( -5.543385399275643444, -15.44746603149420494, 44.07546914105503078 ) ) ;
#2316=CARTESIAN_POINT ( 'NONE',  ( 7.639999817571788476, -12.15899005565156266, 45.21428571428572951 ) ) ;
#2320=CARTESIAN_POINT ( 'NONE',  ( -12.22833218042443271, 7.529642458189139909, 43.78167371608784464 ) ) ;
#2325=CARTESIAN_POINT ( 'NONE',  ( 5.297344310588354865, 15.53355953199867301, 21.06738800180213644 ) ) ;
#2327=CARTESIAN_POINT ( 'NONE',  ( 5.420364854932000931, 15.49051278174644075, 1.071428571428570065 ) ) ;
#2328=CARTESIAN_POINT ( 'NONE',  ( -1.665163862719845067, -15.91362231745477374, 29.85310228751642470 ) ) ;
#2335=CARTESIAN_POINT ( 'NONE',  ( 10.06191849875406064, 10.24623928997363187, 3.495959430373559940 ) ) ;
#2337=CARTESIAN_POINT ( 'NONE',  ( 14.28433602490915000, -1.478298951650544479, 28.35310228751642825 ) ) ;
#2341=CARTESIAN_POINT ( 'NONE',  ( -13.17239914596754424, 4.743843029824683200, 9.575469141055007682 ) ) ;
#2342=CLOSED_SHELL ( 'NONE', ( #1235, #3952, #3173, #1659, #7271, #4523 ) ) ;
#2343=CARTESIAN_POINT ( 'NONE',  ( 13.59724543428031573, 4.619798703722006294, 11.93261199819786178 ) ) ;
#2346=CARTESIAN_POINT ( 'NONE',  ( -8.841785722321695573, 13.82664651025757152, 8.210245144659282346 ) ) ;
#2348=CARTESIAN_POINT ( 'NONE',  ( -13.54758718765249625, -8.512513224245459753, 46.71428571428571530 ) ) ;
#2354=CARTESIAN_POINT ( 'NONE',  ( -8.620103694221995738, -13.47998361472161299, 32.28975485534072476 ) ) ;
#2356=CARTESIAN_POINT ( 'NONE',  ( -11.69682198916834892, -11.51250119794901394, 38.50404056962644006 ) ) ;
#2357=CARTESIAN_POINT ( 'NONE',  ( 1.791431617652837316, 15.89939535829188877, 18.85714285714285765 ) ) ;
#2360=CARTESIAN_POINT ( 'NONE',  ( 8.512513224245308763, 13.54758718765259040, 7.285714285714284699 ) ) ;
#2362=CARTESIAN_POINT ( 'NONE',  ( 11.92174236212692229, 7.340858601238088532, 41.71832628391215536 ) ) ;
#2363=CARTESIAN_POINT ( 'NONE',  ( 11.60466159355862104, 11.60466159355875071, 13.50000000000000178 ) ) ;
#2365=CARTESIAN_POINT ( 'NONE',  ( -1.567502665446231180, -13.91197093850540334, 33.85714285714285410 ) ) ;
#2366=CARTESIAN_POINT ( 'NONE',  ( -13.92619789766827054, -1.441234910513399470, 39.14689771248358596 ) ) ;
#2370=CARTESIAN_POINT ( 'NONE',  ( 4.623906867372411078, -13.21436662431711717, 9.428571428571425272 ) ) ;
#2373=CARTESIAN_POINT ( 'NONE',  ( -8.404922754268618235, -13.61519076058357491, 30.28167371608785530 ) ) ;
#2374=CARTESIAN_POINT ( 'NONE',  ( 11.60466159355861926, 11.60466159355874716, 19.50000000000000355 ) ) ;
#2375=CARTESIAN_POINT ( 'NONE',  ( -13.96533075980324234, 8.621071003556515677, 25.78167371608785530 ) ) ;
#2383=CARTESIAN_POINT ( 'NONE',  ( 1.737328882695370558, -14.25515036105620581, 17.63881657323070939 ) ) ;
#2385=CARTESIAN_POINT ( 'NONE',  ( 16.30827793483735633, -1.837501619626142890, 14.35714285714285587 ) ) ;
#2391=CARTESIAN_POINT ( 'NONE',  ( 1.693770420379222319, 13.89774397934251837, 4.861183426769296823 ) ) ;
#2392=CARTESIAN_POINT ( 'NONE',  ( -9.809645194534070356, 9.989344678689256796, 10.00404056962643651 ) ) ;
#2394=CARTESIAN_POINT ( 'NONE',  ( 15.88516839912898071, 1.917699372586004092, 16.13881657323070584 ) ) ;
#2396=CARTESIAN_POINT ( 'NONE',  ( -1.837501619626328297, 16.30827793483733856, 48.64285714285716011 ) ) ;
#2401=CARTESIAN_POINT ( 'NONE',  ( -13.54758718765249625, -8.512513224245459753, 34.71428571428571530 ) ) ;
#2403=CARTESIAN_POINT ( 'NONE',  ( -1.917699372585823570, -15.88516839912900558, 25.86118342676929416 ) ) ;
#2405=CARTESIAN_POINT ( 'NONE',  ( 5.543385399275644332, 15.44746603149420494, 35.07546914105501656 ) ) ;
#2407=CARTESIAN_POINT ( 'NONE',  ( 1.837501619626330074, -16.30827793483733501, 21.64285714285714590 ) ) ;
#2408=CARTESIAN_POINT ( 'NONE',  ( 4.931155215468822739, 15.20764708138552912, 48.73000000000003240 ) ) ;
#2409=CARTESIAN_POINT ( 'NONE',  ( -8.512513224245306986, -13.54758718765259218, 4.285714285714288252 ) ) ;
#2410=EDGE_CURVE ( 'NONE', #6566, #6181, #4234, .T. ) ;
#2415=CARTESIAN_POINT ( 'NONE',  ( -12.08964793087886314, 7.750357176954159932, 45.78975485534073897 ) ) ;
#2416=CARTESIAN_POINT ( 'NONE',  ( 13.89598863503046111, -8.731428362939032795, 20.78571428571429180 ) ) ;
#2417=CARTESIAN_POINT ( 'NONE',  ( 1.567502665446232957, 13.91197093850540156, 36.85714285714286120 ) ) ;
#2418=CARTESIAN_POINT ( 'NONE',  ( 7.556039541191335474, 11.78653521626503320, 35.28975485534072476 ) ) ;
#2422=CARTESIAN_POINT ( 'NONE',  ( -7.750357176954294935, 12.08964793087877787, 50.21024514465927524 ) ) ;
#2425=CARTESIAN_POINT ( 'NONE',  ( 15.49051278174637858, 5.420364854932174126, 13.92857142857143060 ) ) ;
#2426=CARTESIAN_POINT ( 'NONE',  ( -16.32287076676382398, 1.707986654103809343, 25.35310228751642470 ) ) ;
#2430=( NAMED_UNIT ( * ) PLANE_ANGLE_UNIT ( ) SI_UNIT ( $, .RADIAN. ) );
#2432=CARTESIAN_POINT ( 'NONE',  ( 1.737328882695370558, -14.25515036105620581, 11.63881657323070939 ) ) ;
#2441=CARTESIAN_POINT ( 'NONE',  ( 4.865839792409144771, 13.51115193377589740, 5.075469141055008571 ) ) ;
#2442=CARTESIAN_POINT ( 'NONE',  ( 12.08964793087886314, -7.750357176954162597, 12.78975485534072121 ) ) ;
#2445=CARTESIAN_POINT ( 'NONE',  ( -13.54758718765249625, -8.512513224245459753, 40.71428571428571530 ) ) ;
#2451=CARTESIAN_POINT ( 'NONE',  ( 8.620103694221997515, 13.47998361472160767, 23.28975485534072121 ) ) ;
#2454=CARTESIAN_POINT ( 'NONE',  ( -11.22385875690717327, 11.40355824106234550, 40.00404056962644006 ) ) ;
#2456=CARTESIAN_POINT ( 'NONE',  ( -1.837501619626328297, 16.30827793483733856, 36.64285714285714590 ) ) ;
#2457=CARTESIAN_POINT ( 'NONE',  ( 3.853817051969782970, 14.41361677514167283, 2.166671187435320663E-31 ) ) ;
#2458=CARTESIAN_POINT ( 'NONE',  ( -13.89598863503046111, 8.731428362939027465, 5.785714285714282035 ) ) ;
#2462=CARTESIAN_POINT ( 'NONE',  ( -8.621071003556675549, 13.96533075980314642, -1.781673716087850634 ) ) ;
#2463=CARTESIAN_POINT ( 'NONE',  ( -11.60466159355861926, -11.60466159355875249, 10.50000000000000533 ) ) ;
#2464=CARTESIAN_POINT ( 'NONE',  ( 7.639999817571788476, -12.15899005565156266, 33.21428571428571530 ) ) ;
#2465=CARTESIAN_POINT ( 'NONE',  ( 12.08964793087886314, -7.750357176954162597, 42.78975485534072476 ) ) ;
#2469=CARTESIAN_POINT ( 'NONE',  ( -4.743843029824828861, 13.17239914596749450, 50.42453085894499765 ) ) ;
#2471=CARTESIAN_POINT ( 'NONE',  ( 1.837501619626329630, -16.30827793483733501, 15.64285714285714235 ) ) ;
#2472=CARTESIAN_POINT ( 'NONE',  ( -1.967016585148659846, 16.29368510291087091, 32.63881657323070584 ) ) ;
#2479=CARTESIAN_POINT ( 'NONE',  ( -13.25633410266679313, 4.503970704919840529, 19.56738800180213644 ) ) ;
#2481=CARTESIAN_POINT ( 'NONE',  ( -5.420364854931999155, -15.49051278174644253, 16.07142857142857650 ) ) ;
#2483=CARTESIAN_POINT ( 'NONE',  ( -4.743843029824828861, 13.17239914596749450, 44.42453085894499765 ) ) ;
#2490=CARTESIAN_POINT ( 'NONE',  ( -7.556039541191334585, -11.78653521626503320, 8.289754855340721207 ) ) ;
#2492=CARTESIAN_POINT ( 'NONE',  ( 9.809645194534072132, -9.989344678689256796, 13.00404056962644006 ) ) ;
#2497=CARTESIAN_POINT ( 'NONE',  ( -11.60466159355861926, -11.60466159355875249, 46.50000000000002132 ) ) ;
#2503=CARTESIAN_POINT ( 'NONE',  ( -13.61519076058348254, -8.404922754268771001, 26.71832628391215536 ) ) ;
#2506=CARTESIAN_POINT ( 'NONE',  ( 11.22385875690717683, -11.40355824106234373, 37.00404056962644006 ) ) ;
#2508=CARTESIAN_POINT ( 'NONE',  ( -8.731428362939189114, 13.89598863503036341, 30.21428571428572596 ) ) ;
#2509=CARTESIAN_POINT ( 'NONE',  ( 1.595359904487381852, 14.39304130769396828, -1.488941479308433177E-16 ) ) ;
#2515=CARTESIAN_POINT ( 'NONE',  ( 7.556039541191335474, 11.78653521626503320, 41.28975485534072476 ) ) ;
#2516=CARTESIAN_POINT ( 'NONE',  ( -11.60466159355861926, -11.60466159355875249, 22.50000000000000000 ) ) ;
#2517=CARTESIAN_POINT ( 'NONE',  ( -9.899494936611716867, 9.899494936611610285, 42.00000000000000000 ) ) ;
#2518=CARTESIAN_POINT ( 'NONE',  ( 7.556039541191335474, 11.78653521626503320, 47.28975485534072476 ) ) ;
#2519=CARTESIAN_POINT ( 'NONE',  ( 4.742819248065503146, 13.55419868402813677, 13.07142857142857295 ) ) ;
#2523=CARTESIAN_POINT ( 'NONE',  ( 7.340858601237956194, 11.92174236212700045, 51.28167371608785174 ) ) ;
#2526=CARTESIAN_POINT ( 'NONE',  ( -13.89598863503045933, 8.731428362939027465, 23.78571428571429180 ) ) ;
#2528=CARTESIAN_POINT ( 'NONE',  ( -15.44746603149413922, -5.543385399275820191, 30.92453085894499765 ) ) ;
#2533=CARTESIAN_POINT ( 'NONE',  ( -1.737328882695368115, 14.25515036105620581, 20.63881657323070939 ) ) ;
#2538=CARTESIAN_POINT ( 'NONE',  ( -12.22833218042443271, 7.529642458189139909, 43.78167371608784464 ) ) ;
#2544=CARTESIAN_POINT ( 'NONE',  ( 1.478298951650704351, -14.28433602490913579, 13.64689771248357708 ) ) ;
#2546=CARTESIAN_POINT ( 'NONE',  ( 7.529642458189280241, -12.22833218042435099, 13.21832628391215181 ) ) ;
#2548=CARTESIAN_POINT ( 'NONE',  ( 9.899494936611612061, 9.899494936611718643, 49.50000000000000000 ) ) ;
#2549=CARTESIAN_POINT ( 'NONE',  ( 1.665163862719847732, 15.91362231745477374, 14.85310228751642470 ) ) ;
#2555=CARTESIAN_POINT ( 'NONE',  ( 15.53355953199861794, 5.297344310588528060, 23.93261199819786711 ) ) ;
#2556=CARTESIAN_POINT ( 'NONE',  ( 13.21436662431716869, -4.623906867372263640, 32.57142857142856940 ) ) ;
#2557=CARTESIAN_POINT ( 'NONE',  ( -16.29368510291090288, 1.967016585148476215, 27.36118342676929416 ) ) ;
#2559=CARTESIAN_POINT ( 'NONE',  ( 1.837501619626330074, -16.30827793483733501, 27.64285714285714590 ) ) ;
#2560=CARTESIAN_POINT ( 'NONE',  ( -4.309600312599306982, 13.44913272913615465, 3.300085072504084867E-16 ) ) ;
#2561=CARTESIAN_POINT ( 'NONE',  ( 13.89598863503046111, -8.731428362939032795, 14.78571428571429358 ) ) ;
#2567=CARTESIAN_POINT ( 'NONE',  ( -1.478298951650703019, 14.28433602490913579, 46.64689771248358596 ) ) ;
#2568=CARTESIAN_POINT ( 'NONE',  ( 8.512513224245308763, 13.54758718765259040, 13.28571428571429003 ) ) ;
#2570=CARTESIAN_POINT ( 'NONE',  ( -13.59724543428031573, -4.619798703722008959, 38.93261199819787777 ) ) ;
#2571=CARTESIAN_POINT ( 'NONE',  ( -9.899494936611716867, 9.899494936611610285, 11.99999999999999645 ) ) ;
#2575=CARTESIAN_POINT ( 'NONE',  ( -13.55419868402807992, -4.742819248065651472, 4.928571428571430602 ) ) ;
#2578=CARTESIAN_POINT ( 'NONE',  ( 5.284464991282756152, -15.10213328493384743, 15.42857142857143060 ) ) ;
#2580=CARTESIAN_POINT ( 'NONE',  ( -15.14410076328353227, 5.164528828830164287, 37.56738800180213644 ) ) ;
#2583=CARTESIAN_POINT ( 'NONE',  ( 13.55419868402807992, 4.742819248065649695, 13.92857142857143060 ) ) ;
#2587=CARTESIAN_POINT ( 'NONE',  ( -12.22833218042443271, 7.529642458189139909, 37.78167371608785174 ) ) ;
#2592=CARTESIAN_POINT ( 'NONE',  ( 13.92619789766827587, 1.441234910513398582, 24.14689771248357530 ) ) ;
#2593=CARTESIAN_POINT ( 'NONE',  ( 1.478298951650704351, -14.28433602490913579, 19.64689771248358596 ) ) ;
#2596=CARTESIAN_POINT ( 'NONE',  ( -13.47998361472151174, -8.620103694222146729, 6.710245144659284122 ) ) ;
#2602=CARTESIAN_POINT ( 'NONE',  ( -13.82664651025767100, 8.841785722321537477, 39.78975485534073186 ) ) ;
#2603=CARTESIAN_POINT ( 'NONE',  ( 7.639999817571789364, -12.15899005565156266, 33.21428571428571530 ) ) ;
#2604=CARTESIAN_POINT ( 'NONE',  ( 13.61519076058348254, 8.404922754268771001, 41.71832628391215536 ) ) ;
#2606=CARTESIAN_POINT ( 'NONE',  ( 8.731428362939190890, -13.89598863503036164, 27.21428571428572241 ) ) ;
#2607=CARTESIAN_POINT ( 'NONE',  ( -7.292276458266168326, 11.99875552204202833, 2.357314452189448168E-16 ) ) ;
#2608=CARTESIAN_POINT ( 'NONE',  ( 1.791431617652837316, 15.89939535829188877, 18.85714285714285765 ) ) ;
#2612=CARTESIAN_POINT ( 'NONE',  ( 5.164528828830335705, -15.14410076328347543, 13.43261199819786711 ) ) ;
#2613=CARTESIAN_POINT ( 'NONE',  ( -11.60466159355861926, -11.60466159355875249, 34.50000000000000000 ) ) ;
#2614=CARTESIAN_POINT ( 'NONE',  ( -13.21436662431716869, 4.623906867372262752, 47.57142857142857650 ) ) ;
#2615=CARTESIAN_POINT ( 'NONE',  ( -15.06016580658428694, 5.404401153735006957, 9.575469141055007682 ) ) ;
#2616=CARTESIAN_POINT ( 'NONE',  ( -13.91197093850538380, -1.567502665446387278, 11.14285714285714235 ) ) ;
#2620=CARTESIAN_POINT ( 'NONE',  ( -4.742819248065502258, -13.55419868402813677, 10.07142857142856940 ) ) ;
#2622=CARTESIAN_POINT ( 'NONE',  ( 15.10213328493390783, -5.284464991282587398, 26.57142857142857295 ) ) ;
#2623=CARTESIAN_POINT ( 'NONE',  ( 15.44746603149413922, 5.543385399275817527, 33.92453085894499054 ) ) ;
#2626=CARTESIAN_POINT ( 'NONE',  ( -7.448449071214644945, -11.85413878919601771, 16.28571428571428470 ) ) ;
#2627=CARTESIAN_POINT ( 'NONE',  ( -1.737328882695368115, 14.25515036105620581, 32.63881657323070584 ) ) ;
#2632=CARTESIAN_POINT ( 'NONE',  ( -7.340858601237953529, -11.92174236212700222, 42.28167371608785174 ) ) ;
#2636=CARTESIAN_POINT ( 'NONE',  ( -4.503970704919988854, 13.25633410266674517, 16.43261199819786356 ) ) ;
#2640=CARTESIAN_POINT ( 'NONE',  ( 5.404401153735178376, -15.06016580658422477, 41.42453085894499765 ) ) ;
#2642=CARTESIAN_POINT ( 'NONE',  ( -8.404922754268618235, -13.61519076058357491, 12.28167371608784997 ) ) ;
#2651=CARTESIAN_POINT ( 'NONE',  ( 8.621071003556677326, -13.96533075980314287, 37.21832628391215536 ) ) ;
#2652=CARTESIAN_POINT ( 'NONE',  ( -12.15899005565164792, 7.639999817571651697, 35.78571428571429180 ) ) ;
#2656=CARTESIAN_POINT ( 'NONE',  ( 13.89598863503046111, -8.731428362939032795, 26.78571428571429536 ) ) ;
#2658=CARTESIAN_POINT ( 'NONE',  ( -13.89598863503046111, 8.731428362939027465, 11.78571428571428115 ) ) ;
#2659=FACE_OUTER_BOUND ( 'NONE', #2071, .T. ) ;
#2664=CARTESIAN_POINT ( 'NONE',  ( -1.707986654103994528, 16.32287076676380266, 16.64689771248358596 ) ) ;
#2665=CARTESIAN_POINT ( 'NONE',  ( -13.89598863503046111, 8.731428362939027465, 35.78571428571429180 ) ) ;
#2666=CARTESIAN_POINT ( 'NONE',  ( 16.29368510291089223, -1.967016585148476882, 0.3611834267692887734 ) ) ;
#2668=CARTESIAN_POINT ( 'NONE',  ( -9.899494936611716867, 9.899494936611610285, 5.999999999999998224 ) ) ;
#2672=CARTESIAN_POINT ( 'NONE',  ( 1.567502665446232957, 13.91197093850540156, 12.85714285714285943 ) ) ;
#2674=CARTESIAN_POINT ( 'NONE',  ( 11.60466159355861926, 11.60466159355874716, 31.50000000000000711 ) ) ;
#2675=CARTESIAN_POINT ( 'NONE',  ( 16.32287076676382043, -1.707986654103810897, 40.35310228751642825 ) ) ;
#2677=CARTESIAN_POINT ( 'NONE',  ( 7.639999817571788476, -12.15899005565156266, 9.214285714285717077 ) ) ;
#2680=CARTESIAN_POINT ( 'NONE',  ( 7.750357176954296712, -12.08964793087877787, 29.21024514465927879 ) ) ;
#2683=CARTESIAN_POINT ( 'NONE',  ( 3.002363214934308022, 13.70813944144856755, 48.73000000000003240 ) ) ;
#2685=CARTESIAN_POINT ( 'NONE',  ( -14.28433602490915000, 1.478298951650542481, 37.35310228751641404 ) ) ;
#2690=CARTESIAN_POINT ( 'NONE',  ( 4.503970704919991519, -13.25633410266674517, 19.43261199819785645 ) ) ;
#2692=CARTESIAN_POINT ( 'NONE',  ( 12.08964793087886314, -7.750357176954162597, 24.78975485534072476 ) ) ;
#2694=CARTESIAN_POINT ( 'NONE',  ( -5.297344310588352201, -15.53355953199867301, 42.06738800180214355 ) ) ;
#2696=CARTESIAN_POINT ( 'NONE',  ( 16.30827793483735633, -1.837501619626142890, 20.35714285714286476 ) ) ;
#2697=CARTESIAN_POINT ( 'NONE',  ( 11.40355824106246985, -11.22385875690704538, 4.995959430373563492 ) ) ;
#2703=CARTESIAN_POINT ( 'NONE',  ( -11.85413878919593422, -7.448449071214776396, 28.71428571428571530 ) ) ;
#2704=CARTESIAN_POINT ( 'NONE',  ( -10.15407889436378852, -10.15407889436390576, 40.50000000000000711 ) ) ;
#2706=CARTESIAN_POINT ( 'NONE',  ( -1.967016585148659846, 16.29368510291087091, 2.638816573230710727 ) ) ;
#2707=CARTESIAN_POINT ( 'NONE',  ( -1.373322081274849449, 15.69029061493039023, 5.081489463560647903E-16 ) ) ;
#2708=CARTESIAN_POINT ( 'NONE',  ( 16.30827793483735633, -1.837501619626142890, 20.35714285714286476 ) ) ;
#2711=CARTESIAN_POINT ( 'NONE',  ( -15.06016580658428694, 5.404401153735006957, 9.575469141055007682 ) ) ;
#2712=CARTESIAN_POINT ( 'NONE',  ( 5.284464991282756152, -15.10213328493384743, 33.42857142857143060 ) ) ;
#2713=CARTESIAN_POINT ( 'NONE',  ( -12.15899005565164792, 7.639999817571650809, 47.78571428571429891 ) ) ;
#2714=CARTESIAN_POINT ( 'NONE',  ( -15.91362231745475597, -1.665163862720028254, 3.146897712483577969 ) ) ;
#2715=CARTESIAN_POINT ( 'NONE',  ( -1.607813917173034124, 14.26974319298267524, 18.64285714285715656 ) ) ;
#2716=CARTESIAN_POINT ( 'NONE',  ( -5.420364854931999155, -15.49051278174644253, 10.07142857142856940 ) ) ;
#2719=CARTESIAN_POINT ( 'NONE',  ( 14.26974319298268767, -1.607813917172876916, 14.35714285714285587 ) ) ;
#2722=CARTESIAN_POINT ( 'NONE',  ( 1.791431617652837316, 15.89939535829188877, 24.85714285714285765 ) ) ;
#2723=CARTESIAN_POINT ( 'NONE',  ( 12.22833218042443271, -7.529642458189144349, 4.781673716087850856 ) ) ;
#2726=CARTESIAN_POINT ( 'NONE',  ( -13.55419868402807992, -4.742819248065651472, 16.92857142857143060 ) ) ;
#2727=CARTESIAN_POINT ( 'NONE',  ( 7.340858601237956194, 11.92174236212700045, 33.28167371608784464 ) ) ;
#2731=CARTESIAN_POINT ( 'NONE',  ( 4.742819248065503146, 13.55419868402813677, 1.071428571428570287 ) ) ;
#2735=CARTESIAN_POINT ( 'NONE',  ( -13.92619789766827054, -1.441234910513399470, 21.14689771248358241 ) ) ;
#2737=CARTESIAN_POINT ( 'NONE',  ( -13.59724543428031573, -4.619798703722008959, 20.93261199819787066 ) ) ;
#2739=CARTESIAN_POINT ( 'NONE',  ( 15.88516839912898071, 1.917699372586004092, 40.13881657323070584 ) ) ;
#2740=CARTESIAN_POINT ( 'NONE',  ( -8.334518847312166301, 13.50009031046634611, 48.72999999999998977 ) ) ;
#2748=CARTESIAN_POINT ( 'NONE',  ( 9.899494936611718643, -9.899494936611608509, 27.00000000000000355 ) ) ;
#2750=CARTESIAN_POINT ( 'NONE',  ( -13.21436662431716869, 4.623906867372262752, 35.57142857142857650 ) ) ;
#2752=CARTESIAN_POINT ( 'NONE',  ( 5.284464991282756152, -15.10213328493384743, 39.42857142857143060 ) ) ;
#2754=CARTESIAN_POINT ( 'NONE',  ( -5.284464991282755264, 15.10213328493384743, 18.42857142857143415 ) ) ;
#2758=CARTESIAN_POINT ( 'NONE',  ( -15.53355953199861794, -5.297344310588530725, 8.932611998197868886 ) ) ;
#2759=CARTESIAN_POINT ( 'NONE',  ( 8.512513224245308763, 13.54758718765259040, 31.28571428571428470 ) ) ;
#2760=CARTESIAN_POINT ( 'NONE',  ( -1.567502665446231180, -13.91197093850540334, 45.85714285714286120 ) ) ;
#2762=CARTESIAN_POINT ( 'NONE',  ( 13.61519076058348254, 8.404922754268771001, 11.71832628391215181 ) ) ;
#2763=CARTESIAN_POINT ( 'NONE',  ( -7.639999817571787588, 12.15899005565156266, 30.21428571428572596 ) ) ;
#2764=CARTESIAN_POINT ( 'NONE',  ( -5.284464991282755264, 15.10213328493384743, 0.4285714285714309346 ) ) ;
#2765=CARTESIAN_POINT ( 'NONE',  ( 1.837501619626330074, -16.30827793483733501, 45.64285714285716011 ) ) ;
#2766=ORIENTED_EDGE ( 'NONE', *, *, #4241, .T. ) ;
#2767=CARTESIAN_POINT ( 'NONE',  ( 1.607813917173038121, -14.26974319298267346, 15.64285714285714235 ) ) ;
#2770=CARTESIAN_POINT ( 'NONE',  ( 8.512513224245308763, 13.54758718765259040, 37.28571428571429180 ) ) ;
#2771=CARTESIAN_POINT ( 'NONE',  ( 16.32287076676382043, -1.707986654103810897, 46.35310228751641404 ) ) ;
#2775=CARTESIAN_POINT ( 'NONE',  ( -12.15899005565164792, 7.639999817571650809, 11.78571428571428292 ) ) ;
#2778=CARTESIAN_POINT ( 'NONE',  ( -4.743843029824828861, 13.17239914596749450, 32.42453085894499054 ) ) ;
#2779=CARTESIAN_POINT ( 'NONE',  ( 9.449716478673138909, 10.73265495317049023, 48.73000000000004661 ) ) ;
#2787=CARTESIAN_POINT ( 'NONE',  ( -8.841785722321695573, 13.82664651025757152, 44.21024514465928235 ) ) ;
#2789=CARTESIAN_POINT ( 'NONE',  ( -5.498463549856485777, 12.96445134456831383, 48.73000000000003951 ) ) ;
#2790=CARTESIAN_POINT ( 'NONE',  ( 1.791431617652837316, 15.89939535829188877, 18.85714285714285765 ) ) ;
#2792=CARTESIAN_POINT ( 'NONE',  ( -4.743843029824828861, 13.17239914596749450, 14.42453085894499232 ) ) ;
#2797=CARTESIAN_POINT ( 'NONE',  ( -13.82664651025767100, 8.841785722321537477, 33.78975485534073897 ) ) ;
#2798=CARTESIAN_POINT ( 'NONE',  ( 14.26974319298268767, -1.607813917172876916, 38.35714285714287541 ) ) ;
#2799=CARTESIAN_POINT ( 'NONE',  ( 4.623906867372411078, -13.21436662431711717, 33.42857142857143060 ) ) ;
#2803=CARTESIAN_POINT ( 'NONE',  ( 16.30827793483735633, -1.837501619626142890, 44.35714285714287541 ) ) ;
#2806=CARTESIAN_POINT ( 'NONE',  ( 13.89598863503046111, -8.731428362939032795, 32.78571428571430602 ) ) ;
#2814=CARTESIAN_POINT ( 'NONE',  ( 5.543385399275644332, 15.44746603149420494, 11.07546914105500768 ) ) ;
#2815=CARTESIAN_POINT ( 'NONE',  ( 5.420364854932001819, 15.49051278174644430, 31.07142857142857295 ) ) ;
#2818=CARTESIAN_POINT ( 'NONE',  ( -13.82664651025767100, 8.841785722321537477, 3.789754855340718542 ) ) ;
#2819=CARTESIAN_POINT ( 'NONE',  ( 1.607813917173038121, -14.26974319298267346, 27.64285714285714590 ) ) ;
#2820=CARTESIAN_POINT ( 'NONE',  ( 5.284464991282756152, -15.10213328493384743, 9.428571428571425272 ) ) ;
#2821=CARTESIAN_POINT ( 'NONE',  ( 8.512513224245308763, 13.54758718765259040, 43.28571428571429180 ) ) ;
#2825=CARTESIAN_POINT ( 'NONE',  ( 13.54758718765249803, 8.512513224245457977, 25.71428571428571885 ) ) ;
#2826=CARTESIAN_POINT ( 'NONE',  ( -7.750357176954294935, 12.08964793087877787, 2.210245144659280569 ) ) ;
#2830=CARTESIAN_POINT ( 'NONE',  ( -13.21436662431716869, 4.623906867372262752, 23.57142857142857650 ) ) ;
#2832=CARTESIAN_POINT ( 'NONE',  ( 10.06191849875406064, 10.24623928997363187, 21.49595943037356705 ) ) ;
#2835=CARTESIAN_POINT ( 'NONE',  ( 4.853079829769881393, 13.20943203255562359, 48.72999999999996845 ) ) ;
#2837=CARTESIAN_POINT ( 'NONE',  ( 1.607813917173038121, -14.26974319298267346, 3.642857142857144126 ) ) ;
#2844=CARTESIAN_POINT ( 'NONE',  ( -8.404922754268618235, -13.61519076058357491, 36.28167371608785174 ) ) ;
#2845=CARTESIAN_POINT ( 'NONE',  ( -3.603708530703266799, 13.57059942033907873, 48.73000000000004661 ) ) ;
#2848=CARTESIAN_POINT ( 'NONE',  ( -4.619798703721853528, -13.59724543428036725, 18.06738800180213644 ) ) ;
#2852=CARTESIAN_POINT ( 'NONE',  ( -9.899494936611716867, 9.899494936611610285, 42.00000000000000000 ) ) ;
#2853=CARTESIAN_POINT ( 'NONE',  ( 14.26974319298268767, -1.607813917172876916, 38.35714285714287541 ) ) ;
#2855=CARTESIAN_POINT ( 'NONE',  ( 11.31370849898482334, -11.31370849898469366, 39.00000000000000000 ) ) ;
#2857=CARTESIAN_POINT ( 'NONE',  ( -5.420364854931999155, -15.49051278174644253, 28.07142857142857295 ) ) ;
#2864=CARTESIAN_POINT ( 'NONE',  ( -15.53355953199861794, -5.297344310588530725, 20.93261199819787066 ) ) ;
#2865=CARTESIAN_POINT ( 'NONE',  ( 15.49051278174638036, 5.420364854932175014, 37.92857142857143060 ) ) ;
#2867=CARTESIAN_POINT ( 'NONE',  ( 5.543385399275644332, 15.44746603149420494, 23.07546914105501301 ) ) ;
#2868=CARTESIAN_POINT ( 'NONE',  ( -1.567502665446231180, -13.91197093850540334, 21.85714285714286120 ) ) ;
#2870=CARTESIAN_POINT ( 'NONE',  ( -8.731428362939189114, 13.89598863503036341, 0.2142857142857168273 ) ) ;
#2877=CARTESIAN_POINT ( 'NONE',  ( 9.938986324564400121, 12.66818340422679157, 51.38745637415366474 ) ) ;
#2879=CARTESIAN_POINT ( 'NONE',  ( 11.60466159355862104, 11.60466159355875071, 1.500000000000003553 ) ) ;
#2880=CARTESIAN_POINT ( 'NONE',  ( -4.623906867372410190, 13.21436662431711895, 24.42857142857143060 ) ) ;
#2881=CARTESIAN_POINT ( 'NONE',  ( 1.441234910513245149, 13.92619789766829008, 44.85310228751641404 ) ) ;
#2884=CARTESIAN_POINT ( 'NONE',  ( -16.32287076676382398, 1.707986654103809343, 7.353102287516419366 ) ) ;
#2891=CARTESIAN_POINT ( 'NONE',  ( -14.25515036105622890, 1.737328882695209575, 33.36118342676929416 ) ) ;
#2894=CARTESIAN_POINT ( 'NONE',  ( -15.14410076328353227, 5.164528828830164287, 49.56738800180214355 ) ) ;
#2895=CARTESIAN_POINT ( 'NONE',  ( -3.886497728173464061, 15.50039264458562904, 48.73000000000005372 ) ) ;
#2897=CARTESIAN_POINT ( 'NONE',  ( 13.25633410266679313, -4.503970704919842305, 22.56738800180214000 ) ) ;
#2901=CARTESIAN_POINT ( 'NONE',  ( 15.91362231745475597, 1.665163862720026255, 42.14689771248358596 ) ) ;
#2902=CARTESIAN_POINT ( 'NONE',  ( 13.55419868402807992, 4.742819248065648807, 37.92857142857143060 ) ) ;
#2904=CARTESIAN_POINT ( 'NONE',  ( -1.693770420379220099, -13.89774397934251837, 1.861183426769295490 ) ) ;
#2906=CARTESIAN_POINT ( 'NONE',  ( 15.14410076328353227, -5.164528828830166063, 4.567388001802134667 ) ) ;
#2907=CARTESIAN_POINT ( 'NONE',  ( -3.334129424850329482, 15.49830167892402066, 1.394172777290140936E-15 ) ) ;
#2908=CARTESIAN_POINT ( 'NONE',  ( -16.30827793483735988, 1.837501619626141780, 23.35714285714286476 ) ) ;
#2914=CARTESIAN_POINT ( 'NONE',  ( -16.29368510291090288, 1.967016585148476215, 21.36118342676929771 ) ) ;
#2915=CARTESIAN_POINT ( 'NONE',  ( -13.89598863503046111, 8.731428362939027465, 47.78571428571430602 ) ) ;
#2917=CARTESIAN_POINT ( 'NONE',  ( -13.61519076058348254, -8.404922754268771001, 26.71832628391215536 ) ) ;
#2918=CARTESIAN_POINT ( 'NONE',  ( 13.55419868402807992, 4.742819248065648807, 25.92857142857142705 ) ) ;
#2919=CARTESIAN_POINT ( 'NONE',  ( -11.60466159355861926, -11.60466159355875249, 4.500000000000005329 ) ) ;
#2920=CARTESIAN_POINT ( 'NONE',  ( -15.49051278174638036, -5.420364854932175902, 40.92857142857145192 ) ) ;
#2927=CARTESIAN_POINT ( 'NONE',  ( -13.47998361472151174, -8.620103694222146729, 48.71024514465926814 ) ) ;
#2929=CARTESIAN_POINT ( 'NONE',  ( 1.791431617652837316, 15.89939535829188877, 0.8571428571428549859 ) ) ;
#2930=CARTESIAN_POINT ( 'NONE',  ( -11.22385875690717327, 11.40355824106234550, 46.00404056962644006 ) ) ;
#2931=SHAPE_DEFINITION_REPRESENTATION ( #393, #3956 ) ;
#2932=CARTESIAN_POINT ( 'NONE',  ( 1.567502665446232957, 13.91197093850540156, 18.85714285714285765 ) ) ;
#2933=CARTESIAN_POINT ( 'NONE',  ( 9.809645194534072132, -9.989344678689256796, 25.00404056962644006 ) ) ;
#2934=CARTESIAN_POINT ( 'NONE',  ( 10.06191849875406064, 10.24623928997363187, 45.49595943037356705 ) ) ;
#2937=CARTESIAN_POINT ( 'NONE',  ( 1.967016585148662289, -16.29368510291087091, 29.63881657323071295 ) ) ;
#2940=CARTESIAN_POINT ( 'NONE',  ( -7.340858601237953529, -11.92174236212700222, 48.28167371608785174 ) ) ;
#2944=CARTESIAN_POINT ( 'NONE',  ( -1.478298951650703019, 14.28433602490913579, 28.64689771248357886 ) ) ;
#2947=CARTESIAN_POINT ( 'NONE',  ( -15.88516839912898071, -1.917699372586004980, 49.13881657323070584 ) ) ;
#2950=CARTESIAN_POINT ( 'NONE',  ( -7.340858601237953529, -11.92174236212700222, 12.28167371608784997 ) ) ;
#2954=CARTESIAN_POINT ( 'NONE',  ( -8.620103694221995738, -13.47998361472161299, 44.28975485534073186 ) ) ;
#2955=CARTESIAN_POINT ( 'NONE',  ( -7.448449071214644945, -11.85413878919601771, 40.28571428571428470 ) ) ;
#2956=CARTESIAN_POINT ( 'NONE',  ( 7.529642458189280241, -12.22833218042435099, 1.218326283912148922 ) ) ;
#2958=CARTESIAN_POINT ( 'NONE',  ( 1.665163862719847732, 15.91362231745477374, 8.853102287516419366 ) ) ;
#2960=CARTESIAN_POINT ( 'NONE',  ( 5.284464991282756152, -15.10213328493384743, 33.42857142857143060 ) ) ;
#2961=DIRECTION ( 'NONE',  ( 0.000000000000000000, 0.000000000000000000, -1.000000000000000000 ) ) ;
#2967=CARTESIAN_POINT ( 'NONE',  ( -16.30827793483735988, 1.837501619626141780, 47.35714285714286120 ) ) ;
#2968=CARTESIAN_POINT ( 'NONE',  ( -8.621071003556675549, 13.96533075980314642, 22.21832628391215181 ) ) ;
#2971=CARTESIAN_POINT ( 'NONE',  ( -8.731428362939189114, 13.89598863503036341, 12.21428571428571885 ) ) ;
#2977=CARTESIAN_POINT ( 'NONE',  ( -11.60466159355861748, -11.60466159355874893, 40.50000000000000000 ) ) ;
#2983=CARTESIAN_POINT ( 'NONE',  ( -8.731428362939189114, 13.89598863503036341, 0.2142857142857168273 ) ) ;
#2984=CARTESIAN_POINT ( 'NONE',  ( -15.53355953199861794, -5.297344310588530725, 44.93261199819787777 ) ) ;
#2985=CARTESIAN_POINT ( 'NONE',  ( -13.55419868402807992, -4.742819248065651472, 22.92857142857143060 ) ) ;
#2990=CARTESIAN_POINT ( 'NONE',  ( 13.89774397934249706, 1.693770420379375308, 46.13881657323070584 ) ) ;
#2993=CARTESIAN_POINT ( 'NONE',  ( 5.404401153735178376, -15.06016580658422477, 23.42453085894499409 ) ) ;
#2994=CARTESIAN_POINT ( 'NONE',  ( 8.731428362939189114, -13.89598863503035986, 3.214285714285716633 ) ) ;
#2996=CARTESIAN_POINT ( 'NONE',  ( 16.32287076676382043, -1.707986654103810897, 28.35310228751642825 ) ) ;
#3000=CARTESIAN_POINT ( 'NONE',  ( -1.478298951650703019, 14.28433602490913579, 34.64689771248358596 ) ) ;
#3001=CARTESIAN_POINT ( 'NONE',  ( -8.404922754268618235, -13.61519076058357491, 48.28167371608785174 ) ) ;
#3004=CARTESIAN_POINT ( 'NONE',  ( 1.791431617652837316, 15.89939535829188877, 30.85714285714286120 ) ) ;
#3010=CARTESIAN_POINT ( 'NONE',  ( -9.899494936611716867, 9.899494936611610285, 48.00000000000000000 ) ) ;
#3011=CARTESIAN_POINT ( 'NONE',  ( -7.529642458189277576, 12.22833218042435455, -1.781673716087850634 ) ) ;
#3013=CARTESIAN_POINT ( 'NONE',  ( 15.88516839912898071, 1.917699372586004092, 4.138816573230708507 ) ) ;
#3015=CARTESIAN_POINT ( 'NONE',  ( -11.60466159355861926, -11.60466159355875249, 28.50000000000001066 ) ) ;
#3024=CARTESIAN_POINT ( 'NONE',  ( 16.29368510291089223, -1.967016585148476882, 18.36118342676929771 ) ) ;
#3025=CARTESIAN_POINT ( 'NONE',  ( -15.49051278174638036, -5.420364854932175902, 46.92857142857142350 ) ) ;
#3027=CARTESIAN_POINT ( 'NONE',  ( -15.91362231745475597, -1.665163862720028254, 21.14689771248358241 ) ) ;
#3028=CARTESIAN_POINT ( 'NONE',  ( -15.49051278174638036, -5.420364854932175902, 22.92857142857142705 ) ) ;
#3035=CARTESIAN_POINT ( 'NONE',  ( 16.30827793483735633, -1.837501619626142890, 2.357142857142856762 ) ) ;
#3036=CARTESIAN_POINT ( 'NONE',  ( -11.69682198916834892, -11.51250119794901394, 44.50404056962644006 ) ) ;
#3038=CARTESIAN_POINT ( 'NONE',  ( -9.899494936611716867, 9.899494936611610285, 30.00000000000000355 ) ) ;
#3039=CARTESIAN_POINT ( 'NONE',  ( -7.556039541191334585, -11.78653521626503320, 38.28975485534072476 ) ) ;
#3041=CARTESIAN_POINT ( 'NONE',  ( -10.06191849875405531, -10.24623928997363542, 42.49595943037355994 ) ) ;
#3043=CARTESIAN_POINT ( 'NONE',  ( -9.899494936611716867, 9.899494936611610285, 0.000000000000000000 ) ) ;
#3044=CARTESIAN_POINT ( 'NONE',  ( -15.88516839912898071, -1.917699372586004980, 19.13881657323070584 ) ) ;
#3045=CARTESIAN_POINT ( 'NONE',  ( 15.49051278174637858, 5.420364854932174126, 7.928571428571430602 ) ) ;
#3047=CARTESIAN_POINT ( 'NONE',  ( -5.297344310588352201, -15.53355953199867301, 24.06738800180213644 ) ) ;
#3051=CARTESIAN_POINT ( 'NONE',  ( -7.529642458189277576, 12.22833218042435455, 46.21832628391216247 ) ) ;
#3052=CARTESIAN_POINT ( 'NONE',  ( -7.750357176954294935, 12.08964793087877787, 8.210245144659282346 ) ) ;
#3054=CARTESIAN_POINT ( 'NONE',  ( 5.420364854932001819, 15.49051278174644430, 31.07142857142857295 ) ) ;
#3056=CARTESIAN_POINT ( 'NONE',  ( 4.619798703721856192, 13.59724543428036725, 27.06738800180213644 ) ) ;
#3060=CARTESIAN_POINT ( 'NONE',  ( 1.707986654103998303, -16.32287076676380266, 43.64689771248358596 ) ) ;
#3061=CARTESIAN_POINT ( 'NONE',  ( -7.529642458189277576, 12.22833218042435455, 10.21832628391215358 ) ) ;
#3062=CARTESIAN_POINT ( 'NONE',  ( 1.567502665446232957, 13.91197093850540156, 48.85714285714286120 ) ) ;
#3064=CARTESIAN_POINT ( 'NONE',  ( 1.665163862719847732, 15.91362231745477374, 14.85310228751642470 ) ) ;
#3067=CARTESIAN_POINT ( 'NONE',  ( 1.837501619626330074, -16.30827793483733501, 45.64285714285716011 ) ) ;
#3073=CARTESIAN_POINT ( 'NONE',  ( 13.89598863503046111, -8.731428362939032795, 44.78571428571428470 ) ) ;
#3075=CARTESIAN_POINT ( 'NONE',  ( -11.69682198916834892, -11.51250119794901394, 20.50404056962644006 ) ) ;
#3076=CARTESIAN_POINT ( 'NONE',  ( -8.731428362939189114, 13.89598863503036341, 24.21428571428571530 ) ) ;
#3079=CARTESIAN_POINT ( 'NONE',  ( -11.60466159355861926, -11.60466159355875249, 4.500000000000005329 ) ) ;
#3081=CARTESIAN_POINT ( 'NONE',  ( -5.284464991282755264, 15.10213328493384743, 42.42857142857143060 ) ) ;
#3084=CARTESIAN_POINT ( 'NONE',  ( -8.512513224245306986, -13.54758718765259218, 4.285714285714288252 ) ) ;
#3085=CARTESIAN_POINT ( 'NONE',  ( 14.26974319298268767, -1.607813917172876472, 44.35714285714286831 ) ) ;
#3087=CARTESIAN_POINT ( 'NONE',  ( -13.59724543428031573, -4.619798703722008959, 38.93261199819787777 ) ) ;
#3092=CARTESIAN_POINT ( 'NONE',  ( -13.89774397934249706, -1.693770420379375974, 43.13881657323070584 ) ) ;
#3093=VERTEX_POINT ( 'NONE', #9738 ) ;
#3095=CARTESIAN_POINT ( 'NONE',  ( -11.51250119794888072, -11.69682198916848037, 18.49595943037356705 ) ) ;
#3096=CARTESIAN_POINT ( 'NONE',  ( -1.791431617652833763, -15.89939535829188877, 9.857142857142855874 ) ) ;
#3098=CARTESIAN_POINT ( 'NONE',  ( 15.88516839912898071, 1.917699372586004092, 28.13881657323070939 ) ) ;
#3105=CARTESIAN_POINT ( 'NONE',  ( 9.938986324564400121, 12.66818340422679157, 51.38745637415366474 ) ) ;
#3107=CARTESIAN_POINT ( 'NONE',  ( -1.837501619626328297, 16.30827793483733856, 12.64285714285714235 ) ) ;
#3113=CARTESIAN_POINT ( 'NONE',  ( 7.529642458189280241, -12.22833218042435099, 1.218326283912148922 ) ) ;
#3114=CARTESIAN_POINT ( 'NONE',  ( 9.899494936611718643, -9.899494936611608509, 45.00000000000000711 ) ) ;
#3117=CARTESIAN_POINT ( 'NONE',  ( -5.420364854931999155, -15.49051278174644253, 46.07142857142856940 ) ) ;
#3121=CARTESIAN_POINT ( 'NONE',  ( -11.31370849898482156, 11.31370849898469544, 36.00000000000000711 ) ) ;
#3123=CARTESIAN_POINT ( 'NONE',  ( 11.22385875690717683, -11.40355824106234373, 31.00404056962644006 ) ) ;
#3125=CARTESIAN_POINT ( 'NONE',  ( -8.621071003556675549, 13.96533075980314642, 28.21832628391215181 ) ) ;
#3132=CARTESIAN_POINT ( 'NONE',  ( -1.837501619626328297, 16.30827793483733856, 18.64285714285715656 ) ) ;
#3134=CARTESIAN_POINT ( 'NONE',  ( 10.15407889436379030, 10.15407889436390221, 37.50000000000001421 ) ) ;
#3135=CARTESIAN_POINT ( 'NONE',  ( 13.17239914596754424, -4.743843029824685864, 36.57546914105501656 ) ) ;
#3139=CARTESIAN_POINT ( 'NONE',  ( 12.15899005565164792, -7.639999817571655250, 8.785714285714293581 ) ) ;
#3145=CARTESIAN_POINT ( 'NONE',  ( -15.44746603149413922, -5.543385399275820191, 30.92453085894499765 ) ) ;
#3147=CARTESIAN_POINT ( 'NONE',  ( 13.54758718765249803, 8.512513224245457977, 7.714285714285715301 ) ) ;
#3148=CARTESIAN_POINT ( 'NONE',  ( 1.967016585148662289, -16.29368510291087091, 17.63881657323070939 ) ) ;
#3155=( NAMED_UNIT ( * ) SI_UNIT ( $, .STERADIAN. ) SOLID_ANGLE_UNIT ( ) );
#3157=CARTESIAN_POINT ( 'NONE',  ( -13.51115193377584589, -4.865839792409295761, 12.92453085894499587 ) ) ;
#3159=CARTESIAN_POINT ( 'NONE',  ( 13.89598863503046111, -8.731428362939032795, 14.78571428571429358 ) ) ;
#3162=CARTESIAN_POINT ( 'NONE',  ( -13.25633410266679313, 4.503970704919840529, 31.56738800180213644 ) ) ;
#3166=CARTESIAN_POINT ( 'NONE',  ( 12.08964793087886314, -7.750357176954162597, 0.7897548553407187644 ) ) ;
#3168=CARTESIAN_POINT ( 'NONE',  ( 12.08964793087886314, -7.750357176954162597, 18.78975485534072121 ) ) ;
#3170=AXIS2_PLACEMENT_3D ( 'NONE', #6388, #8888, #9567 ) ;
#3171=CARTESIAN_POINT ( 'NONE',  ( 16.32287076676382043, -1.707986654103810897, 16.35310228751641759 ) ) ;
#3173=ADVANCED_FACE ( 'NONE', ( #3269 ), #5737, .F. ) ;
#3174=CARTESIAN_POINT ( 'NONE',  ( -5.284464991282755264, 15.10213328493384743, 42.42857142857143060 ) ) ;
#3179=CARTESIAN_POINT ( 'NONE',  ( -15.10213328493390961, 5.284464991282586510, 35.57142857142857650 ) ) ;
#3182=CARTESIAN_POINT ( 'NONE',  ( -15.91362231745475597, -1.665163862720028254, 39.14689771248358596 ) ) ;
#3184=CARTESIAN_POINT ( 'NONE',  ( 11.31370849898482334, -11.31370849898469366, 21.00000000000000355 ) ) ;
#3192=CARTESIAN_POINT ( 'NONE',  ( 8.884063115244108744, 10.93517402715751885, 47.39553751340654486 ) ) ;
#3193=CARTESIAN_POINT ( 'NONE',  ( 13.54758718765249803, 8.512513224245457977, 19.71428571428571175 ) ) ;
#3195=CARTESIAN_POINT ( 'NONE',  ( -13.91197093850538380, -1.567502665446387278, 35.14285714285713880 ) ) ;
#3197=CARTESIAN_POINT ( 'NONE',  ( -12.08964793087886314, 7.750357176954159932, 33.78975485534073897 ) ) ;
#3201=CARTESIAN_POINT ( 'NONE',  ( 8.684116361910502846, 11.09462624213450610, 51.38745637415366474 ) ) ;
#3205=CARTESIAN_POINT ( 'NONE',  ( 11.31370849898482334, -11.31370849898469366, 15.00000000000000000 ) ) ;
#3206=CARTESIAN_POINT ( 'NONE',  ( -8.404922754268618235, -13.61519076058357491, 18.28167371608785174 ) ) ;
#3212=CARTESIAN_POINT ( 'NONE',  ( 4.743843029824831525, -13.17239914596749095, 17.42453085894499409 ) ) ;
#3215=CARTESIAN_POINT ( 'NONE',  ( -10.06191849875405531, -10.24623928997363542, 24.49595943037356705 ) ) ;
#3219=CARTESIAN_POINT ( 'NONE',  ( -9.809645194534070356, 9.989344678689256796, 4.004040569626432067 ) ) ;
#3220=CARTESIAN_POINT ( 'NONE',  ( -4.865839792409144771, -13.51115193377589740, 14.07546914105500768 ) ) ;
#3223=CARTESIAN_POINT ( 'NONE',  ( -11.31370849898482156, 11.31370849898469544, 48.00000000000000000 ) ) ;
#3230=CARTESIAN_POINT ( 'NONE',  ( -15.06016580658428694, 5.404401153735006957, 39.57546914105500946 ) ) ;
#3232=CARTESIAN_POINT ( 'NONE',  ( -15.89939535829186923, -1.791431617653016062, 35.14285714285713880 ) ) ;
#3240=CARTESIAN_POINT ( 'NONE',  ( -11.92174236212692051, -7.340858601238089420, 44.71832628391215536 ) ) ;
#3241=CARTESIAN_POINT ( 'NONE',  ( 15.89939535829187278, 1.791431617653015174, 14.14285714285714413 ) ) ;
#3242=CARTESIAN_POINT ( 'NONE',  ( 7.639999817571788476, -12.15899005565156266, 39.21428571428571530 ) ) ;
#3243=CARTESIAN_POINT ( 'NONE',  ( -7.556039541191334585, -11.78653521626503320, 44.28975485534073186 ) ) ;
#3244=CARTESIAN_POINT ( 'NONE',  ( -12.15899005565164792, 7.639999817571651697, 5.785714285714282035 ) ) ;
#3248=CARTESIAN_POINT ( 'NONE',  ( -13.91197093850538380, -1.567502665446387278, 5.142857142857143238 ) ) ;
#3250=CARTESIAN_POINT ( 'NONE',  ( -11.31370849898482156, 11.31370849898469544, 18.00000000000000355 ) ) ;
#3251=CARTESIAN_POINT ( 'NONE',  ( 13.96533075980324234, -8.621071003556521006, 34.78167371608785885 ) ) ;
#3254=CARTESIAN_POINT ( 'NONE',  ( 11.85413878919593422, 7.448449071214774619, 1.714285714285716855 ) ) ;
#3257=CARTESIAN_POINT ( 'NONE',  ( 12.22833218042443271, -7.529642458189144349, 16.78167371608784819 ) ) ;
#3260=CARTESIAN_POINT ( 'NONE',  ( -1.441234910513241818, -13.92619789766829008, 41.85310228751642825 ) ) ;
#3265=CARTESIAN_POINT ( 'NONE',  ( 1.478298951650704351, -14.28433602490913579, 7.646897712483577969 ) ) ;
#3267=CARTESIAN_POINT ( 'NONE',  ( 12.08964793087886314, -7.750357176954162597, 6.789754855340717654 ) ) ;
#3269=FACE_OUTER_BOUND ( 'NONE', #2084, .T. ) ;
#3270=CARTESIAN_POINT ( 'NONE',  ( 11.31370849898482334, -11.31370849898469366, 39.00000000000000000 ) ) ;
#3276=CARTESIAN_POINT ( 'NONE',  ( 15.91362231745475597, 1.665163862720026255, 24.14689771248357530 ) ) ;
#3278=CARTESIAN_POINT ( 'NONE',  ( 11.69682198916835070, 11.51250119794901394, 35.50404056962644006 ) ) ;
#3280=CARTESIAN_POINT ( 'NONE',  ( 5.420364854932001819, 15.49051278174644430, 25.07142857142858361 ) ) ;
#3282=CARTESIAN_POINT ( 'NONE',  ( 13.54758718765249803, 8.512513224245457977, 1.714285714285716855 ) ) ;
#3284=( NAMED_UNIT ( * ) SI_UNIT ( $, .STERADIAN. ) SOLID_ANGLE_UNIT ( ) );
#3287=UNCERTAINTY_MEASURE_WITH_UNIT (LENGTH_MEASURE( 1.000000000000000082E-05 ), #7007, 'distance_accuracy_value', 'NONE');
#3288=CARTESIAN_POINT ( 'NONE',  ( 4.865839792409144771, 13.51115193377589740, 41.07546914105501656 ) ) ;
#3289=CARTESIAN_POINT ( 'NONE',  ( -8.512513224245306986, -13.54758718765259218, 22.28571428571428470 ) ) ;
#3290=CARTESIAN_POINT ( 'NONE',  ( 4.742819248065502258, 13.55419868402813499, 37.07142857142857650 ) ) ;
#3291=CARTESIAN_POINT ( 'NONE',  ( -11.92174236212692051, -7.340858601238089420, 38.71832628391214826 ) ) ;
#3293=CARTESIAN_POINT ( 'NONE',  ( -7.448449071214644945, -11.85413878919601771, 10.28571428571428648 ) ) ;
#3297=CARTESIAN_POINT ( 'NONE',  ( -13.25633410266679313, 4.503970704919840529, 49.56738800180214355 ) ) ;
#3302=CARTESIAN_POINT ( 'NONE',  ( -15.10213328493390961, 5.284464991282586510, 11.57142857142857295 ) ) ;
#3304=CARTESIAN_POINT ( 'NONE',  ( 8.841785722321695573, -13.82664651025757152, 35.21024514465927524 ) ) ;
#3312=CARTESIAN_POINT ( 'NONE',  ( -9.989344678689363377, 9.809645194533960222, 19.99595943037356349 ) ) ;
#3315=CARTESIAN_POINT ( 'NONE',  ( -1.737328882695368115, 14.25515036105620581, 38.63881657323070584 ) ) ;
#3322=CARTESIAN_POINT ( 'NONE',  ( 7.529642458189280241, -12.22833218042435099, 19.21832628391215181 ) ) ;
#3325=CARTESIAN_POINT ( 'NONE',  ( -13.17239914596754424, 4.743843029824683200, 9.575469141055007682 ) ) ;
#3328=CARTESIAN_POINT ( 'NONE',  ( 1.665163862719847732, 15.91362231745477374, 8.853102287516419366 ) ) ;
#3334=CARTESIAN_POINT ( 'NONE',  ( 1.707986654103998303, -16.32287076676380266, 31.64689771248358241 ) ) ;
#3336=CARTESIAN_POINT ( 'NONE',  ( -13.82664651025767100, 8.841785722321537477, 33.78975485534073897 ) ) ;
#3338=CARTESIAN_POINT ( 'NONE',  ( 13.54758718765249803, 8.512513224245457977, 31.71428571428571530 ) ) ;
#3341=CARTESIAN_POINT ( 'NONE',  ( -8.512513224245306986, -13.54758718765259218, 22.28571428571428470 ) ) ;
#3346=CARTESIAN_POINT ( 'NONE',  ( 11.69682198916835070, 11.51250119794901394, -0.4959594303735606058 ) ) ;
#3347=CARTESIAN_POINT ( 'NONE',  ( 5.284464991282756152, -15.10213328493384743, 15.42857142857143060 ) ) ;
#3348=CARTESIAN_POINT ( 'NONE',  ( -4.742819248065500481, -13.55419868402813499, 46.07142857142857650 ) ) ;
#3349=CARTESIAN_POINT ( 'NONE',  ( 13.17239914596754424, -4.743843029824685864, 36.57546914105501656 ) ) ;
#3350=CARTESIAN_POINT ( 'NONE',  ( 13.91197093850538380, 1.567502665446386390, 14.14285714285714413 ) ) ;
#3354=CARTESIAN_POINT ( 'NONE',  ( 13.55419868402807992, 4.742819248065648807, 7.928571428571430602 ) ) ;
#3357=CARTESIAN_POINT ( 'NONE',  ( -15.89939535829186923, -1.791431617653016062, 11.14285714285714235 ) ) ;
#3358=CARTESIAN_POINT ( 'NONE',  ( -1.665163862719845067, -15.91362231745477374, 35.85310228751641404 ) ) ;
#3361=CARTESIAN_POINT ( 'NONE',  ( -1.567502665446231180, -13.91197093850540334, 3.857142857142857650 ) ) ;
#3362=CARTESIAN_POINT ( 'NONE',  ( 13.25633410266679313, -4.503970704919842305, 16.56738800180213289 ) ) ;
#3364=CARTESIAN_POINT ( 'NONE',  ( -13.54758718765249625, -8.512513224245459753, 16.71428571428571530 ) ) ;
#3366=CARTESIAN_POINT ( 'NONE',  ( -13.89774397934249706, -1.693770420379375974, 43.13881657323070584 ) ) ;
#3371=CARTESIAN_POINT ( 'NONE',  ( 11.92174236212692229, 7.340858601238088532, 23.71832628391215181 ) ) ;
#3373=CARTESIAN_POINT ( 'NONE',  ( -1.478298951650703019, 14.28433602490913579, 16.64689771248358596 ) ) ;
#3375=CARTESIAN_POINT ( 'NONE',  ( -0.3021515714675195863, 13.99673906407701729, 48.73000000000003951 ) ) ;
#3376=CARTESIAN_POINT ( 'NONE',  ( 13.47998361472151529, 8.620103694222146729, 15.71024514465927879 ) ) ;
#3382=CARTESIAN_POINT ( 'NONE',  ( -15.91362231745475597, -1.665163862720028254, 39.14689771248358596 ) ) ;
#3383=CARTESIAN_POINT ( 'NONE',  ( 10.15407889436379030, 10.15407889436390576, 31.50000000000001421 ) ) ;
#3384=CARTESIAN_POINT ( 'NONE',  ( 11.69682198916835070, 11.51250119794901394, 41.50404056962644006 ) ) ;
#3386=CARTESIAN_POINT ( 'NONE',  ( 16.30827793483735633, -1.837501619626142890, 32.35714285714286120 ) ) ;
#3388=CARTESIAN_POINT ( 'NONE',  ( 11.60466159355862104, 11.60466159355875071, 13.50000000000000178 ) ) ;
#3389=PLANE ( 'NONE',  #9926 ) ;
#3392=CARTESIAN_POINT ( 'NONE',  ( 15.06016580658428694, -5.404401153735007846, 0.5754691410550027975 ) ) ;
#3393=CARTESIAN_POINT ( 'NONE',  ( -8.512513224245306986, -13.54758718765259218, 34.28571428571428470 ) ) ;
#3395=CARTESIAN_POINT ( 'NONE',  ( 1.478298951650704351, -14.28433602490913579, 43.64689771248358596 ) ) ;
#3396=CARTESIAN_POINT ( 'NONE',  ( -4.742819248065502258, -13.55419868402813677, 10.07142857142856940 ) ) ;
#3400=CARTESIAN_POINT ( 'NONE',  ( -7.448449071214644945, -11.85413878919601771, 22.28571428571428470 ) ) ;
#3403=CARTESIAN_POINT ( 'NONE',  ( -11.60466159355861748, -11.60466159355874893, 16.50000000000000000 ) ) ;
#3404=CARTESIAN_POINT ( 'NONE',  ( -8.841785722321695573, 13.82664651025757152, 32.21024514465928235 ) ) ;
#3407=CARTESIAN_POINT ( 'NONE',  ( 12.15899005565164792, -7.639999817571654361, 8.785714285714290028 ) ) ;
#3409=CARTESIAN_POINT ( 'NONE',  ( 14.28433602490915000, -1.478298951650544479, 22.35310228751642114 ) ) ;
#3412=CARTESIAN_POINT ( 'NONE',  ( 13.25633410266679313, -4.503970704919842305, 34.56738800180213644 ) ) ;
#3417=CARTESIAN_POINT ( 'NONE',  ( 4.503970704919991519, -13.25633410266674517, 25.43261199819786711 ) ) ;
#3420=CARTESIAN_POINT ( 'NONE',  ( -11.51250119794888072, -11.69682198916848037, 6.495959430373559051 ) ) ;
#3426=CARTESIAN_POINT ( 'NONE',  ( 15.91362231745475597, 1.665163862720026255, 36.14689771248357886 ) ) ;
#3427=CARTESIAN_POINT ( 'NONE',  ( 1.567502665446232957, 13.91197093850540156, 24.85714285714285765 ) ) ;
#3428=CARTESIAN_POINT ( 'NONE',  ( -1.607813917173034124, 14.26974319298267524, 42.64285714285715301 ) ) ;
#3430=CARTESIAN_POINT ( 'NONE',  ( -15.10213328493390961, 5.284464991282586510, 29.57142857142857650 ) ) ;
#3432=CARTESIAN_POINT ( 'NONE',  ( -11.60466159355861926, -11.60466159355875249, 16.50000000000000000 ) ) ;
#3437=CARTESIAN_POINT ( 'NONE',  ( -5.164528828830334817, 15.14410076328347543, 16.43261199819786356 ) ) ;
#3438=CARTESIAN_POINT ( 'NONE',  ( -15.10213328493390961, 5.284464991282586510, 29.57142857142857650 ) ) ;
#3439=CARTESIAN_POINT ( 'NONE',  ( 15.91362231745475597, 1.665163862720026255, 0.1468977124835755543 ) ) ;
#3440=CARTESIAN_POINT ( 'NONE',  ( -1.607813917173034124, 14.26974319298267524, 6.642857142857143238 ) ) ;
#3444=CARTESIAN_POINT ( 'NONE',  ( -1.567502665446231180, -13.91197093850540334, 21.85714285714286120 ) ) ;
#3446=CARTESIAN_POINT ( 'NONE',  ( 15.10213328493390783, -5.284464991282587398, 32.57142857142856940 ) ) ;
#3447=CARTESIAN_POINT ( 'NONE',  ( -5.297344310588352201, -15.53355953199867301, 36.06738800180213644 ) ) ;
#3449=CARTESIAN_POINT ( 'NONE',  ( 1.607813917173037899, -14.26974319298267169, 15.64285714285714235 ) ) ;
#3452=CARTESIAN_POINT ( 'NONE',  ( -13.89774397934249706, -1.693770420379375974, 31.13881657323070939 ) ) ;
#3455=CARTESIAN_POINT ( 'NONE',  ( 10.19143222367002366, 10.12210786732603474, 48.73000000000001819 ) ) ;
#3456=CARTESIAN_POINT ( 'NONE',  ( -10.06191849875405531, -10.24623928997363542, 36.49595943037355994 ) ) ;
#3459=EDGE_CURVE ( 'NONE', #6853, #7160, #7021, .T. ) ;
#3461=CARTESIAN_POINT ( 'NONE',  ( -4.865839792409144771, -13.51115193377589740, 20.07546914105500591 ) ) ;
#3465=CARTESIAN_POINT ( 'NONE',  ( -1.478298951650703019, 14.28433602490913579, 22.64689771248357530 ) ) ;
#3467=CARTESIAN_POINT ( 'NONE',  ( -15.14410076328353227, 5.164528828830164287, 43.56738800180213644 ) ) ;
#3469=CARTESIAN_POINT ( 'NONE',  ( -11.25886268110355992, 10.92057193546596494, 48.72999999999974108 ) ) ;
#3470=CARTESIAN_POINT ( 'NONE',  ( -15.88516839912898071, -1.917699372586004980, 7.138816573230711171 ) ) ;
#3480=CARTESIAN_POINT ( 'NONE',  ( 5.164528828830335705, -15.14410076328347543, 37.43261199819787066 ) ) ;
#3481=CARTESIAN_POINT ( 'NONE',  ( -12.15899005565164792, 7.639999817571651697, 29.78571428571428825 ) ) ;
#3484=CARTESIAN_POINT ( 'NONE',  ( -13.91197093850538380, -1.567502665446387278, 41.14285714285714590 ) ) ;
#3487=CARTESIAN_POINT ( 'NONE',  ( -5.420364854931999155, -15.49051278174644253, 40.07142857142857650 ) ) ;
#3489=CARTESIAN_POINT ( 'NONE',  ( 8.512513224245308763, 13.54758718765259040, 13.28571428571429003 ) ) ;
#3495=CARTESIAN_POINT ( 'NONE',  ( 8.621071003556677326, -13.96533075980314287, 7.218326283912148256 ) ) ;
#3496=CARTESIAN_POINT ( 'NONE',  ( 1.791431617652837316, 15.89939535829188877, 24.85714285714285765 ) ) ;
#3497=CARTESIAN_POINT ( 'NONE',  ( 15.91362231745475597, 1.665163862720026255, 6.146897712483580634 ) ) ;
#3498=( BOUNDED_CURVE ( )  B_SPLINE_CURVE ( 2, ( #7707, #628, #1403, #6080, #731, #2327, #7071, #7022, #1558, #3927, #6233, #3776, #4704, #1502, #4502, #2994, #777, #8528, #6856, #680, #6908, #6137, #7654, #2180, #9313, #7852, #3719, #4604, #2226, #6186, #9362, #5372, #3829, #6967, #3879, #10129, #3147, #3045, #2274, #5421, #8578, #10028, #5476, #4655, #10180, #6287, #3096, #9472, #6236, #9413, #5260, #1709, #3357, #9568, #3302, #4182, #1654, #7332, #982, #4855, #7283, #255, #1802, #46, #7955, #2425, #9670, #6492, #207, #933, #3205, #6339, #2578, #2471, #7131, #4078, #96, #3403, #8844, #6538, #5525, #9519, #5721, #8791, #3250, #4757, #6444, #5571, #148, #7228, #6390, #2374, #8684, #4804, #5625, #1606, #8890, #7901, #8734, #4956, #4130, #884, #4035, #4906, #8109, #825, #1038, #3982, #7180, #8003, #9624, #2526, #1755, #5676, #8052, #5208, #2722, #1087, #1953, #7583, #2825, #8943, #7428, #3654, #2622, #5970, #359, #8310, #5160, #5006, #9718, #9771, #5767, #409, #6731, #9919, #6636, #3599, #9148, #7379, #4437, #2055, #8358, #8153, #1278, #506, #1856, #2674, #4228, #5917, #305, #4278, #3446, #5865, #6586, #5102, #5820, #8997, #1906, #5055, #3553, #8201, #1133, #3506, #1231, #4382, #9820, #9043, #8252, #1181, #6681, #4330, #7481, #9865, #2770, #9091, #2006, #7533, #460, #4639, #2259, #1543, #4689, #7696, #9197, #560, #6069, #10166, #6018, #2977, #9243, #7746, #665, #6896, #10064, #9301, #5407, #2215, #3081, #6126, #5361, #6224, #10014, #8406, #7006, #2161, #8515, #7837, #1439, #5459, #6174, #4592, #1389, #3816, #7798, #3762, #6953, #8621, #5307, #764, #8564, #1488, #8464, #718, #3865, #4542, #615, #10118, #9401 ),
 .UNSPECIFIED., .F., .F. ) 
 B_SPLINE_CURVE_WITH_KNOTS ( ( 3, 2, 2, 2, 2, 2, 2, 2, 2, 2, 2, 2, 2, 2, 2, 2, 2, 2, 2, 2, 2, 2, 2, 2, 2, 2, 2, 2, 2, 2, 2, 2, 2, 2, 2, 2, 2, 2, 2, 2, 2, 2, 2, 2, 2, 2, 2, 2, 2, 2, 2, 2, 2, 2, 2, 2, 2, 2, 2, 2, 2, 2, 2, 2, 2, 2, 2, 2, 2, 2, 2, 2, 2, 2, 2, 2, 2, 2, 2, 2, 2, 2, 2, 2, 2, 2, 2, 2, 2, 2, 2, 2, 2, 2, 2, 2, 2, 2, 2, 2, 2, 2, 2, 2, 2, 2, 2, 2, 2, 2, 2, 2, 2, 2, 3 ),
 ( 0.000000000000000000, 0.007936507936507936067, 0.01587301587301587213, 0.02380952380952380820, 0.03174603174603174427, 0.03968253968253968728, 0.04761904761904761640, 0.05555555555555555247, 0.06349206349206348854, 0.07142857142857142461, 0.07936507936507937455, 0.08730158730158729674, 0.09523809523809523281, 0.1031746031746031828, 0.1111111111111111049, 0.1190476190476190410, 0.1269841269841269771, 0.1349206349206349131, 0.1428571428571428492, 0.1507936507936507853, 0.1587301587301587491, 0.1666666666666666574, 0.1746031746031745935, 0.1825396825396825295, 0.1904761904761904656, 0.1984126984126984017, 0.2063492063492063655, 0.2142857142857142738, 0.2222222222222222099, 0.2301587301587301460, 0.2380952380952380820, 0.2460317460317460181, 0.2539682539682539542, 0.2619047619047619180, 0.2698412698412698263, 0.2777777777777777901, 0.2857142857142856984, 0.2936507936507936622, 0.3015873015873015706, 0.3095238095238095344, 0.3174603174603174982, 0.3253968253968254065, 0.3333333333333333148, 0.3412698412698412787, 0.3492063492063491870, 0.3571428571428571508, 0.3650793650793650591, 0.3730158730158730229, 0.3809523809523809312, 0.3888888888888888951, 0.3968253968253968034, 0.4047619047619047672, 0.4126984126984127310, 0.4206349206349206393, 0.4285714285714285476, 0.4365079365079365115, 0.4444444444444444198, 0.4523809523809524391, 0.4603174603174602919, 0.4682539682539682557, 0.4761904761904761640, 0.4841269841269841279, 0.4920634920634920362, 0.5000000000000000000, 0.5079365079365079083, 0.5158730158730159276, 0.5238095238095238360, 0.5317460317460317443, 0.5396825396825396526, 0.5476190476190476719, 0.5555555555555555802, 0.5634920634920634885, 0.5714285714285713969, 0.5793650793650794162, 0.5873015873015873245, 0.5952380952380951218, 0.6031746031746031411, 0.6111111111111111605, 0.6190476190476190688, 0.6269841269841269771, 0.6349206349206349964, 0.6428571428571429047, 0.6507936507936508130, 0.6587301587301587213, 0.6666666666666666297, 0.6746031746031745380, 0.6825396825396825573, 0.6904761904761904656, 0.6984126984126983739, 0.7063492063492063933, 0.7142857142857143016, 0.7222222222222222099, 0.7301587301587301182, 0.7380952380952381375, 0.7460317460317460458, 0.7539682539682539542, 0.7619047619047618625, 0.7698412698412698818, 0.7777777777777777901, 0.7857142857142856984, 0.7936507936507936067, 0.8015873015873016261, 0.8095238095238095344, 0.8174603174603174427, 0.8253968253968254620, 0.8333333333333333703, 0.8412698412698412787, 0.8492063492063491870, 0.8571428571428570953, 0.8650793650793650036, 0.8730158730158730229, 0.8809523809523809312, 0.8888888888888888395, 0.8968253968253968589, 0.9023904529665212060 ),
 .UNSPECIFIED. ) 
 CURVE ( )  GEOMETRIC_REPRESENTATION_ITEM ( )  RATIONAL_B_SPLINE_CURVE ( ( 1.000000000000000000, 0.9749279121818236193, 1.000000000000000000, 0.9749279121818236193, 1.000000000000000000, 0.9749279121818236193, 1.000000000000000000, 0.9749279121818236193, 1.000000000000000000, 0.9749279121818236193, 1.000000000000000000, 0.9749279121818236193, 1.000000000000000000, 0.9749279121818236193, 1.000000000000000000, 0.9749279121818236193, 1.000000000000000000, 0.9749279121818236193, 1.000000000000000000, 0.9749279121818236193, 1.000000000000000000, 0.9749279121818236193, 1.000000000000000000, 0.9749279121818236193, 1.000000000000000000, 0.9749279121818236193, 1.000000000000000000, 0.9749279121818236193, 1.000000000000000000, 0.9749279121818236193, 1.000000000000000000, 0.9749279121818236193, 1.000000000000000000, 0.9749279121818236193, 1.000000000000000000, 0.9749279121818236193, 1.000000000000000000, 0.9749279121818236193, 1.000000000000000000, 0.9749279121818236193, 1.000000000000000000, 0.9749279121818236193, 1.000000000000000000, 0.9749279121818236193, 1.000000000000000000, 0.9749279121818236193, 1.000000000000000000, 0.9749279121818236193, 1.000000000000000000, 0.9749279121818236193, 1.000000000000000000, 0.9749279121818236193, 1.000000000000000000, 0.9749279121818236193, 1.000000000000000000, 0.9749279121818236193, 1.000000000000000000, 0.9749279121818236193, 1.000000000000000000, 0.9749279121818236193, 1.000000000000000000, 0.9749279121818236193, 1.000000000000000000, 0.9749279121818236193, 1.000000000000000000, 0.9749279121818236193, 1.000000000000000000, 0.9749279121818236193, 1.000000000000000000, 0.9749279121818236193, 1.000000000000000000, 0.9749279121818236193, 1.000000000000000000, 0.9749279121818236193, 1.000000000000000000, 0.9749279121818236193, 1.000000000000000000, 0.9749279121818236193, 1.000000000000000000, 0.9749279121818236193, 1.000000000000000000, 0.9749279121818236193, 1.000000000000000000, 0.9749279121818236193, 1.000000000000000000, 0.9749279121818236193, 1.000000000000000000, 0.9749279121818236193, 1.000000000000000000, 0.9749279121818236193, 1.000000000000000000, 0.9749279121818236193, 1.000000000000000000, 0.9749279121818236193, 1.000000000000000000, 0.9749279121818236193, 1.000000000000000000, 0.9749279121818236193, 1.000000000000000000, 0.9749279121818236193, 1.000000000000000000, 0.9749279121818236193, 1.000000000000000000, 0.9749279121818236193, 1.000000000000000000, 0.9749279121818236193, 1.000000000000000000, 0.9749279121818236193, 1.000000000000000000, 0.9749279121818236193, 1.000000000000000000, 0.9749279121818236193, 1.000000000000000000, 0.9749279121818236193, 1.000000000000000000, 0.9749279121818236193, 1.000000000000000000, 0.9749279121818236193, 1.000000000000000000, 0.9749279121818236193, 1.000000000000000000, 0.9749279121818236193, 1.000000000000000000, 0.9749279121818236193, 1.000000000000000000, 0.9749279121818236193, 1.000000000000000000, 0.9749279121818236193, 1.000000000000000000, 0.9749279121818236193, 1.000000000000000000, 0.9749279121818236193, 1.000000000000000000, 0.9749279121818236193, 1.000000000000000000, 0.9749279121818236193, 1.000000000000000000, 0.9749279121818236193, 1.000000000000000000, 0.9749279121818236193, 1.000000000000000000, 0.9749279121818236193, 1.000000000000000000, 0.9749279121818236193, 1.000000000000000000, 0.9749279121818236193, 1.000000000000000000, 0.9749279121818236193, 1.000000000000000000, 0.9749279121818236193, 1.000000000000000000, 0.9749279121818236193, 1.000000000000000000, 0.9749279121818236193, 1.000000000000000000, 0.9749279121818236193, 1.000000000000000000, 0.9749279121818236193, 1.000000000000000000, 0.9749279121818236193, 1.000000000000000000, 0.9749279121818236193, 1.000000000000000000, 0.9749279121818236193, 1.000000000000000000, 0.9749279121818236193, 1.000000000000000000, 0.9749279121818236193, 1.000000000000000000, 0.9749279121818236193, 1.000000000000000000, 0.9749279121818236193, 1.000000000000000000, 0.9749279121818236193, 1.000000000000000000, 0.9749279121818236193, 1.000000000000000000, 0.9749279121818236193, 1.000000000000000000, 0.9749279121818236193, 1.000000000000000000, 0.9749279121818236193, 1.000000000000000000, 0.9749279121818236193, 1.000000000000000000, 0.9749279121818236193, 1.000000000000000000, 0.9749279121818236193, 1.000000000000000000, 0.9749279121818236193, 1.000000000000000000, 0.9749279121818236193, 1.000000000000000000, 0.9749279121818236193, 1.000000000000000000, 0.9749279121818236193, 1.000000000000000000, 0.9749279121818236193, 1.000000000000000000, 0.9749279121818236193, 1.000000000000000000, 0.9749279121818236193, 1.000000000000000000, 0.9749279121818236193, 1.000000000000000000, 0.9749279121818236193, 1.000000000000000000, 0.9749279121818236193, 1.000000000000000000, 0.9749279121818236193, 1.000000000000000000, 0.9749279121818236193, 1.000000000000000000, 0.9749279121818236193, 1.000000000000000000, 0.9749279121818236193, 1.000000000000000000, 0.9749279121818236193, 1.000000000000000000, 0.9749279121818236193, 1.000000000000000000, 0.9749279121818236193, 1.000000000000000000, 0.9749279121818236193, 1.000000000000000000, 0.9749279121818236193, 1.000000000000000000, 0.9824195253882976875, 0.9894938054834325758 ) ) 
 REPRESENTATION_ITEM ( '' )  );
#3499=CARTESIAN_POINT ( 'NONE',  ( 7.448449071214646722, 11.85413878919601594, 25.28571428571428470 ) ) ;
#3500=CARTESIAN_POINT ( 'NONE',  ( 11.31370849898482334, -11.31370849898469366, 9.000000000000001776 ) ) ;
#3503=CARTESIAN_POINT ( 'NONE',  ( -14.26974319298268767, 1.607813917172874918, 11.35714285714285943 ) ) ;
#3506=CARTESIAN_POINT ( 'NONE',  ( -15.49051278174637858, -5.420364854932175014, 34.92857142857143771 ) ) ;
#3507=CARTESIAN_POINT ( 'NONE',  ( 13.25633410266679313, -4.503970704919842305, 4.567388001802134667 ) ) ;
#3510=CARTESIAN_POINT ( 'NONE',  ( -13.91197093850538380, -1.567502665446387278, 5.142857142857143238 ) ) ;
#3512=CARTESIAN_POINT ( 'NONE',  ( 13.51115193377584589, 4.865839792409294873, 33.92453085894499054 ) ) ;
#3518=CARTESIAN_POINT ( 'NONE',  ( 4.619798703721856192, 13.59724543428036725, 51.06738800180214355 ) ) ;
#3523=CARTESIAN_POINT ( 'NONE',  ( -13.92619789766827054, -1.441234910513399470, 15.14689771248357708 ) ) ;
#3526=CARTESIAN_POINT ( 'NONE',  ( 13.92619789766827587, 1.441234910513398582, 24.14689771248357530 ) ) ;
#3528=CARTESIAN_POINT ( 'NONE',  ( 1.665163862719847732, 15.91362231745477374, 32.85310228751642114 ) ) ;
#3529=CARTESIAN_POINT ( 'NONE',  ( -12.86099432095302575, 7.347572223948011683, 48.73000000000000398 ) ) ;
#3530=CARTESIAN_POINT ( 'NONE',  ( -15.49051278174638036, -5.420364854932175902, 22.92857142857142705 ) ) ;
#3536=CARTESIAN_POINT ( 'NONE',  ( -4.623906867372410190, 13.21436662431711895, 24.42857142857143060 ) ) ;
#3537=CARTESIAN_POINT ( 'NONE',  ( 7.639999817571789364, -12.15899005565156266, 39.21428571428571530 ) ) ;
#3539=CARTESIAN_POINT ( 'NONE',  ( -11.31370849898482156, 11.31370849898469544, 48.00000000000000000 ) ) ;
#3541=CARTESIAN_POINT ( 'NONE',  ( 15.49051278174638036, 5.420364854932175014, 13.92857142857143238 ) ) ;
#3544=CARTESIAN_POINT ( 'NONE',  ( 5.164528828830335705, -15.14410076328347543, 7.432611998197861780 ) ) ;
#3545=CARTESIAN_POINT ( 'NONE',  ( -15.89939535829186923, -1.791431617653016062, 23.14285714285714590 ) ) ;
#3546=CARTESIAN_POINT ( 'NONE',  ( 8.620103694221997515, 13.47998361472160767, 11.28975485534071943 ) ) ;
#3547=CARTESIAN_POINT ( 'NONE',  ( 11.85413878919593422, 7.448449071214774619, 25.71428571428571885 ) ) ;
#3551=CARTESIAN_POINT ( 'NONE',  ( 11.85413878919593422, 7.448449071214774619, 13.71428571428571352 ) ) ;
#3553=CARTESIAN_POINT ( 'NONE',  ( -8.512513224245306986, -13.54758718765259218, 34.28571428571428470 ) ) ;
#3554=CARTESIAN_POINT ( 'NONE',  ( -13.51115193377584589, -4.865839792409295761, 6.924530858944994982 ) ) ;
#3557=CARTESIAN_POINT ( 'NONE',  ( -11.85413878919593422, -7.448449071214776396, 4.714285714285712636 ) ) ;
#3559=CARTESIAN_POINT ( 'NONE',  ( 1.441234910513245149, 13.92619789766829008, 20.85310228751641759 ) ) ;
#3562=CARTESIAN_POINT ( 'NONE',  ( 13.21436662431716869, -4.623906867372263640, 2.571428571428571619 ) ) ;
#3566=CARTESIAN_POINT ( 'NONE',  ( 1.478298951650704351, -14.28433602490913579, 31.64689771248358241 ) ) ;
#3569=CARTESIAN_POINT ( 'NONE',  ( -13.17001005284346249, 7.209383666200358753, 48.73000000000002530 ) ) ;
#3571=CARTESIAN_POINT ( 'NONE',  ( 1.737328882695370558, -14.25515036105620581, 11.63881657323070939 ) ) ;
#3575=CARTESIAN_POINT ( 'NONE',  ( -5.543385399275643444, -15.44746603149420494, 38.07546914105502367 ) ) ;
#3576=CARTESIAN_POINT ( 'NONE',  ( -11.85413878919593422, -7.448449071214776396, 46.71428571428571530 ) ) ;
#3579=CARTESIAN_POINT ( 'NONE',  ( 14.26974319298268767, -1.607813917172876916, 44.35714285714287541 ) ) ;
#3581=CARTESIAN_POINT ( 'NONE',  ( 5.284464991282756152, -15.10213328493384743, 45.42857142857143060 ) ) ;
#3582=CARTESIAN_POINT ( 'NONE',  ( -4.920110265629110025, 15.11696251504478106, 1.442806492371169420E-14 ) ) ;
#3583=CARTESIAN_POINT ( 'NONE',  ( 13.54758718765249803, 8.512513224245457977, 31.71428571428571530 ) ) ;
#3589=CARTESIAN_POINT ( 'NONE',  ( 1.707986654103998303, -16.32287076676380266, 7.646897712483577969 ) ) ;
#3590=CARTESIAN_POINT ( 'NONE',  ( -13.89598863503046111, 8.731428362939027465, 23.78571428571429536 ) ) ;
#3592=CARTESIAN_POINT ( 'NONE',  ( -11.22385875690717327, 11.40355824106234550, 4.004040569626432067 ) ) ;
#3593=CARTESIAN_POINT ( 'NONE',  ( 1.567502665446232957, 13.91197093850540156, 18.85714285714285765 ) ) ;
#3594=CARTESIAN_POINT ( 'NONE',  ( -11.31370849898482156, 11.31370849898469544, 0.000000000000000000 ) ) ;
#3595=CARTESIAN_POINT ( 'NONE',  ( -13.54758718765249625, -8.512513224245459753, 40.71428571428571530 ) ) ;
#3597=CARTESIAN_POINT ( 'NONE',  ( 7.639999817571789364, -12.15899005565156266, 15.21428571428571530 ) ) ;
#3599=CARTESIAN_POINT ( 'NONE',  ( -16.30827793483735988, 1.837501619626141558, 29.35714285714286120 ) ) ;
#3600=CARTESIAN_POINT ( 'NONE',  ( -1.665163862719845067, -15.91362231745477374, 47.85310228751642114 ) ) ;
#3603=CARTESIAN_POINT ( 'NONE',  ( -4.742819248065500481, -13.55419868402813499, 10.07142857142856940 ) ) ;
#3606=CARTESIAN_POINT ( 'NONE',  ( 13.51115193377584589, 4.865839792409294873, 27.92453085894499054 ) ) ;
#3614=CARTESIAN_POINT ( 'NONE',  ( -13.59724543428031573, -4.619798703722008959, 26.93261199819786356 ) ) ;
#3616=CARTESIAN_POINT ( 'NONE',  ( 15.44746603149413922, 5.543385399275817527, 33.92453085894499054 ) ) ;
#3617=CARTESIAN_POINT ( 'NONE',  ( -8.994172837283734623, 11.03823571387622415, 48.73000000000002530 ) ) ;
#3618=CARTESIAN_POINT ( 'NONE',  ( 5.284464991282756152, -15.10213328493384743, 21.42857142857142705 ) ) ;
#3620=CARTESIAN_POINT ( 'NONE',  ( 7.750357176954296712, -12.08964793087877787, 17.21024514465927879 ) ) ;
#3625=CARTESIAN_POINT ( 'NONE',  ( -1.478298951650703019, 14.28433602490913579, -1.353102287516420921 ) ) ;
#3627=CARTESIAN_POINT ( 'NONE',  ( -11.85413878919593422, -7.448449071214776396, 40.71428571428571530 ) ) ;
#3631=CARTESIAN_POINT ( 'NONE',  ( -13.54758718765249625, -8.512513224245459753, 40.71428571428571530 ) ) ;
#3633=CARTESIAN_POINT ( 'NONE',  ( -2.358840667064915575, 15.62261993150980111, 1.394172777290095379E-15 ) ) ;
#3635=CARTESIAN_POINT ( 'NONE',  ( 1.791431617652837316, 15.89939535829188877, 24.85714285714285765 ) ) ;
#3641=CARTESIAN_POINT ( 'NONE',  ( 8.621071003556677326, -13.96533075980314287, 13.21832628391215181 ) ) ;
#3642=CARTESIAN_POINT ( 'NONE',  ( 16.30827793483735633, -1.837501619626142890, 44.35714285714287541 ) ) ;
#3645=CARTESIAN_POINT ( 'NONE',  ( -16.29368510291090288, 1.967016585148476215, 9.361183426769292382 ) ) ;
#3647=CARTESIAN_POINT ( 'NONE',  ( 12.15899005565164792, -7.639999817571655250, 20.78571428571429180 ) ) ;
#3648=CARTESIAN_POINT ( 'NONE',  ( -8.512513224245306986, -13.54758718765259218, 10.28571428571428648 ) ) ;
#3649=CARTESIAN_POINT ( 'NONE',  ( 10.03895970123120307, 12.58845729673829972, 49.39149694378009769 ) ) ;
#3654=CARTESIAN_POINT ( 'NONE',  ( 16.30827793483735633, -1.837501619626142890, 26.35714285714286120 ) ) ;
#3655=CARTESIAN_POINT ( 'NONE',  ( -11.51250119794888072, -11.69682198916848037, 48.49595943037355994 ) ) ;
#3657=CARTESIAN_POINT ( 'NONE',  ( 5.284464991282756152, -15.10213328493384743, 3.428571428571426605 ) ) ;
#3659=CARTESIAN_POINT ( 'NONE',  ( 13.55419868402807992, 4.742819248065649695, 31.92857142857143060 ) ) ;
#3662=CARTESIAN_POINT ( 'NONE',  ( -4.743843029824828861, 13.17239914596749450, 44.42453085894499765 ) ) ;
#3665=CARTESIAN_POINT ( 'NONE',  ( 16.32287076676382043, -1.707986654103810897, 4.353102287516421143 ) ) ;
#3666=CARTESIAN_POINT ( 'NONE',  ( 9.826155085340783302, 10.43469318297800896, 48.73000000000001819 ) ) ;
#3670=CARTESIAN_POINT ( 'NONE',  ( -13.89774397934249706, -1.693770420379375974, 49.13881657323070584 ) ) ;
#3674=CARTESIAN_POINT ( 'NONE',  ( -4.865839792409144771, -13.51115193377589740, 32.07546914105502367 ) ) ;
#3678=CARTESIAN_POINT ( 'NONE',  ( 15.14410076328353227, -5.164528828830166063, 40.56738800180214355 ) ) ;
#3679=CARTESIAN_POINT ( 'NONE',  ( -6.723343338700901839, 12.41960368482901700, 48.73000000000001819 ) ) ;
#3680=CARTESIAN_POINT ( 'NONE',  ( 1.837501619626330074, -16.30827793483733501, 27.64285714285714590 ) ) ;
#3682=CARTESIAN_POINT ( 'NONE',  ( -14.28433602490915000, 1.478298951650542481, 19.35310228751642825 ) ) ;
#3686=CARTESIAN_POINT ( 'NONE',  ( 8.620103694221997515, 13.47998361472160767, 41.28975485534072476 ) ) ;
#3687=CARTESIAN_POINT ( 'NONE',  ( -13.21436662431716869, 4.623906867372262752, 47.57142857142857650 ) ) ;
#3688=CARTESIAN_POINT ( 'NONE',  ( 1.478298951650704351, -14.28433602490913579, 1.646897712483578857 ) ) ;
#3690=CARTESIAN_POINT ( 'NONE',  ( 8.731428362939190890, -13.89598863503036164, 45.21428571428572951 ) ) ;
#3692=CARTESIAN_POINT ( 'NONE',  ( 15.49051278174638036, 5.420364854932175014, 31.92857142857143415 ) ) ;
#3698=CARTESIAN_POINT ( 'NONE',  ( 11.69682198916835070, 11.51250119794901394, 17.50404056962643651 ) ) ;
#3699=CARTESIAN_POINT ( 'NONE',  ( -15.10213328493390961, 5.284464991282586510, 47.57142857142857650 ) ) ;
#3702=CARTESIAN_POINT ( 'NONE',  ( 1.917699372585825790, 15.88516839912900203, 16.86118342676929061 ) ) ;
#3703=CARTESIAN_POINT ( 'NONE',  ( -9.899494936611716867, 9.899494936611610285, 24.00000000000000000 ) ) ;
#3704=CARTESIAN_POINT ( 'NONE',  ( 15.89939535829187278, 1.791431617653015174, 8.142857142857145902 ) ) ;
#3705=CARTESIAN_POINT ( 'NONE',  ( 8.731428362939190890, -13.89598863503036164, 45.21428571428572951 ) ) ;
#3710=CARTESIAN_POINT ( 'NONE',  ( 13.47998361472151529, 8.620103694222146729, 45.71024514465928235 ) ) ;
#3712=CARTESIAN_POINT ( 'NONE',  ( -5.420364854931999155, -15.49051278174644253, 4.071428571428569398 ) ) ;
#3713=CARTESIAN_POINT ( 'NONE',  ( -14.26974319298268767, 1.607813917172874696, 23.35714285714286120 ) ) ;
#3715=CARTESIAN_POINT ( 'NONE',  ( 14.28433602490915000, -1.478298951650544479, 46.35310228751641404 ) ) ;
#3718=CARTESIAN_POINT ( 'NONE',  ( 8.841785722321695573, -13.82664651025757152, 29.21024514465927879 ) ) ;
#3719=CARTESIAN_POINT ( 'NONE',  ( -15.10213328493390961, 5.284464991282586510, 5.571428571428574728 ) ) ;
#3721=CARTESIAN_POINT ( 'NONE',  ( 8.684116361910502846, 11.09462624213450610, 51.38745637415366474 ) ) ;
#3725=CARTESIAN_POINT ( 'NONE',  ( -7.556039541191334585, -11.78653521626503320, 32.28975485534072476 ) ) ;
#3728=CARTESIAN_POINT ( 'NONE',  ( -15.44746603149413922, -5.543385399275820191, 48.92453085894499054 ) ) ;
#3730=CARTESIAN_POINT ( 'NONE',  ( -15.49051278174638036, -5.420364854932175902, 28.92857142857143771 ) ) ;
#3732=CARTESIAN_POINT ( 'NONE',  ( 1.441234910513245149, 13.92619789766829008, 20.85310228751641759 ) ) ;
#3736=CARTESIAN_POINT ( 'NONE',  ( 11.22385875690717683, -11.40355824106234373, 43.00404056962644717 ) ) ;
#3737=CARTESIAN_POINT ( 'NONE',  ( -10.15407889436378852, -10.15407889436390576, 46.50000000000002132 ) ) ;
#3739=CARTESIAN_POINT ( 'NONE',  ( -4.623906867372410190, 13.21436662431711895, 48.42857142857143060 ) ) ;
#3741=CARTESIAN_POINT ( 'NONE',  ( 11.40355824106246985, -11.22385875690704538, 4.995959430373563492 ) ) ;
#3743=CARTESIAN_POINT ( 'NONE',  ( -1.837501619626328297, 16.30827793483733856, 36.64285714285714590 ) ) ;
#3750=CARTESIAN_POINT ( 'NONE',  ( 13.82664651025767100, -8.841785722321541030, 18.78975485534072121 ) ) ;
#3751=CARTESIAN_POINT ( 'NONE',  ( 1.837501619626330074, -16.30827793483733501, 45.64285714285716011 ) ) ;
#3754=CARTESIAN_POINT ( 'NONE',  ( 5.164528828830335705, -15.14410076328347543, 13.43261199819786711 ) ) ;
#3756=CARTESIAN_POINT ( 'NONE',  ( 10.15407889436379030, 10.15407889436390576, 31.50000000000001421 ) ) ;
#3757=CARTESIAN_POINT ( 'NONE',  ( -5.420364854931999155, -15.49051278174644253, 22.07142857142858006 ) ) ;
#3758=CARTESIAN_POINT ( 'NONE',  ( 5.420364854932001819, 15.49051278174644430, 49.07142857142859071 ) ) ;
#3762=CARTESIAN_POINT ( 'NONE',  ( -5.420364854931998266, -15.49051278174643898, 46.07142857142857650 ) ) ;
#3765=CARTESIAN_POINT ( 'NONE',  ( 11.31370849898482334, -11.31370849898469366, 9.000000000000001776 ) ) ;
#3766=CARTESIAN_POINT ( 'NONE',  ( 11.31370849898482334, -11.31370849898469366, 3.000000000000002665 ) ) ;
#3768=CARTESIAN_POINT ( 'NONE',  ( -12.15899005565164792, 7.639999817571650809, 23.78571428571429180 ) ) ;
#3770=CARTESIAN_POINT ( 'NONE',  ( -9.809645194534070356, 9.989344678689256796, 22.00404056962643651 ) ) ;
#3771=CARTESIAN_POINT ( 'NONE',  ( -9.989344678689363377, 9.809645194533960222, 43.99595943037355994 ) ) ;
#3775=CARTESIAN_POINT ( 'NONE',  ( 13.96533075980324234, -8.621071003556521006, 22.78167371608784464 ) ) ;
#3776=CARTESIAN_POINT ( 'NONE',  ( 16.30827793483735633, -1.837501619626142890, 2.357142857142856762 ) ) ;
#3778=CARTESIAN_POINT ( 'NONE',  ( 15.44746603149413922, 5.543385399275817527, 27.92453085894499054 ) ) ;
#3782=CARTESIAN_POINT ( 'NONE',  ( -14.25515036105622890, 1.737328882695209575, 27.36118342676929416 ) ) ;
#3786=CARTESIAN_POINT ( 'NONE',  ( -14.28433602490915000, 1.478298951650542481, 7.353102287516419366 ) ) ;
#3790=CARTESIAN_POINT ( 'NONE',  ( 13.25633410266679313, -4.503970704919842305, 16.56738800180213289 ) ) ;
#3794=CARTESIAN_POINT ( 'NONE',  ( 9.899494936611718643, -9.899494936611608509, 39.00000000000000000 ) ) ;
#3795=CARTESIAN_POINT ( 'NONE',  ( 12.15899005565164792, -7.639999817571655250, 44.78571428571428470 ) ) ;
#3797=CARTESIAN_POINT ( 'NONE',  ( -15.88516839912898071, -1.917699372586004980, 13.13881657323070584 ) ) ;
#3799=CARTESIAN_POINT ( 'NONE',  ( -1.837501619626328297, 16.30827793483733856, 24.64285714285714235 ) ) ;
#3806=CARTESIAN_POINT ( 'NONE',  ( -11.31370849898482156, 11.31370849898469544, 42.00000000000000000 ) ) ;
#3808=CARTESIAN_POINT ( 'NONE',  ( 15.06016580658428694, -5.404401153735007846, 18.57546914105500235 ) ) ;
#3811=CARTESIAN_POINT ( 'NONE',  ( -15.89939535829186923, -1.791431617653016062, 23.14285714285714590 ) ) ;
#3816=CARTESIAN_POINT ( 'NONE',  ( 1.837501619626329630, -16.30827793483733501, 45.64285714285715301 ) ) ;
#3821=CARTESIAN_POINT ( 'NONE',  ( -5.420364854931999155, -15.49051278174644253, 4.071428571428569398 ) ) ;
#3822=CARTESIAN_POINT ( 'NONE',  ( -8.731428362939189114, 13.89598863503036341, 6.214285714285717965 ) ) ;
#3823=CARTESIAN_POINT ( 'NONE',  ( -4.742819248065500481, -13.55419868402813499, 28.07142857142857295 ) ) ;
#3825=CARTESIAN_POINT ( 'NONE',  ( 13.25633410266679313, -4.503970704919842305, 46.56738800180214355 ) ) ;
#3828=CARTESIAN_POINT ( 'NONE',  ( -13.47998361472151174, -8.620103694222146729, 24.71024514465928235 ) ) ;
#3829=CARTESIAN_POINT ( 'NONE',  ( 1.791431617652837316, 15.89939535829188877, 6.857142857142860315 ) ) ;
#3831=CARTESIAN_POINT ( 'NONE',  ( 1.665163862719847732, 15.91362231745477374, 20.85310228751641759 ) ) ;
#3835=CARTESIAN_POINT ( 'NONE',  ( -1.693770420379220099, -13.89774397934251837, 37.86118342676929416 ) ) ;
#3838=CARTESIAN_POINT ( 'NONE',  ( -12.22833218042443271, 7.529642458189139909, 7.781673716087849968 ) ) ;
#3841=CARTESIAN_POINT ( 'NONE',  ( -5.284464991282755264, 15.10213328493384743, 30.42857142857143060 ) ) ;
#3843=CARTESIAN_POINT ( 'NONE',  ( -14.28433602490915000, 1.478298951650542481, 31.35310228751642470 ) ) ;
#3847=CARTESIAN_POINT ( 'NONE',  ( -9.809645194534070356, 9.989344678689256796, 10.00404056962643651 ) ) ;
#3848=CARTESIAN_POINT ( 'NONE',  ( -7.639999817571787588, 12.15899005565156266, 48.21428571428570820 ) ) ;
#3850=CARTESIAN_POINT ( 'NONE',  ( -8.841785722321695573, 13.82664651025757152, 14.21024514465927702 ) ) ;
#3852=CARTESIAN_POINT ( 'NONE',  ( 13.89598863503046111, -8.731428362939032795, 38.78571428571429180 ) ) ;
#3858=CARTESIAN_POINT ( 'NONE',  ( -11.60466159355861926, -11.60466159355875249, 40.50000000000000711 ) ) ;
#3861=CARTESIAN_POINT ( 'NONE',  ( 5.543385399275644332, 15.44746603149420494, 17.07546914105500591 ) ) ;
#3862=CARTESIAN_POINT ( 'NONE',  ( -13.89598863503046111, 8.731428362939027465, 23.78571428571429536 ) ) ;
#3863=CARTESIAN_POINT ( 'NONE',  ( 1.805317605496833622, 15.89926306122265309, 48.73000000000001108 ) ) ;
#3865=CARTESIAN_POINT ( 'NONE',  ( -11.31370849898482156, 11.31370849898469544, 48.00000000000000000 ) ) ;
#3867=CARTESIAN_POINT ( 'NONE',  ( 13.89598863503046111, -8.731428362939032795, 2.785714285714284255 ) ) ;
#3868=CARTESIAN_POINT ( 'NONE',  ( 1.791431617652837316, 15.89939535829188877, 0.8571428571428549859 ) ) ;
#3870=CARTESIAN_POINT ( 'NONE',  ( -10.15407889436378852, -10.15407889436390398, 22.50000000000000355 ) ) ;
#3872=CARTESIAN_POINT ( 'NONE',  ( 1.693770420379222319, 13.89774397934251837, 34.86118342676929416 ) ) ;
#3875=CARTESIAN_POINT ( 'NONE',  ( 7.750357176954296712, -12.08964793087877787, 35.21024514465927524 ) ) ;
#3878=CARTESIAN_POINT ( 'NONE',  ( -16.32287076676382398, 1.707986654103809343, 25.35310228751642470 ) ) ;
#3879=CARTESIAN_POINT ( 'NONE',  ( 8.512513224245308763, 13.54758718765259040, 7.285714285714284699 ) ) ;
#3881=CARTESIAN_POINT ( 'NONE',  ( -15.88516839912898071, -1.917699372586004980, 25.13881657323070939 ) ) ;
#3887=CARTESIAN_POINT ( 'NONE',  ( -1.737328882695368115, 14.25515036105620581, 2.638816573230710727 ) ) ;
#3890=CARTESIAN_POINT ( 'NONE',  ( -1.441234910513241818, -13.92619789766829008, 29.85310228751642470 ) ) ;
#3894=CARTESIAN_POINT ( 'NONE',  ( 14.25515036105622535, -1.737328882695210241, 0.3611834267692887734 ) ) ;
#3896=CARTESIAN_POINT ( 'NONE',  ( 4.623906867372411078, -13.21436662431711717, 45.42857142857143060 ) ) ;
#3898=CARTESIAN_POINT ( 'NONE',  ( 8.404922754268618235, 13.61519076058357491, 9.281673716087846415 ) ) ;
#3900=CARTESIAN_POINT ( 'NONE',  ( 8.731428362939190890, -13.89598863503036164, 39.21428571428571530 ) ) ;
#3907=CARTESIAN_POINT ( 'NONE',  ( 13.82664651025767100, -8.841785722321541030, 30.78975485534071765 ) ) ;
#3908=CARTESIAN_POINT ( 'NONE',  ( 13.89598863503046111, -8.731428362939032795, 20.78571428571429180 ) ) ;
#3910=CARTESIAN_POINT ( 'NONE',  ( 13.89598863503046111, -8.731428362939032795, 8.785714285714293581 ) ) ;
#3913=CARTESIAN_POINT ( 'NONE',  ( -11.60466159355861926, -11.60466159355875249, 4.500000000000005329 ) ) ;
#3914=CARTESIAN_POINT ( 'NONE',  ( -15.49051278174638036, -5.420364854932175902, 10.92857142857142883 ) ) ;
#3916=CARTESIAN_POINT ( 'NONE',  ( 4.623906867372411078, -13.21436662431711717, 45.42857142857143060 ) ) ;
#3917=CARTESIAN_POINT ( 'NONE',  ( 11.92174236212692229, 7.340858601238088532, 29.71832628391214826 ) ) ;
#3922=CARTESIAN_POINT ( 'NONE',  ( 13.21436662431716869, -4.623906867372263640, 8.571428571428569398 ) ) ;
#3925=CARTESIAN_POINT ( 'NONE',  ( 13.47998361472151529, 8.620103694222146729, 21.71024514465928235 ) ) ;
#3926=COLOUR_RGB ( '', 0.40784314, 0.44705882, 0.49803922) ;
#3927=CARTESIAN_POINT ( 'NONE',  ( 15.49051278174637858, 5.420364854932174126, 1.928571428571430380 ) ) ;
#3928=CARTESIAN_POINT ( 'NONE',  ( 8.841785722321695573, -13.82664651025757152, 17.21024514465927879 ) ) ;
#3934=CARTESIAN_POINT ( 'NONE',  ( -5.420364854931999155, -15.49051278174644253, 34.07142857142859071 ) ) ;
#3935=ORIENTED_EDGE ( 'NONE', *, *, #10187, .F. ) ;
#3936=CARTESIAN_POINT ( 'NONE',  ( 16.32287076676382043, -1.707986654103810897, 46.35310228751641404 ) ) ;
#3939=CARTESIAN_POINT ( 'NONE',  ( -7.340858601237953529, -11.92174236212700222, 24.28167371608785530 ) ) ;
#3943=CARTESIAN_POINT ( 'NONE',  ( 1.478298951650704351, -14.28433602490913579, 1.646897712483578857 ) ) ;
#3944=CARTESIAN_POINT ( 'NONE',  ( 13.92619789766827587, 1.441234910513398582, 18.14689771248357530 ) ) ;
#3946=CARTESIAN_POINT ( 'NONE',  ( -8.404922754268618235, -13.61519076058357491, 12.28167371608784997 ) ) ;
#3948=CARTESIAN_POINT ( 'NONE',  ( -15.89939535829186923, -1.791431617653016062, 47.14285714285714590 ) ) ;
#3952=ADVANCED_FACE ( 'NONE', ( #4653 ), #6965, .T. ) ;
#3954=CARTESIAN_POINT ( 'NONE',  ( -1.707986654103994528, 16.32287076676380266, 28.64689771248357886 ) ) ;
#3956=SHAPE_REPRESENTATION ( 'main spring', ( #3995 ), #5075 ) ;
#3957=CARTESIAN_POINT ( 'NONE',  ( 15.06016580658428694, -5.404401153735007846, 30.57546914105500946 ) ) ;
#3961=CARTESIAN_POINT ( 'NONE',  ( 13.54758718765249803, 8.512513224245457977, 13.71428571428571352 ) ) ;
#3964=FACE_OUTER_BOUND ( 'NONE', #6307, .T. ) ;
#3968=CARTESIAN_POINT ( 'NONE',  ( 13.92619789766827587, 1.441234910513398582, 42.14689771248358596 ) ) ;
#3970=CARTESIAN_POINT ( 'NONE',  ( -13.54758718765249625, -8.512513224245459753, 16.71428571428571530 ) ) ;
#3972=CARTESIAN_POINT ( 'NONE',  ( 11.85413878919593422, 7.448449071214774619, 37.71428571428571530 ) ) ;
#3975=ORIENTED_EDGE ( 'NONE', *, *, #2410, .T. ) ;
#3976=CARTESIAN_POINT ( 'NONE',  ( 9.809645194533960222, 9.989344678689363377, 51.49595943037355994 ) ) ;
#3980=CARTESIAN_POINT ( 'NONE',  ( -15.14410076328353227, 5.164528828830164287, 31.56738800180213644 ) ) ;
#3982=CARTESIAN_POINT ( 'NONE',  ( -15.49051278174637858, -5.420364854932175014, 22.92857142857143060 ) ) ;
#3983=CARTESIAN_POINT ( 'NONE',  ( -1.967016585148659846, 16.29368510291087091, 20.63881657323070939 ) ) ;
#3990=CARTESIAN_POINT ( 'NONE',  ( 9.989344678689365153, -9.809645194533958446, 10.99595943037356882 ) ) ;
#3995=AXIS2_PLACEMENT_3D ( 'NONE', #245, #8930, #7419 ) ;
#3996=CARTESIAN_POINT ( 'NONE',  ( -12.22833218042443271, 7.529642458189139909, 25.78167371608785530 ) ) ;
#4000=CARTESIAN_POINT ( 'NONE',  ( 13.92619789766827587, 1.441234910513398582, 12.14689771248358063 ) ) ;
#4001=CARTESIAN_POINT ( 'NONE',  ( -12.08964793087886314, 7.750357176954159932, 9.789754855340722983 ) ) ;
#4005=CARTESIAN_POINT ( 'NONE',  ( -5.404401153735176599, 15.06016580658422477, 2.424530858944988321 ) ) ;
#4010=CARTESIAN_POINT ( 'NONE',  ( -5.164528828830334817, 15.14410076328347543, 28.43261199819786356 ) ) ;
#4012=CARTESIAN_POINT ( 'NONE',  ( 8.621071003556677326, -13.96533075980314287, 37.21832628391215536 ) ) ;
#4014=CARTESIAN_POINT ( 'NONE',  ( -5.420364854931999155, -15.49051278174644253, 34.07142857142859071 ) ) ;
#4023=CARTESIAN_POINT ( 'NONE',  ( 1.917699372585825790, 15.88516839912900203, -1.138816573230706286 ) ) ;
#4024=CARTESIAN_POINT ( 'NONE',  ( -15.49051278174638036, -5.420364854932175902, 16.92857142857143771 ) ) ;
#4026=CARTESIAN_POINT ( 'NONE',  ( -12.15899005565164792, 7.639999817571650809, 41.78571428571429180 ) ) ;
#4027=CARTESIAN_POINT ( 'NONE',  ( -12.08964793087886314, 7.750357176954159932, 45.78975485534073897 ) ) ;
#4028=CARTESIAN_POINT ( 'NONE',  ( -13.21436662431716869, 4.623906867372262752, 5.571428571428574728 ) ) ;
#4032=CARTESIAN_POINT ( 'NONE',  ( -10.15407889436378852, -10.15407889436390576, 4.500000000000005329 ) ) ;
#4035=CARTESIAN_POINT ( 'NONE',  ( -1.791431617652833763, -15.89939535829188877, 21.85714285714286120 ) ) ;
#4036=CARTESIAN_POINT ( 'NONE',  ( -15.44746603149413922, -5.543385399275820191, 42.92453085894499054 ) ) ;
#4041=CARTESIAN_POINT ( 'NONE',  ( -12.22833218042443271, 7.529642458189139909, 13.78167371608785174 ) ) ;
#4043=CARTESIAN_POINT ( 'NONE',  ( 1.837501619626330074, -16.30827793483733501, 15.64285714285714235 ) ) ;
#4048=CARTESIAN_POINT ( 'NONE',  ( -13.17239914596754424, 4.743843029824683200, 3.575469141055005462 ) ) ;
#4049=CARTESIAN_POINT ( 'NONE',  ( -10.24623928997352351, -10.06191849875416899, 14.50404056962643651 ) ) ;
#4052=CARTESIAN_POINT ( 'NONE',  ( 15.10213328493390783, -5.284464991282587398, 44.57142857142857650 ) ) ;
#4059=CARTESIAN_POINT ( 'NONE',  ( 15.91362231745475597, 1.665163862720026255, 30.14689771248358241 ) ) ;
#4061=CARTESIAN_POINT ( 'NONE',  ( -8.621071003556675549, 13.96533075980314642, 34.21832628391215536 ) ) ;
#4063=CARTESIAN_POINT ( 'NONE',  ( 15.89939535829187278, 1.791431617653015174, 32.14285714285714590 ) ) ;
#4064=CARTESIAN_POINT ( 'NONE',  ( 3.896594582693065245, 14.56547797550490309, 3.589645083274735104E-17 ) ) ;
#4069=CARTESIAN_POINT ( 'NONE',  ( -15.91362231745475597, -1.665163862720028254, 3.146897712483577969 ) ) ;
#4070=CARTESIAN_POINT ( 'NONE',  ( 1.837501619626330074, -16.30827793483733501, 21.64285714285714590 ) ) ;
#4071=CARTESIAN_POINT ( 'NONE',  ( 13.55419868402807992, 4.742819248065649695, 37.92857142857143060 ) ) ;
#4072=CARTESIAN_POINT ( 'NONE',  ( 1.693770420379222319, 13.89774397934251837, 40.86118342676929416 ) ) ;
#4073=CARTESIAN_POINT ( 'NONE',  ( 7.448449071214646722, 11.85413878919601594, 7.285714285714284699 ) ) ;
#4076=CARTESIAN_POINT ( 'NONE',  ( 10.15407889436379030, 10.15407889436390576, 7.500000000000005329 ) ) ;
#4078=CARTESIAN_POINT ( 'NONE',  ( -5.420364854931998266, -15.49051278174643898, 16.07142857142857650 ) ) ;
#4079=CARTESIAN_POINT ( 'NONE',  ( 13.47998361472151529, 8.620103694222146729, 39.71024514465927524 ) ) ;
#4086=CARTESIAN_POINT ( 'NONE',  ( -9.989344678689363377, 9.809645194533960222, 13.99595943037356527 ) ) ;
#4088=CARTESIAN_POINT ( 'NONE',  ( -11.31370849898482156, 11.31370849898469544, 11.99999999999999645 ) ) ;
#4090=CARTESIAN_POINT ( 'NONE',  ( 13.54758718765249803, 8.512513224245457977, 37.71428571428571530 ) ) ;
#4091=CARTESIAN_POINT ( 'NONE',  ( -11.78653521626494793, -7.556039541191465148, 36.71024514465928235 ) ) ;
#4097=CARTESIAN_POINT ( 'NONE',  ( -13.59724543428031573, -4.619798703722008959, 14.93261199819787066 ) ) ;
#4099=CARTESIAN_POINT ( 'NONE',  ( 1.478298951650704351, -14.28433602490913579, 7.646897712483577969 ) ) ;
#4102=CARTESIAN_POINT ( 'NONE',  ( -13.47998361472151174, -8.620103694222146729, 12.71024514465927879 ) ) ;
#4109=CARTESIAN_POINT ( 'NONE',  ( 1.917699372585825790, 15.88516839912900203, 22.86118342676929061 ) ) ;
#4111=CARTESIAN_POINT ( 'NONE',  ( 5.164528828830335705, -15.14410076328347543, 31.43261199819787421 ) ) ;
#4113=CARTESIAN_POINT ( 'NONE',  ( 13.54758718765249803, 8.512513224245457977, 37.71428571428571530 ) ) ;
#4115=CARTESIAN_POINT ( 'NONE',  ( 16.30827793483735633, -1.837501619626142890, 8.357142857142855874 ) ) ;
#4120=CARTESIAN_POINT ( 'NONE',  ( 13.59724543428031573, 4.619798703722006294, 41.93261199819787066 ) ) ;
#4121=CARTESIAN_POINT ( 'NONE',  ( -5.420364854931999155, -15.49051278174644253, 10.07142857142856940 ) ) ;
#4122=CARTESIAN_POINT ( 'NONE',  ( 4.865839792409144771, 13.51115193377589740, 41.07546914105501656 ) ) ;
#4123=CARTESIAN_POINT ( 'NONE',  ( 13.55419868402807992, 4.742819248065648807, 7.928571428571430602 ) ) ;
#4127=CARTESIAN_POINT ( 'NONE',  ( -4.623906867372410190, 13.21436662431711895, 0.4285714285714309346 ) ) ;
#4130=CARTESIAN_POINT ( 'NONE',  ( 5.284464991282756152, -15.10213328493384743, 21.42857142857142705 ) ) ;
#4132=CARTESIAN_POINT ( 'NONE',  ( 13.47998361472151529, 8.620103694222146729, 33.71024514465927524 ) ) ;
#4147=CARTESIAN_POINT ( 'NONE',  ( -1.478298951650703019, 14.28433602490913579, 16.64689771248358596 ) ) ;
#4149=CARTESIAN_POINT ( 'NONE',  ( 9.809645194534072132, -9.989344678689256796, 7.004040569626434731 ) ) ;
#4152=CARTESIAN_POINT ( 'NONE',  ( 11.51250119794888249, 11.69682198916847682, 15.49595943037356882 ) ) ;
#4158=CARTESIAN_POINT ( 'NONE',  ( -5.164528828830334817, 15.14410076328347543, 34.43261199819786356 ) ) ;
#4160=CARTESIAN_POINT ( 'NONE',  ( 10.15407889436379030, 10.15407889436390576, 25.50000000000000711 ) ) ;
#4162=CARTESIAN_POINT ( 'NONE',  ( 15.53355953199861794, 5.297344310588528060, 41.93261199819787066 ) ) ;
#4165=CARTESIAN_POINT ( 'NONE',  ( 11.60466159355862104, 11.60466159355875071, 37.50000000000002842 ) ) ;
#4167=CARTESIAN_POINT ( 'NONE',  ( -5.284464991282755264, 15.10213328493384743, 12.42857142857142705 ) ) ;
#4171=CARTESIAN_POINT ( 'NONE',  ( -4.503970704919988854, 13.25633410266674517, 40.43261199819787066 ) ) ;
#4172=CARTESIAN_POINT ( 'NONE',  ( 8.731428362939190890, -13.89598863503036164, 33.21428571428571530 ) ) ;
#4173=CARTESIAN_POINT ( 'NONE',  ( 13.92619789766827587, 1.441234910513398582, 42.14689771248358596 ) ) ;
#4175=CARTESIAN_POINT ( 'NONE',  ( -1.567502665446231180, -13.91197093850540334, 15.85714285714286120 ) ) ;
#4179=CARTESIAN_POINT ( 'NONE',  ( 1.607813917173038121, -14.26974319298267346, 21.64285714285714590 ) ) ;
#4182=CARTESIAN_POINT ( 'NONE',  ( -13.89598863503045933, 8.731428362939027465, 11.78571428571428292 ) ) ;
#4183=CARTESIAN_POINT ( 'NONE',  ( -8.841785722321695573, 13.82664651025757152, 38.21024514465928235 ) ) ;
#4187=CARTESIAN_POINT ( 'NONE',  ( -13.21436662431716869, 4.623906867372262752, 11.57142857142857295 ) ) ;
#4188=CARTESIAN_POINT ( 'NONE',  ( -13.51115193377584589, -4.865839792409295761, 24.92453085894499765 ) ) ;
#4191=CARTESIAN_POINT ( 'NONE',  ( -15.89939535829186923, -1.791431617653016062, 17.14285714285713880 ) ) ;
#4193=CARTESIAN_POINT ( 'NONE',  ( -11.78653521626494793, -7.556039541191465148, 42.71024514465928235 ) ) ;
#4197=CARTESIAN_POINT ( 'NONE',  ( 14.25515036105622535, -1.737328882695210241, 18.36118342676929771 ) ) ;
#4198=CARTESIAN_POINT ( 'NONE',  ( 7.556039541191335474, 11.78653521626503320, 23.28975485534072121 ) ) ;
#4200=CARTESIAN_POINT ( 'NONE',  ( 5.297344310588354865, 15.53355953199867301, 9.067388001802141773 ) ) ;
#4206=CARTESIAN_POINT ( 'NONE',  ( -13.91197093850538380, -1.567502665446387278, 35.14285714285713880 ) ) ;
#4208=CARTESIAN_POINT ( 'NONE',  ( -9.899494936611716867, 9.899494936611610285, 36.00000000000000711 ) ) ;
#4210=CARTESIAN_POINT ( 'NONE',  ( 13.54758718765249803, 8.512513224245457977, 25.71428571428571885 ) ) ;
#4212=CARTESIAN_POINT ( 'NONE',  ( -15.10213328493390961, 5.284464991282586510, 11.57142857142857295 ) ) ;
#4217=CARTESIAN_POINT ( 'NONE',  ( -13.82664651025767100, 8.841785722321537477, 15.78975485534072121 ) ) ;
#4218=CARTESIAN_POINT ( 'NONE',  ( 16.30827793483735633, -1.837501619626142890, 26.35714285714285765 ) ) ;
#4221=CARTESIAN_POINT ( 'NONE',  ( -5.164528828830334817, 15.14410076328347543, 4.432611998197859116 ) ) ;
#4223=CARTESIAN_POINT ( 'NONE',  ( 14.26974319298268767, -1.607813917172876916, 8.357142857142855874 ) ) ;
#4227=CARTESIAN_POINT ( 'NONE',  ( 13.91197093850538380, 1.567502665446386390, 14.14285714285714413 ) ) ;
#4228=CARTESIAN_POINT ( 'NONE',  ( 13.54758718765249803, 8.512513224245457977, 31.71428571428571530 ) ) ;
#4229=CARTESIAN_POINT ( 'NONE',  ( 8.404922754268618235, 13.61519076058357491, 33.28167371608784464 ) ) ;
#4231=CARTESIAN_POINT ( 'NONE',  ( 13.21436662431716869, -4.623906867372263640, 14.57142857142856940 ) ) ;
#4232=CARTESIAN_POINT ( 'NONE',  ( -11.78653521626494793, -7.556039541191465148, 24.71024514465928235 ) ) ;
#4234=B_SPLINE_CURVE_WITH_KNOTS ( 'NONE', 3,
 ( #4938, #4262, #1016, #6372, #2607, #7312, #8037, #2560, #288, #185, #236, #9550, #2509, #5751, #4991, #6520, #1069, #1739, #5803, #8980, #5658, #6424, #2457, #5603, #9699, #1694, #8768, #4835, #4064, #8919, #7211, #9605, #8826, #4889, #964, #9849, #6618, #6050, #4362, #9180, #4465, #8389, #2707, #9074, #3633, #2907, #8339, #3582, #1257, #338, #4522, #9225, #7621, #7515, #4416, #1312, #2141, #542 ),
 .UNSPECIFIED., .F., .F.,
 ( 4, 2, 2, 2, 2, 2, 2, 2, 2, 2, 2, 2, 2, 2, 2, 2, 2, 2, 2, 2, 2, 2, 2, 2, 2, 2, 2, 2, 4 ),
 ( 0.000000000000000000, 0.002013233252797604154, 0.004026466505595208308, 0.006039699758392812895, 0.008052933011190416615, 0.01207939951678562579, 0.01308601614318442678, 0.01409263276958323124, 0.01459594108278263087, 0.01484759523938233156, 0.01497342231768217929, 0.01503633585683210490, 0.01509924939598203050, 0.01516216293513195611, 0.01522507647428187998, 0.01535090355258173465, 0.01560255770918144401, 0.01610586602238086099, 0.01711248264877969841, 0.01811909927517853583, 0.02013233252797621067, 0.02113894915437504810, 0.02214556578077388899, 0.02415879903357156383, 0.02516541565997040125, 0.02617203228636923867, 0.02818526553916691699, 0.03019849879196460224, 0.03221173204476228402 ),
 .UNSPECIFIED. ) ;
#4236=EDGE_CURVE ( 'NONE', #6181, #6566, #7850, .T. ) ;
#4237=CARTESIAN_POINT ( 'NONE',  ( -1.737328882695368115, 14.25515036105620581, 32.63881657323070584 ) ) ;
#4241=EDGE_CURVE ( 'NONE', #6181, #6566, #9457, .T. ) ;
#4243=CARTESIAN_POINT ( 'NONE',  ( -7.529642458189277576, 12.22833218042435455, 22.21832628391215181 ) ) ;
#4244=CARTESIAN_POINT ( 'NONE',  ( -12.08964793087886314, 7.750357176954159932, 27.78975485534072121 ) ) ;
#4246=CARTESIAN_POINT ( 'NONE',  ( 8.841785722321695573, -13.82664651025757152, 35.21024514465927524 ) ) ;
#4248=CARTESIAN_POINT ( 'NONE',  ( -11.67616201620524130, 10.40597831933767736, 48.73000000000001108 ) ) ;
#4249=CARTESIAN_POINT ( 'NONE',  ( 15.49051278174638036, 5.420364854932175014, 19.92857142857143771 ) ) ;
#4250=CARTESIAN_POINT ( 'NONE',  ( -15.14410076328353227, 5.164528828830164287, 13.56738800180213822 ) ) ;
#4253=STYLED_ITEM ( 'NONE', ( #7960 ), #939 ) ;
#4257=CARTESIAN_POINT ( 'NONE',  ( 1.567502665446232957, 13.91197093850540156, 36.85714285714286120 ) ) ;
#4258=CARTESIAN_POINT ( 'NONE',  ( -1.567502665446231180, -13.91197093850540334, 33.85714285714285410 ) ) ;
#4261=CARTESIAN_POINT ( 'NONE',  ( -5.404401153735176599, 15.06016580658422477, 2.424530858944988321 ) ) ;
#4262=CARTESIAN_POINT ( 'NONE',  ( -9.423904007443638875, 10.37508586577969183, -0.000000000000000000 ) ) ;
#4263=CARTESIAN_POINT ( 'NONE',  ( -13.54758718765249625, -8.512513224245459753, 22.71428571428571530 ) ) ;
#4268=CARTESIAN_POINT ( 'NONE',  ( -11.22385875690717327, 11.40355824106234550, 4.004040569626432067 ) ) ;
#4269=CARTESIAN_POINT ( 'NONE',  ( -1.837501619626328297, 16.30827793483733856, 30.64285714285715301 ) ) ;
#4271=CARTESIAN_POINT ( 'NONE',  ( -5.164528828830334817, 15.14410076328347543, 10.43261199819786356 ) ) ;
#4272=CARTESIAN_POINT ( 'NONE',  ( -12.15899005565164792, 7.639999817571651697, 29.78571428571428825 ) ) ;
#4273=CARTESIAN_POINT ( 'NONE',  ( -5.420364854931999155, -15.49051278174644253, 4.071428571428569398 ) ) ;
#4276=CARTESIAN_POINT ( 'NONE',  ( -13.21436662431716869, 4.623906867372262752, 23.57142857142857650 ) ) ;
#4278=CARTESIAN_POINT ( 'NONE',  ( 16.30827793483735633, -1.837501619626142890, 32.35714285714286120 ) ) ;
#4279=CARTESIAN_POINT ( 'NONE',  ( -1.737328882695368115, 14.25515036105620581, 2.638816573230710727 ) ) ;
#4281=CARTESIAN_POINT ( 'NONE',  ( 14.26974319298268767, -1.607813917172876472, 8.357142857142855874 ) ) ;
#4283=CARTESIAN_POINT ( 'NONE',  ( -13.51115193377584589, -4.865839792409295761, 30.92453085894499765 ) ) ;
#4286=CARTESIAN_POINT ( 'NONE',  ( 4.398722002148208077, 13.35545020628939739, 48.73000000000001819 ) ) ;
#4291=CARTESIAN_POINT ( 'NONE',  ( -10.24623928997352351, -10.06191849875416899, 20.50404056962644006 ) ) ;
#4294=CARTESIAN_POINT ( 'NONE',  ( 1.693770420379222319, 13.89774397934251837, 22.86118342676929061 ) ) ;
#4296=CARTESIAN_POINT ( 'NONE',  ( -15.88516839912898071, -1.917699372586004980, 43.13881657323070584 ) ) ;
#4297=CARTESIAN_POINT ( 'NONE',  ( -12.16676467619702606, 8.075659364407771434, 48.73000000000002530 ) ) ;
#4298=CARTESIAN_POINT ( 'NONE',  ( -5.420364854931999155, -15.49051278174644253, 22.07142857142858006 ) ) ;
#4299=CARTESIAN_POINT ( 'NONE',  ( 1.665163862719847732, 15.91362231745477374, 2.853102287516426916 ) ) ;
#4307=CARTESIAN_POINT ( 'NONE',  ( 13.91197093850538380, 1.567502665446386390, 26.14285714285714590 ) ) ;
#4311=CARTESIAN_POINT ( 'NONE',  ( 7.448449071214646722, 11.85413878919601594, 43.28571428571429180 ) ) ;
#4313=CARTESIAN_POINT ( 'NONE',  ( 1.791431617652837316, 15.89939535829188877, 42.85714285714285410 ) ) ;
#4315=CARTESIAN_POINT ( 'NONE',  ( -8.731428362939189114, 13.89598863503036341, 12.21428571428571885 ) ) ;
#4321=CARTESIAN_POINT ( 'NONE',  ( -5.543385399275643444, -15.44746603149420494, 14.07546914105500768 ) ) ;
#4322=CARTESIAN_POINT ( 'NONE',  ( -13.54758718765249625, -8.512513224245459753, 22.71428571428571530 ) ) ;
#4323=CARTESIAN_POINT ( 'NONE',  ( -11.22385875690717327, 11.40355824106234550, 10.00404056962643651 ) ) ;
#4324=CARTESIAN_POINT ( 'NONE',  ( -9.899494936611716867, 9.899494936611610285, 30.00000000000000355 ) ) ;
#4325=CARTESIAN_POINT ( 'NONE',  ( -13.89598863503046111, 8.731428362939027465, 11.78571428571428115 ) ) ;
#4328=CARTESIAN_POINT ( 'NONE',  ( 1.567502665446232957, 13.91197093850540156, 18.85714285714285765 ) ) ;
#4330=CARTESIAN_POINT ( 'NONE',  ( -1.837501619626327853, 16.30827793483733856, 36.64285714285714590 ) ) ;
#4331=CARTESIAN_POINT ( 'NONE',  ( 13.51115193377584589, 4.865839792409294873, 3.924530858944990541 ) ) ;
#4334=CARTESIAN_POINT ( 'NONE',  ( 1.567502665446232957, 13.91197093850540156, 6.857142857142860315 ) ) ;
#4335=CARTESIAN_POINT ( 'NONE',  ( 14.28433602490915000, -1.478298951650544479, 28.35310228751642825 ) ) ;
#4340=CARTESIAN_POINT ( 'NONE',  ( 12.15899005565164792, -7.639999817571655250, 2.785714285714284255 ) ) ;
#4344=CARTESIAN_POINT ( 'NONE',  ( 13.17239914596754424, -4.743843029824685864, 30.57546914105500946 ) ) ;
#4345=CARTESIAN_POINT ( 'NONE',  ( -11.92174236212692051, -7.340858601238089420, 20.71832628391214826 ) ) ;
#4348=CARTESIAN_POINT ( 'NONE',  ( -8.841785722321695573, 13.82664651025757152, 38.21024514465928235 ) ) ;
#4349=CARTESIAN_POINT ( 'NONE',  ( -10.03741027250566020, 10.21278494640099588, 48.73000000000001819 ) ) ;
#4350=CARTESIAN_POINT ( 'NONE',  ( -1.837501619626328297, 16.30827793483733856, 24.64285714285714235 ) ) ;
#4353=CARTESIAN_POINT ( 'NONE',  ( -13.51115193377584589, -4.865839792409295761, 12.92453085894499587 ) ) ;
#4357=CARTESIAN_POINT ( 'NONE',  ( 8.620103694221997515, 13.47998361472160767, 35.28975485534072476 ) ) ;
#4358=CARTESIAN_POINT ( 'NONE',  ( 1.567502665446232957, 13.91197093850540156, 30.85714285714286120 ) ) ;
#4359=CARTESIAN_POINT ( 'NONE',  ( -1.567502665446231180, -13.91197093850540334, 39.85714285714286120 ) ) ;
#4361=CARTESIAN_POINT ( 'NONE',  ( -13.54758718765249625, -8.512513224245459753, 46.71428571428571530 ) ) ;
#4362=CARTESIAN_POINT ( 'NONE',  ( 1.550455870813287396, 15.46333760686143144, 9.306676823330681010E-17 ) ) ;
#4363=CARTESIAN_POINT ( 'NONE',  ( -16.30827793483735988, 1.837501619626141780, 35.35714285714285410 ) ) ;
#4372=CARTESIAN_POINT ( 'NONE',  ( 15.06016580658428694, -5.404401153735007846, 6.575469141055007682 ) ) ;
#4373=CARTESIAN_POINT ( 'NONE',  ( 15.89939535829187278, 1.791431617653015174, 26.14285714285714590 ) ) ;
#4375=CARTESIAN_POINT ( 'NONE',  ( 13.82664651025767100, -8.841785722321541030, 12.78975485534072121 ) ) ;
#4376=CARTESIAN_POINT ( 'NONE',  ( -4.623906867372410190, 13.21436662431711895, 18.42857142857143415 ) ) ;
#4377=CARTESIAN_POINT ( 'NONE',  ( -8.731428362939189114, 13.89598863503036341, 6.214285714285717965 ) ) ;
#4378=CARTESIAN_POINT ( 'NONE',  ( -16.30827793483735988, 1.837501619626141780, 41.35714285714286120 ) ) ;
#4380=CARTESIAN_POINT ( 'NONE',  ( -4.623906867372410190, 13.21436662431711895, 12.42857142857142705 ) ) ;
#4382=CARTESIAN_POINT ( 'NONE',  ( -16.30827793483735988, 1.837501619626141558, 35.35714285714286120 ) ) ;
#4383=CARTESIAN_POINT ( 'NONE',  ( 4.743843029824831525, -13.17239914596749095, 5.424530858944991429 ) ) ;
#4386=CARTESIAN_POINT ( 'NONE',  ( -14.26974319298268767, 1.607813917172874696, 5.357142857142856762 ) ) ;
#4388=CARTESIAN_POINT ( 'NONE',  ( -13.25633410266679313, 4.503970704919840529, 25.56738800180213644 ) ) ;
#4394=CARTESIAN_POINT ( 'NONE',  ( 1.737328882695370558, -14.25515036105620581, 47.63881657323071295 ) ) ;
#4398=CARTESIAN_POINT ( 'NONE',  ( 13.92619789766827587, 1.441234910513398582, 30.14689771248358241 ) ) ;
#4401=CARTESIAN_POINT ( 'NONE',  ( -5.404401153735176599, 15.06016580658422477, 38.42453085894499054 ) ) ;
#4402=CARTESIAN_POINT ( 'NONE',  ( -8.450287677708004708, 11.41786575994333042, 48.73000000000001819 ) ) ;
#4403=CARTESIAN_POINT ( 'NONE',  ( 11.60466159355862104, 11.60466159355875071, 19.50000000000000355 ) ) ;
#4406=CARTESIAN_POINT ( 'NONE',  ( -10.06191849875405531, -10.24623928997363542, 18.49595943037356705 ) ) ;
#4411=CARTESIAN_POINT ( 'NONE',  ( -7.529642458189277576, 12.22833218042435455, -1.781673716087850634 ) ) ;
#4413=CARTESIAN_POINT ( 'NONE',  ( -13.91197093850538380, -1.567502665446387278, 35.14285714285713880 ) ) ;
#4415=CARTESIAN_POINT ( 'NONE',  ( -11.40355824106246807, 11.22385875690704715, 1.995959430373561272 ) ) ;
#4416=CARTESIAN_POINT ( 'NONE',  ( -9.315939868251517098, 13.01050362062812660, 4.615094676506724096E-15 ) ) ;
#4417=CARTESIAN_POINT ( 'NONE',  ( 5.420364854932001819, 15.49051278174644430, 31.07142857142857295 ) ) ;
#4425=CARTESIAN_POINT ( 'NONE',  ( 1.707986654103998303, -16.32287076676380266, 13.64689771248357708 ) ) ;
#4426=CARTESIAN_POINT ( 'NONE',  ( -8.512513224245306986, -13.54758718765259218, 40.28571428571428470 ) ) ;
#4428=CARTESIAN_POINT ( 'NONE',  ( 1.707986654103998303, -16.32287076676380266, 1.646897712483578857 ) ) ;
#4429=CARTESIAN_POINT ( 'NONE',  ( -10.15407889436378852, -10.15407889436390576, 28.50000000000001066 ) ) ;
#4430=CARTESIAN_POINT ( 'NONE',  ( -5.284464991282755264, 15.10213328493384743, 6.428571428571429713 ) ) ;
#4431=CARTESIAN_POINT ( 'NONE',  ( 11.31370849898469899, 11.31370849898481978, 49.50000000000000711 ) ) ;
#4437=CARTESIAN_POINT ( 'NONE',  ( -11.31370849898482156, 11.31370849898469544, 30.00000000000000355 ) ) ;
#4438=CARTESIAN_POINT ( 'NONE',  ( -7.340858601237953529, -11.92174236212700222, 6.281673716087846415 ) ) ;
#4441=CARTESIAN_POINT ( 'NONE',  ( 14.26974319298268767, -1.607813917172876472, 20.35714285714285765 ) ) ;
#4442=CARTESIAN_POINT ( 'NONE',  ( -1.441234910513241818, -13.92619789766829008, 35.85310228751641404 ) ) ;
#4446=CARTESIAN_POINT ( 'NONE',  ( 13.25633410266679313, -4.503970704919842305, 46.56738800180214355 ) ) ;
#4450=CARTESIAN_POINT ( 'NONE',  ( 12.08964793087886314, -7.750357176954162597, 30.78975485534071765 ) ) ;
#4452=CARTESIAN_POINT ( 'NONE',  ( 11.51250119794888249, 11.69682198916847682, 39.49595943037357415 ) ) ;
#4453=CARTESIAN_POINT ( 'NONE',  ( -12.40202720642545309, 9.316290079762461929, 48.72999999999998266 ) ) ;
#4455=CARTESIAN_POINT ( 'NONE',  ( 12.22833218042443271, -7.529642458189144349, 16.78167371608784819 ) ) ;
#4459=CARTESIAN_POINT ( 'NONE',  ( 4.623906867372411078, -13.21436662431711717, 45.42857142857143060 ) ) ;
#4460=CARTESIAN_POINT ( 'NONE',  ( 10.24623928997352884, 10.06191849875416899, 5.504040569626439172 ) ) ;
#4463=CARTESIAN_POINT ( 'NONE',  ( 15.10213328493390783, -5.284464991282587398, 44.57142857142857650 ) ) ;
#4465=CARTESIAN_POINT ( 'NONE',  ( -0.06637551812352288083, 15.68265704790004023, -1.227588689168337064E-16 ) ) ;
#4468=CARTESIAN_POINT ( 'NONE',  ( -15.89939535829186923, -1.791431617653016062, 29.14285714285714235 ) ) ;
#4475=CARTESIAN_POINT ( 'NONE',  ( -13.54758718765249625, -8.512513224245459753, 40.71428571428571530 ) ) ;
#4476=( GEOMETRIC_REPRESENTATION_CONTEXT ( 3 ) GLOBAL_UNCERTAINTY_ASSIGNED_CONTEXT ( ( #8878 ) ) GLOBAL_UNIT_ASSIGNED_CONTEXT ( ( #8772, #133, #3284 ) ) REPRESENTATION_CONTEXT ( 'NONE', 'WORKASPACE' ) );
#4479=CARTESIAN_POINT ( 'NONE',  ( -1.917699372585823570, -15.88516839912900558, 25.86118342676929416 ) ) ;
#4480=CARTESIAN_POINT ( 'NONE',  ( 14.26974319298268767, -1.607813917172876916, 20.35714285714286476 ) ) ;
#4481=CARTESIAN_POINT ( 'NONE',  ( -13.54758718765249625, -8.512513224245459753, 4.714285714285712636 ) ) ;
#4482=CARTESIAN_POINT ( 'NONE',  ( 11.31370849898482334, -11.31370849898469366, 45.00000000000000711 ) ) ;
#4488=CARTESIAN_POINT ( 'NONE',  ( -9.989344678689363377, 9.809645194533960222, 7.995959430373565269 ) ) ;
#4490=CARTESIAN_POINT ( 'NONE',  ( 16.30827793483735633, -1.837501619626142890, 8.357142857142855874 ) ) ;
#4491=CARTESIAN_POINT ( 'NONE',  ( 16.30827793483735633, -1.837501619626142890, 8.357142857142855874 ) ) ;
#4493=CARTESIAN_POINT ( 'NONE',  ( -13.21436662431716869, 4.623906867372262752, 29.57142857142857650 ) ) ;
#4498=CARTESIAN_POINT ( 'NONE',  ( 4.619798703721856192, 13.59724543428036725, 45.06738800180215065 ) ) ;
#4501=CARTESIAN_POINT ( 'NONE',  ( 11.40355824106246985, -11.22385875690704538, 28.99595943037357060 ) ) ;
#4502=CARTESIAN_POINT ( 'NONE',  ( 11.31370849898482334, -11.31370849898469366, 3.000000000000002665 ) ) ;
#4504=CARTESIAN_POINT ( 'NONE',  ( -4.619798703721853528, -13.59724543428036725, 48.06738800180213644 ) ) ;
#4508=CARTESIAN_POINT ( 'NONE',  ( 1.693770420379222319, 13.89774397934251837, 34.86118342676929416 ) ) ;
#4511=CARTESIAN_POINT ( 'NONE',  ( 9.989344678689365153, -9.809645194533958446, 4.995959430373563492 ) ) ;
#4514=CARTESIAN_POINT ( 'NONE',  ( 13.51115193377584589, 4.865839792409294873, 15.92453085894499409 ) ) ;
#4518=CARTESIAN_POINT ( 'NONE',  ( -13.21436662431716869, 4.623906867372262752, 41.57142857142856940 ) ) ;
#4519=CARTESIAN_POINT ( 'NONE',  ( -14.26974319298268767, 1.607813917172874918, 47.35714285714286120 ) ) ;
#4521=CARTESIAN_POINT ( 'NONE',  ( 13.47998361472151529, 8.620103694222146729, 9.710245144659278793 ) ) ;
#4522=CARTESIAN_POINT ( 'NONE',  ( -6.162860009432963970, 14.69216993800150739, -4.192871190346624312E-15 ) ) ;
#4523=ADVANCED_FACE ( 'NONE', ( #6537 ), #9133, .T. ) ;
#4524=CARTESIAN_POINT ( 'NONE',  ( -15.10213328493390961, 5.284464991282586510, 35.57142857142857650 ) ) ;
#4532=CARTESIAN_POINT ( 'NONE',  ( 11.60466159355862104, 11.60466159355875071, 43.50000000000000711 ) ) ;
#4535=CARTESIAN_POINT ( 'NONE',  ( -15.53355953199861794, -5.297344310588530725, 20.93261199819787066 ) ) ;
#4536=CARTESIAN_POINT ( 'NONE',  ( 7.448449071214646722, 11.85413878919601594, 31.28571428571428470 ) ) ;
#4537=CARTESIAN_POINT ( 'NONE',  ( 16.30827793483735633, -1.837501619626142890, 14.35714285714285587 ) ) ;
#4538=CARTESIAN_POINT ( 'NONE',  ( -16.30827793483735988, 1.837501619626141780, 47.35714285714286120 ) ) ;
#4542=CARTESIAN_POINT ( 'NONE',  ( -8.731428362939187338, 13.89598863503036164, 48.21428571428571530 ) ) ;
#4546=CARTESIAN_POINT ( 'NONE',  ( -15.49051278174638036, -5.420364854932175902, 4.928571428571430602 ) ) ;
#4547=CARTESIAN_POINT ( 'NONE',  ( -8.621071003556675549, 13.96533075980314642, 46.21832628391216247 ) ) ;
#4551=CARTESIAN_POINT ( 'NONE',  ( 11.85413878919593422, 7.448449071214774619, 19.71428571428571175 ) ) ;
#4552=CARTESIAN_POINT ( 'NONE',  ( 4.743843029824831525, -13.17239914596749095, 47.42453085894499765 ) ) ;
#4555=CARTESIAN_POINT ( 'NONE',  ( 1.967016585148662289, -16.29368510291087091, 17.63881657323070939 ) ) ;
#4556=CARTESIAN_POINT ( 'NONE',  ( -0.3021515714675195863, 13.99673906407701729, 48.73000000000003951 ) ) ;
#4558=CARTESIAN_POINT ( 'NONE',  ( 11.51250119794888249, 11.69682198916847682, 27.49595943037356705 ) ) ;
#4562=CARTESIAN_POINT ( 'NONE',  ( 7.556039541191335474, 11.78653521626503320, 29.28975485534071765 ) ) ;
#4563=CARTESIAN_POINT ( 'NONE',  ( 15.88516839912898071, 1.917699372586004092, 46.13881657323070584 ) ) ;
#4565=CARTESIAN_POINT ( 'NONE',  ( -15.89939535829186923, -1.791431617653016062, 29.14285714285714235 ) ) ;
#4567=CARTESIAN_POINT ( 'NONE',  ( 12.22833218042443271, -7.529642458189144349, 10.78167371608784819 ) ) ;
#4571=CARTESIAN_POINT ( 'NONE',  ( -13.91197093850538380, -1.567502665446387278, 41.14285714285714590 ) ) ;
#4572=CARTESIAN_POINT ( 'NONE',  ( -7.448449071214644945, -11.85413878919601771, 46.28571428571429180 ) ) ;
#4576=CARTESIAN_POINT ( 'NONE',  ( 8.512513224245308763, 13.54758718765259040, 25.28571428571428470 ) ) ;
#4582=CARTESIAN_POINT ( 'NONE',  ( 13.61519076058348254, 8.404922754268771001, 17.71832628391214826 ) ) ;
#4583=CARTESIAN_POINT ( 'NONE',  ( 8.512513224245308763, 13.54758718765259040, 37.28571428571429180 ) ) ;
#4586=CARTESIAN_POINT ( 'NONE',  ( 15.91362231745475597, 1.665163862720026255, 18.14689771248357530 ) ) ;
#4592=CARTESIAN_POINT ( 'NONE',  ( 8.731428362939189114, -13.89598863503035986, 45.21428571428572951 ) ) ;
#4594=CARTESIAN_POINT ( 'NONE',  ( -5.164528828830334817, 15.14410076328347543, 46.43261199819787066 ) ) ;
#4596=CARTESIAN_POINT ( 'NONE',  ( 13.55419868402807992, 4.742819248065649695, 25.92857142857143060 ) ) ;
#4598=CARTESIAN_POINT ( 'NONE',  ( 13.25633410266679313, -4.503970704919842305, 34.56738800180213644 ) ) ;
#4603=CARTESIAN_POINT ( 'NONE',  ( 11.51250119794888249, 11.69682198916847682, 21.49595943037356705 ) ) ;
#4604=CARTESIAN_POINT ( 'NONE',  ( -13.89598863503045933, 8.731428362939027465, 5.785714285714282923 ) ) ;
#4606=CARTESIAN_POINT ( 'NONE',  ( 5.297344310588354865, 15.53355953199867301, 27.06738800180213644 ) ) ;
#4610=CARTESIAN_POINT ( 'NONE',  ( -10.24623928997352351, -10.06191849875416899, 44.50404056962644006 ) ) ;
#4611=CARTESIAN_POINT ( 'NONE',  ( -4.619798703721853528, -13.59724543428036725, 6.067388001802139996 ) ) ;
#4614=CARTESIAN_POINT ( 'NONE',  ( 4.743843029824831525, -13.17239914596749095, 23.42453085894499409 ) ) ;
#4618=CARTESIAN_POINT ( 'NONE',  ( 5.543385399275644332, 15.44746603149420494, 41.07546914105501656 ) ) ;
#4619=CARTESIAN_POINT ( 'NONE',  ( -13.91197093850538380, -1.567502665446387278, 47.14285714285714590 ) ) ;
#4620=CARTESIAN_POINT ( 'NONE',  ( 1.607813917173038121, -14.26974319298267346, 45.64285714285716011 ) ) ;
#4622=CARTESIAN_POINT ( 'NONE',  ( 11.40355824106246985, -11.22385875690704538, 10.99595943037356882 ) ) ;
#4624=CARTESIAN_POINT ( 'NONE',  ( -16.30827793483735988, 1.837501619626141780, 47.35714285714286120 ) ) ;
#4631=CARTESIAN_POINT ( 'NONE',  ( 5.420364854932001819, 15.49051278174644430, 43.07142857142858361 ) ) ;
#4633=CARTESIAN_POINT ( 'NONE',  ( -15.06016580658428694, 5.404401153735006957, 15.57546914105500413 ) ) ;
#4636=CARTESIAN_POINT ( 'NONE',  ( -16.30827793483735988, 1.837501619626141780, 23.35714285714286476 ) ) ;
#4639=CARTESIAN_POINT ( 'NONE',  ( 16.30827793483735633, -1.837501619626142890, 38.35714285714286831 ) ) ;
#4645=CARTESIAN_POINT ( 'NONE',  ( -1.707986654103994528, 16.32287076676380266, 46.64689771248358596 ) ) ;
#4647=CARTESIAN_POINT ( 'NONE',  ( -14.26974319298268767, 1.607813917172874696, 29.35714285714286120 ) ) ;
#4651=CARTESIAN_POINT ( 'NONE',  ( 1.441234910513245149, 13.92619789766829008, 38.85310228751641404 ) ) ;
#4653=FACE_OUTER_BOUND ( 'NONE', #1800, .T. ) ;
#4654=CARTESIAN_POINT ( 'NONE',  ( -15.44746603149413922, -5.543385399275820191, 24.92453085894499765 ) ) ;
#4655=CARTESIAN_POINT ( 'NONE',  ( 8.731428362939189114, -13.89598863503035986, 9.214285714285717077 ) ) ;
#4656=CARTESIAN_POINT ( 'NONE',  ( 11.40355824106246985, -11.22385875690704538, 22.99595943037356705 ) ) ;
#4662=CARTESIAN_POINT ( 'NONE',  ( 7.340858601237956194, 11.92174236212700045, 9.281673716087846415 ) ) ;
#4665=CARTESIAN_POINT ( 'NONE',  ( -10.06191849875405531, -10.24623928997363542, 30.49595943037356349 ) ) ;
#4669=CARTESIAN_POINT ( 'NONE',  ( -1.707986654103994528, 16.32287076676380266, 46.64689771248358596 ) ) ;
#4670=CARTESIAN_POINT ( 'NONE',  ( -4.503970704919988854, 13.25633410266674517, 4.432611998197859116 ) ) ;
#4672=CARTESIAN_POINT ( 'NONE',  ( -7.529642458189277576, 12.22833218042435455, 4.218326283912150032 ) ) ;
#4674=CARTESIAN_POINT ( 'NONE',  ( -13.47998361472151174, -8.620103694222146729, 12.71024514465927879 ) ) ;
#4676=CARTESIAN_POINT ( 'NONE',  ( 15.89939535829187278, 1.791431617653015174, 38.14285714285714590 ) ) ;
#4685=CARTESIAN_POINT ( 'NONE',  ( -11.22385875690717327, 11.40355824106234550, 22.00404056962643651 ) ) ;
#4686=CARTESIAN_POINT ( 'NONE',  ( 5.420364854932001819, 15.49051278174644430, 13.07142857142857295 ) ) ;
#4688=CARTESIAN_POINT ( 'NONE',  ( 8.731428362939190890, -13.89598863503036164, 3.214285714285716633 ) ) ;
#4689=CARTESIAN_POINT ( 'NONE',  ( 11.31370849898482334, -11.31370849898469366, 39.00000000000000000 ) ) ;
#4692=CIRCLE ( 'NONE', #234, 1.000000000000000000 ) ;
#4694=CARTESIAN_POINT ( 'NONE',  ( -16.30827793483735988, 1.837501619626141780, 5.357142857142856762 ) ) ;
#4696=CARTESIAN_POINT ( 'NONE',  ( 14.26974319298268767, -1.607813917172876472, 32.35714285714286120 ) ) ;
#4697=CARTESIAN_POINT ( 'NONE',  ( 12.08964793087886314, -7.750357176954162597, 30.78975485534071765 ) ) ;
#4701=CARTESIAN_POINT ( 'NONE',  ( -7.639999817571787588, 12.15899005565156266, 0.2142857142857168273 ) ) ;
#4703=CARTESIAN_POINT ( 'NONE',  ( -15.14410076328353227, 5.164528828830164287, 19.56738800180213644 ) ) ;
#4704=CARTESIAN_POINT ( 'NONE',  ( 15.10213328493390783, -5.284464991282587398, 2.571428571428571619 ) ) ;
#4705=CARTESIAN_POINT ( 'NONE',  ( -8.404922754268618235, -13.61519076058357491, 30.28167371608785530 ) ) ;
#4708=CARTESIAN_POINT ( 'NONE',  ( -7.448449071214644945, -11.85413878919601771, 4.285714285714288252 ) ) ;
#4711=CARTESIAN_POINT ( 'NONE',  ( -5.404401153735176599, 15.06016580658422477, 50.42453085894499765 ) ) ;
#4714=CARTESIAN_POINT ( 'NONE',  ( -11.60466159355861926, -11.60466159355875249, 10.50000000000000533 ) ) ;
#4716=CARTESIAN_POINT ( 'NONE',  ( -9.989344678689363377, 9.809645194533960222, 31.99595943037357060 ) ) ;
#4721=CARTESIAN_POINT ( 'NONE',  ( 7.556039541191335474, 11.78653521626503320, 11.28975485534071943 ) ) ;
#4722=CARTESIAN_POINT ( 'NONE',  ( -1.693770420379220099, -13.89774397934251837, 13.86118342676929416 ) ) ;
#4724=CARTESIAN_POINT ( 'NONE',  ( -5.297344310588352201, -15.53355953199867301, 6.067388001802139996 ) ) ;
#4726=CARTESIAN_POINT ( 'NONE',  ( -15.49051278174638036, -5.420364854932175902, 40.92857142857145192 ) ) ;
#4732=CARTESIAN_POINT ( 'NONE',  ( -15.53355953199861794, -5.297344310588530725, 32.93261199819787777 ) ) ;
#4734=CARTESIAN_POINT ( 'NONE',  ( -8.620103694221995738, -13.47998361472161299, 32.28975485534072476 ) ) ;
#4735=CARTESIAN_POINT ( 'NONE',  ( -16.30827793483735988, 1.837501619626141780, 17.35714285714286476 ) ) ;
#4744=CARTESIAN_POINT ( 'NONE',  ( 4.503970704919991519, -13.25633410266674517, 43.43261199819787066 ) ) ;
#4745=CARTESIAN_POINT ( 'NONE',  ( -8.512513224245306986, -13.54758718765259218, 16.28571428571428470 ) ) ;
#4747=CARTESIAN_POINT ( 'NONE',  ( -1.567502665446231180, -13.91197093850540334, 39.85714285714286120 ) ) ;
#4748=CARTESIAN_POINT ( 'NONE',  ( 11.92174236212692229, 7.340858601238088532, 35.71832628391214115 ) ) ;
#4752=CARTESIAN_POINT ( 'NONE',  ( 13.55419868402807992, 4.742819248065648807, 1.928571428571430380 ) ) ;
#4755=CARTESIAN_POINT ( 'NONE',  ( -15.88516839912898071, -1.917699372586004980, 31.13881657323070939 ) ) ;
#4757=CARTESIAN_POINT ( 'NONE',  ( -8.731428362939187338, 13.89598863503036164, 18.21428571428572241 ) ) ;
#4758=CARTESIAN_POINT ( 'NONE',  ( 8.404922754268618235, 13.61519076058357491, 21.28167371608785530 ) ) ;
#4765=CARTESIAN_POINT ( 'NONE',  ( -1.737328882695368115, 14.25515036105620581, 26.63881657323070939 ) ) ;
#4769=CARTESIAN_POINT ( 'NONE',  ( -13.92619789766827054, -1.441234910513399470, 3.146897712483577969 ) ) ;
#4770=CARTESIAN_POINT ( 'NONE',  ( 7.529642458189280241, -12.22833218042435099, 7.218326283912148256 ) ) ;
#4773=CARTESIAN_POINT ( 'NONE',  ( 11.31370849898469899, 11.31370849898481978, 49.50000000000000711 ) ) ;
#4774=DIRECTION ( 'NONE',  ( 0.7071067811865431318, 0.7071067811865519026, -7.359808400080253795E-17 ) ) ;
#4780=CARTESIAN_POINT ( 'NONE',  ( 11.69682198916835070, 11.51250119794901394, 29.50404056962643295 ) ) ;
#4783=CARTESIAN_POINT ( 'NONE',  ( 1.791431617652837316, 15.89939535829188877, 30.85714285714286120 ) ) ;
#4785=CARTESIAN_POINT ( 'NONE',  ( 13.54758718765249803, 8.512513224245457977, 7.714285714285715301 ) ) ;
#4788=CARTESIAN_POINT ( 'NONE',  ( -5.543385399275643444, -15.44746603149420494, 2.075469141055009015 ) ) ;
#4790=CARTESIAN_POINT ( 'NONE',  ( -5.284464991282755264, 15.10213328493384743, 12.42857142857142705 ) ) ;
#4793=CARTESIAN_POINT ( 'NONE',  ( -4.623906867372410190, 13.21436662431711895, 42.42857142857143060 ) ) ;
#4794=CARTESIAN_POINT ( 'NONE',  ( 7.529642458189280241, -12.22833218042435099, 37.21832628391215536 ) ) ;
#4795=CARTESIAN_POINT ( 'NONE',  ( -7.556039541191334585, -11.78653521626503320, 32.28975485534072476 ) ) ;
#4799=CARTESIAN_POINT ( 'NONE',  ( 1.607813917173038121, -14.26974319298267346, 3.642857142857144126 ) ) ;
#4804=CARTESIAN_POINT ( 'NONE',  ( 15.49051278174637858, 5.420364854932174126, 19.92857142857143415 ) ) ;
#4805=CARTESIAN_POINT ( 'NONE',  ( -8.404922754268618235, -13.61519076058357491, 42.28167371608785174 ) ) ;
#4810=SURFACE_STYLE_FILL_AREA ( #153 ) ;
#4812=CARTESIAN_POINT ( 'NONE',  ( -14.28433602490915000, 1.478298951650542481, 19.35310228751642825 ) ) ;
#4816=CARTESIAN_POINT ( 'NONE',  ( 11.78653521626494793, 7.556039541191463371, 27.71024514465928235 ) ) ;
#4820=CARTESIAN_POINT ( 'NONE',  ( -7.529642458189277576, 12.22833218042435455, 4.218326283912150032 ) ) ;
#4821=CARTESIAN_POINT ( 'NONE',  ( -14.25515036105622890, 1.737328882695209575, 15.36118342676929771 ) ) ;
#4824=CARTESIAN_POINT ( 'NONE',  ( -15.10213328493390961, 5.284464991282586510, 41.57142857142856940 ) ) ;
#4830=CARTESIAN_POINT ( 'NONE',  ( 5.164528828830335705, -15.14410076328347543, 25.43261199819786711 ) ) ;
#4832=CARTESIAN_POINT ( 'NONE',  ( 16.29368510291089223, -1.967016585148476882, 30.36118342676929771 ) ) ;
#4834=CARTESIAN_POINT ( 'NONE',  ( -13.89598863503046111, 8.731428362939027465, 35.78571428571429180 ) ) ;
#4835=CARTESIAN_POINT ( 'NONE',  ( 3.908916549244207506, 14.54798010869238567, 2.434022981070398982E-13 ) ) ;
#4837=CARTESIAN_POINT ( 'NONE',  ( 8.512513224245308763, 13.54758718765259040, 1.285714285714285809 ) ) ;
#4843=CARTESIAN_POINT ( 'NONE',  ( 11.22385875690717683, -11.40355824106234373, 1.004040569626440726 ) ) ;
#4844=CARTESIAN_POINT ( 'NONE',  ( 11.31370849898482334, -11.31370849898469366, 21.00000000000000355 ) ) ;
#4845=CARTESIAN_POINT ( 'NONE',  ( 9.899494936611718643, -9.899494936611608509, 33.00000000000000000 ) ) ;
#4846=CARTESIAN_POINT ( 'NONE',  ( 12.08964793087886314, -7.750357176954162597, 36.78975485534072476 ) ) ;
#4847=CARTESIAN_POINT ( 'NONE',  ( 1.567502665446232957, 13.91197093850540156, 6.857142857142860315 ) ) ;
#4851=CARTESIAN_POINT ( 'NONE',  ( 7.448449071214646722, 11.85413878919601594, 7.285714285714284699 ) ) ;
#4855=CARTESIAN_POINT ( 'NONE',  ( -1.837501619626327853, 16.30827793483733856, 12.64285714285714235 ) ) ;
#4857=CARTESIAN_POINT ( 'NONE',  ( 15.14410076328353227, -5.164528828830166063, 34.56738800180213644 ) ) ;
#4860=CARTESIAN_POINT ( 'NONE',  ( 13.55419868402807992, 4.742819248065649695, 1.928571428571430380 ) ) ;
#4863=CARTESIAN_POINT ( 'NONE',  ( -7.340858601237953529, -11.92174236212700222, 12.28167371608784997 ) ) ;
#4865=CARTESIAN_POINT ( 'NONE',  ( 1.837501619626330074, -16.30827793483733501, 9.642857142857147679 ) ) ;
#4867=CARTESIAN_POINT ( 'NONE',  ( 5.420364854932001819, 15.49051278174644430, 37.07142857142857650 ) ) ;
#4868=CARTESIAN_POINT ( 'NONE',  ( 7.340858601237956194, 11.92174236212700045, 33.28167371608784464 ) ) ;
#4872=CARTESIAN_POINT ( 'NONE',  ( 12.08964793087886314, -7.750357176954162597, 6.789754855340717654 ) ) ;
#4874=CARTESIAN_POINT ( 'NONE',  ( 4.503970704919991519, -13.25633410266674517, 7.432611998197861780 ) ) ;
#4878=CARTESIAN_POINT ( 'NONE',  ( 1.967016585148662289, -16.29368510291087091, 11.63881657323070939 ) ) ;
#4884=CARTESIAN_POINT ( 'NONE',  ( 11.22385875690717683, -11.40355824106234373, 25.00404056962644006 ) ) ;
#4886=CARTESIAN_POINT ( 'NONE',  ( -15.06016580658428694, 5.404401153735006957, 33.57546914105500946 ) ) ;
#4888=CARTESIAN_POINT ( 'NONE',  ( 13.89598863503046111, -8.731428362939032795, 32.78571428571430602 ) ) ;
#4889=CARTESIAN_POINT ( 'NONE',  ( 3.436234746893573444, 14.87838136757911656, 2.020632658447805774E-13 ) ) ;
#4890=CARTESIAN_POINT ( 'NONE',  ( 5.420364854932001819, 15.49051278174644430, 7.071428571428569398 ) ) ;
#4894=CARTESIAN_POINT ( 'NONE',  ( 8.620103694221997515, 13.47998361472160767, -0.7102451446592792372 ) ) ;
#4895=CARTESIAN_POINT ( 'NONE',  ( -11.31370849898482156, 11.31370849898469544, 11.99999999999999645 ) ) ;
#4896=CARTESIAN_POINT ( 'NONE',  ( -14.26974319298268767, 1.607813917172874696, 41.35714285714286120 ) ) ;
#4897=CARTESIAN_POINT ( 'NONE',  ( -9.809645194534070356, 9.989344678689256796, 40.00404056962644006 ) ) ;
#4898=CARTESIAN_POINT ( 'NONE',  ( 13.55419868402807992, 4.742819248065648807, 13.92857142857143238 ) ) ;
#4902=CARTESIAN_POINT ( 'NONE',  ( -7.448449071214644945, -11.85413878919601771, 4.285714285714288252 ) ) ;
#4906=CARTESIAN_POINT ( 'NONE',  ( -5.420364854931998266, -15.49051278174643898, 22.07142857142858006 ) ) ;
#4907=CARTESIAN_POINT ( 'NONE',  ( 15.14410076328353227, -5.164528828830166063, 40.56738800180214355 ) ) ;
#4910=CARTESIAN_POINT ( 'NONE',  ( 7.639999817571788476, -12.15899005565156266, 3.214285714285716633 ) ) ;
#4911=AXIS2_PLACEMENT_3D ( 'NONE', #3043, #8576, #7806 ) ;
#4913=CARTESIAN_POINT ( 'NONE',  ( 11.78653521626494793, 7.556039541191463371, 9.710245144659278793 ) ) ;
#4915=CARTESIAN_POINT ( 'NONE',  ( -13.54758718765249625, -8.512513224245459753, 10.71428571428571708 ) ) ;
#4918=CARTESIAN_POINT ( 'NONE',  ( -5.284464991282755264, 15.10213328493384743, 36.42857142857143060 ) ) ;
#4919=CARTESIAN_POINT ( 'NONE',  ( 7.750357176954296712, -12.08964793087877787, 35.21024514465927524 ) ) ;
#4923=CARTESIAN_POINT ( 'NONE',  ( 10.24623928997352884, 10.06191849875416899, 23.50404056962643295 ) ) ;
#4924=CARTESIAN_POINT ( 'NONE',  ( 4.865839792409144771, 13.51115193377589740, 11.07546914105500768 ) ) ;
#4925=CARTESIAN_POINT ( 'NONE',  ( -0.9669241168434388189, 13.98238843080921079, 48.73000000000005372 ) ) ;
#4926=CARTESIAN_POINT ( 'NONE',  ( 15.14410076328353227, -5.164528828830166063, 10.56738800180213644 ) ) ;
#4933=CARTESIAN_POINT ( 'NONE',  ( 13.61519076058348254, 8.404922754268771001, 29.71832628391214826 ) ) ;
#4934=CARTESIAN_POINT ( 'NONE',  ( -4.742819248065502258, -13.55419868402813677, 34.07142857142859071 ) ) ;
#4935=CARTESIAN_POINT ( 'NONE',  ( 15.06016580658428694, -5.404401153735007846, 36.57546914105501656 ) ) ;
#4937=CARTESIAN_POINT ( 'NONE',  ( -1.791431617652833763, -15.89939535829188877, 33.85714285714285410 ) ) ;
#4938=CARTESIAN_POINT ( 'NONE',  ( -9.899494936611716867, 9.899494936611610285, 0.000000000000000000 ) ) ;
#4939=CARTESIAN_POINT ( 'NONE',  ( -11.60466159355861926, -11.60466159355875249, 22.50000000000000000 ) ) ;
#4944=CARTESIAN_POINT ( 'NONE',  ( 1.478298951650704351, -14.28433602490913579, 43.64689771248358596 ) ) ;
#4945=CARTESIAN_POINT ( 'NONE',  ( 11.31370849898482334, -11.31370849898469366, 33.00000000000000000 ) ) ;
#4947=CARTESIAN_POINT ( 'NONE',  ( 9.809645194534072132, -9.989344678689256796, 43.00404056962644717 ) ) ;
#4949=CARTESIAN_POINT ( 'NONE',  ( 15.89939535829187278, 1.791431617653015174, 38.14285714285714590 ) ) ;
#4953=CARTESIAN_POINT ( 'NONE',  ( 9.899494936611718643, -9.899494936611608509, 21.00000000000000355 ) ) ;
#4956=CARTESIAN_POINT ( 'NONE',  ( 8.731428362939189114, -13.89598863503035986, 21.21428571428571530 ) ) ;
#4958=CARTESIAN_POINT ( 'NONE',  ( 5.404401153735178376, -15.06016580658422477, 41.42453085894499765 ) ) ;
#4961=CARTESIAN_POINT ( 'NONE',  ( -9.899494936611716867, 9.899494936611610285, 18.00000000000000355 ) ) ;
#4965=CARTESIAN_POINT ( 'NONE',  ( 13.51115193377584589, 4.865839792409294873, 15.92453085894499409 ) ) ;
#4970=CARTESIAN_POINT ( 'NONE',  ( 13.25633410266679313, -4.503970704919842305, 40.56738800180214355 ) ) ;
#4975=CARTESIAN_POINT ( 'NONE',  ( 11.92174236212692229, 7.340858601238088532, 17.71832628391214826 ) ) ;
#4976=CARTESIAN_POINT ( 'NONE',  ( -7.529642458189277576, 12.22833218042435455, 22.21832628391215181 ) ) ;
#4978=CARTESIAN_POINT ( 'NONE',  ( 8.841785722321695573, -13.82664651025757152, 5.210245144659280569 ) ) ;
#4985=CARTESIAN_POINT ( 'NONE',  ( -11.22385875690717327, 11.40355824106234550, 40.00404056962644006 ) ) ;
#4987=CARTESIAN_POINT ( 'NONE',  ( -7.448449071214644945, -11.85413878919601771, 28.28571428571428825 ) ) ;
#4988=CARTESIAN_POINT ( 'NONE',  ( 15.91362231745475597, 1.665163862720026255, 42.14689771248358596 ) ) ;
#4990=CARTESIAN_POINT ( 'NONE',  ( -11.60466159355861926, -11.60466159355875249, 34.50000000000000000 ) ) ;
#4991=CARTESIAN_POINT ( 'NONE',  ( 2.601377816629832473, 14.36985073060440499, 7.004981435163793185E-16 ) ) ;
#4992=CARTESIAN_POINT ( 'NONE',  ( 11.31370849898482334, -11.31370849898469366, 21.00000000000000355 ) ) ;
#4996=CARTESIAN_POINT ( 'NONE',  ( -15.91362231745475597, -1.665163862720028254, 15.14689771248357708 ) ) ;
#4997=CARTESIAN_POINT ( 'NONE',  ( 15.10213328493390783, -5.284464991282587398, 32.57142857142856940 ) ) ;
#4998=CARTESIAN_POINT ( 'NONE',  ( 13.61519076058348254, 8.404922754268771001, 5.718326283912152697 ) ) ;
#5000=CARTESIAN_POINT ( 'NONE',  ( 11.85413878919593422, 7.448449071214774619, 7.714285714285715301 ) ) ;
#5004=CARTESIAN_POINT ( 'NONE',  ( -13.21436662431716869, 4.623906867372262752, 17.57142857142856940 ) ) ;
#5006=CARTESIAN_POINT ( 'NONE',  ( 1.837501619626329630, -16.30827793483733501, 27.64285714285714590 ) ) ;
#5007=CARTESIAN_POINT ( 'NONE',  ( 16.32287076676382043, -1.707986654103810897, 34.35310228751642825 ) ) ;
#5010=CARTESIAN_POINT ( 'NONE',  ( 7.448449071214646722, 11.85413878919601594, 7.285714285714284699 ) ) ;
#5011=CARTESIAN_POINT ( 'NONE',  ( -4.743843029824828861, 13.17239914596749450, 26.42453085894499765 ) ) ;
#5015=CARTESIAN_POINT ( 'NONE',  ( -10.06191849875405531, -10.24623928997363542, 42.49595943037355994 ) ) ;
#5020=CARTESIAN_POINT ( 'NONE',  ( -11.92174236212692051, -7.340858601238089420, 20.71832628391214826 ) ) ;
#5022=CARTESIAN_POINT ( 'NONE',  ( -7.556039541191334585, -11.78653521626503320, 26.28975485534072831 ) ) ;
#5024=CARTESIAN_POINT ( 'NONE',  ( -1.665163862719845067, -15.91362231745477374, 41.85310228751642825 ) ) ;
#5026=CARTESIAN_POINT ( 'NONE',  ( -2.927791565357304115, 15.72098899558116436, 48.73000000000027399 ) ) ;
#5027=CARTESIAN_POINT ( 'NONE',  ( -1.837501619626328297, 16.30827793483733856, 18.64285714285715656 ) ) ;
#5028=CARTESIAN_POINT ( 'NONE',  ( -15.44746603149413922, -5.543385399275820191, 12.92453085894499587 ) ) ;
#5034=CARTESIAN_POINT ( 'NONE',  ( -16.29368510291090288, 1.967016585148476215, 33.36118342676929416 ) ) ;
#5035=CARTESIAN_POINT ( 'NONE',  ( -1.567502665446231180, -13.91197093850540334, 33.85714285714285410 ) ) ;
#5036=CARTESIAN_POINT ( 'NONE',  ( 13.91197093850538380, 1.567502665446386390, 38.14285714285714590 ) ) ;
#5038=CARTESIAN_POINT ( 'NONE',  ( -5.284464991282755264, 15.10213328493384743, 48.42857142857143060 ) ) ;
#5040=CARTESIAN_POINT ( 'NONE',  ( 5.284464991282756152, -15.10213328493384743, 21.42857142857142705 ) ) ;
#5045=CARTESIAN_POINT ( 'NONE',  ( -13.61519076058348254, -8.404922754268771001, 8.718326283912148256 ) ) ;
#5046=CARTESIAN_POINT ( 'NONE',  ( -11.60466159355861926, -11.60466159355875249, 28.50000000000001066 ) ) ;
#5048=CARTESIAN_POINT ( 'NONE',  ( -8.620103694221995738, -13.47998361472161299, 2.289754855340722539 ) ) ;
#5049=CARTESIAN_POINT ( 'NONE',  ( -11.85413878919593422, -7.448449071214776396, 16.71428571428571530 ) ) ;
#5053=CARTESIAN_POINT ( 'NONE',  ( -7.639999817571787588, 12.15899005565156266, 18.21428571428571885 ) ) ;
#5055=CARTESIAN_POINT ( 'NONE',  ( -5.420364854931998266, -15.49051278174643898, 34.07142857142857650 ) ) ;
#5056=CARTESIAN_POINT ( 'NONE',  ( 11.40355824106246985, -11.22385875690704538, 46.99595943037356705 ) ) ;
#5058=CARTESIAN_POINT ( 'NONE',  ( -7.639999817571786700, 12.15899005565156266, 6.214285714285717077 ) ) ;
#5059=CARTESIAN_POINT ( 'NONE',  ( 1.737328882695370558, -14.25515036105620581, 23.63881657323070939 ) ) ;
#5063=CARTESIAN_POINT ( 'NONE',  ( 4.619798703721856192, 13.59724543428036725, 33.06738800180213644 ) ) ;
#5067=CARTESIAN_POINT ( 'NONE',  ( -9.809645194534070356, 9.989344678689256796, 16.00404056962643651 ) ) ;
#5068=CARTESIAN_POINT ( 'NONE',  ( -10.24623928997352351, -10.06191849875416899, 26.50404056962643651 ) ) ;
#5070=CARTESIAN_POINT ( 'NONE',  ( 15.14410076328353227, -5.164528828830166063, 34.56738800180213644 ) ) ;
#5071=CARTESIAN_POINT ( 'NONE',  ( -12.72000065966944504, 8.744481972363274735, 48.72999999999997556 ) ) ;
#5072=CARTESIAN_POINT ( 'NONE',  ( 13.89598863503046111, -8.731428362939032795, 20.78571428571429180 ) ) ;
#5073=CARTESIAN_POINT ( 'NONE',  ( -1.665163862719845067, -15.91362231745477374, 11.85310228751642470 ) ) ;
#5075=( GEOMETRIC_REPRESENTATION_CONTEXT ( 3 ) GLOBAL_UNCERTAINTY_ASSIGNED_CONTEXT ( ( #5958 ) ) GLOBAL_UNIT_ASSIGNED_CONTEXT ( ( #1611, #2430, #3155 ) ) REPRESENTATION_CONTEXT ( 'NONE', 'WORKASPACE' ) );
#5079=CARTESIAN_POINT ( 'NONE',  ( 4.742819248065503146, 13.55419868402813677, 37.07142857142857650 ) ) ;
#5080=CARTESIAN_POINT ( 'NONE',  ( 10.15407889436379030, 10.15407889436390576, 37.50000000000002842 ) ) ;
#5083=CARTESIAN_POINT ( 'NONE',  ( 8.512513224245308763, 13.54758718765259040, 49.28571428571428470 ) ) ;
#5085=CARTESIAN_POINT ( 'NONE',  ( 16.30827793483735633, -1.837501619626142890, 14.35714285714285587 ) ) ;
#5092=CARTESIAN_POINT ( 'NONE',  ( -11.22385875690717327, 11.40355824106234550, 16.00404056962643651 ) ) ;
#5093=CARTESIAN_POINT ( 'NONE',  ( -13.54758718765249625, -8.512513224245459753, 34.71428571428571530 ) ) ;
#5095=CARTESIAN_POINT ( 'NONE',  ( -13.61519076058348254, -8.404922754268771001, 8.718326283912148256 ) ) ;
#5096=CARTESIAN_POINT ( 'NONE',  ( 7.639999817571789364, -12.15899005565156266, 21.21428571428571885 ) ) ;
#5097=CARTESIAN_POINT ( 'NONE',  ( -16.30827793483735988, 1.837501619626141780, 11.35714285714285943 ) ) ;
#5100=CARTESIAN_POINT ( 'NONE',  ( 13.55419868402807992, 4.742819248065648807, 19.92857142857143771 ) ) ;
#5102=CARTESIAN_POINT ( 'NONE',  ( 8.731428362939189114, -13.89598863503035986, 33.21428571428571530 ) ) ;
#5103=CARTESIAN_POINT ( 'NONE',  ( -12.22833218042443271, 7.529642458189139909, 7.781673716087849968 ) ) ;
#5106=CARTESIAN_POINT ( 'NONE',  ( 13.21436662431716869, -4.623906867372263640, 8.571428571428569398 ) ) ;
#5108=CARTESIAN_POINT ( 'NONE',  ( -10.06191849875405531, -10.24623928997363542, 24.49595943037356705 ) ) ;
#5113=CARTESIAN_POINT ( 'NONE',  ( 13.55419868402807992, 4.742819248065648807, 1.928571428571430380 ) ) ;
#5117=CARTESIAN_POINT ( 'NONE',  ( 7.556039541191335474, 11.78653521626503320, 35.28975485534072476 ) ) ;
#5121=CARTESIAN_POINT ( 'NONE',  ( -1.478298951650703019, 14.28433602490913579, 28.64689771248357886 ) ) ;
#5124=CARTESIAN_POINT ( 'NONE',  ( 15.88516839912898071, 1.917699372586004092, 34.13881657323070584 ) ) ;
#5125=CARTESIAN_POINT ( 'NONE',  ( -13.17294599347781769, 7.596107530180142398, 48.73000000000000398 ) ) ;
#5126=CARTESIAN_POINT ( 'NONE',  ( -8.731428362939189114, 13.89598863503036341, 24.21428571428571530 ) ) ;
#5133=CARTESIAN_POINT ( 'NONE',  ( 13.25633410266679313, -4.503970704919842305, 10.56738800180213644 ) ) ;
#5137=CARTESIAN_POINT ( 'NONE',  ( -9.899494936611716867, 9.899494936611610285, 30.00000000000000355 ) ) ;
#5139=CARTESIAN_POINT ( 'NONE',  ( 9.899494936611718643, -9.899494936611608509, 33.00000000000000000 ) ) ;
#5141=CARTESIAN_POINT ( 'NONE',  ( -8.731428362939189114, 13.89598863503036341, 48.21428571428570820 ) ) ;
#5143=CARTESIAN_POINT ( 'NONE',  ( 5.420364854932001819, 15.49051278174644430, 19.07142857142856940 ) ) ;
#5149=CARTESIAN_POINT ( 'NONE',  ( 11.69682198916835070, 11.51250119794901394, 11.50404056962644006 ) ) ;
#5150=CARTESIAN_POINT ( 'NONE',  ( 13.89598863503046111, -8.731428362939032795, 26.78571428571429536 ) ) ;
#5152=CARTESIAN_POINT ( 'NONE',  ( 16.29368510291089223, -1.967016585148476882, 12.36118342676929771 ) ) ;
#5153=CARTESIAN_POINT ( 'NONE',  ( -4.623906867372410190, 13.21436662431711895, 30.42857142857143060 ) ) ;
#5155=CARTESIAN_POINT ( 'NONE',  ( 15.10213328493390783, -5.284464991282587398, 2.571428571428571619 ) ) ;
#5156=CARTESIAN_POINT ( 'NONE',  ( 1.791431617652837316, 15.89939535829188877, 42.85714285714285410 ) ) ;
#5158=CARTESIAN_POINT ( 'NONE',  ( 12.15899005565164792, -7.639999817571655250, 20.78571428571429180 ) ) ;
#5160=CARTESIAN_POINT ( 'NONE',  ( 5.284464991282756152, -15.10213328493384743, 27.42857142857143060 ) ) ;
#5161=CARTESIAN_POINT ( 'NONE',  ( 11.78653521626494793, 7.556039541191463371, 3.710245144659281458 ) ) ;
#5164=CARTESIAN_POINT ( 'NONE',  ( -4.742819248065500481, -13.55419868402813499, 16.07142857142857650 ) ) ;
#5165=EDGE_CURVE ( 'NONE', #7090, #3093, #8606, .T. ) ;
#5166=CARTESIAN_POINT ( 'NONE',  ( 11.78653521626494793, 7.556039541191463371, 27.71024514465928235 ) ) ;
#5170=CARTESIAN_POINT ( 'NONE',  ( -9.899494936611716867, 9.899494936611610285, 0.000000000000000000 ) ) ;
#5172=CARTESIAN_POINT ( 'NONE',  ( 7.639999817571789364, -12.15899005565156266, 3.214285714285716633 ) ) ;
#5176=CARTESIAN_POINT ( 'NONE',  ( 13.59724543428031573, 4.619798703722006294, 29.93261199819786356 ) ) ;
#5179=CARTESIAN_POINT ( 'NONE',  ( -16.32287076676382398, 1.707986654103809343, 37.35310228751641404 ) ) ;
#5182=CARTESIAN_POINT ( 'NONE',  ( 4.619798703721856192, 13.59724543428036725, 15.06738800180213822 ) ) ;
#5186=CARTESIAN_POINT ( 'NONE',  ( 13.21436662431716869, -4.623906867372263640, 38.57142857142857650 ) ) ;
#5188=CARTESIAN_POINT ( 'NONE',  ( 4.742819248065503146, 13.55419868402813677, 37.07142857142857650 ) ) ;
#5189=ORIENTED_EDGE ( 'NONE', *, *, #6503, .F. ) ;
#5190=CARTESIAN_POINT ( 'NONE',  ( -15.10213328493390961, 5.284464991282586510, 47.57142857142857650 ) ) ;
#5192=CARTESIAN_POINT ( 'NONE',  ( 15.10213328493390783, -5.284464991282587398, 32.57142857142856940 ) ) ;
#5199=CARTESIAN_POINT ( 'NONE',  ( 13.82664651025767100, -8.841785722321541030, 12.78975485534072121 ) ) ;
#5200=CARTESIAN_POINT ( 'NONE',  ( -5.420364854931999155, -15.49051278174644253, 40.07142857142857650 ) ) ;
#5202=CARTESIAN_POINT ( 'NONE',  ( 15.53355953199861794, 5.297344310588528060, 5.932611998197868886 ) ) ;
#5203=CARTESIAN_POINT ( 'NONE',  ( -1.791431617652833763, -15.89939535829188877, 3.857142857142857650 ) ) ;
#5204=CARTESIAN_POINT ( 'NONE',  ( 13.89598863503046111, -8.731428362939032795, 44.78571428571428470 ) ) ;
#5208=CARTESIAN_POINT ( 'NONE',  ( -1.837501619626327853, 16.30827793483733856, 24.64285714285714235 ) ) ;
#5209=CARTESIAN_POINT ( 'NONE',  ( 1.441234910513245149, 13.92619789766829008, 2.853102287516426916 ) ) ;
#5212=CARTESIAN_POINT ( 'NONE',  ( 7.639999817571788476, -12.15899005565156266, 27.21428571428571885 ) ) ;
#5214=CARTESIAN_POINT ( 'NONE',  ( -14.28433602490915000, 1.478298951650542481, 31.35310228751642470 ) ) ;
#5221=CARTESIAN_POINT ( 'NONE',  ( -1.693770420379220099, -13.89774397934251837, 25.86118342676929416 ) ) ;
#5223=CARTESIAN_POINT ( 'NONE',  ( 1.967016585148662289, -16.29368510291087091, 35.63881657323071295 ) ) ;
#5224=CARTESIAN_POINT ( 'NONE',  ( -13.04911192085559790, 7.214667598204639987, 48.73000000000001819 ) ) ;
#5226=CARTESIAN_POINT ( 'NONE',  ( -13.51115193377584589, -4.865839792409295761, 18.92453085894499409 ) ) ;
#5230=CARTESIAN_POINT ( 'NONE',  ( 13.21436662431716869, -4.623906867372263640, 44.57142857142857650 ) ) ;
#5231=CARTESIAN_POINT ( 'NONE',  ( 7.556039541191335474, 11.78653521626503320, 5.289754855340725648 ) ) ;
#5233=CARTESIAN_POINT ( 'NONE',  ( -1.837501619626328297, 16.30827793483733856, 42.64285714285715301 ) ) ;
#5235=CARTESIAN_POINT ( 'NONE',  ( -1.837501619626328297, 16.30827793483733856, 30.64285714285715301 ) ) ;
#5242=CARTESIAN_POINT ( 'NONE',  ( 1.837501619626330074, -16.30827793483733501, 39.64285714285716722 ) ) ;
#5243=CARTESIAN_POINT ( 'NONE',  ( 13.82664651025767100, -8.841785722321541030, 24.78975485534072476 ) ) ;
#5244=CARTESIAN_POINT ( 'NONE',  ( 1.567502665446232957, 13.91197093850540156, 24.85714285714285765 ) ) ;
#5246=CARTESIAN_POINT ( 'NONE',  ( -15.10213328493390961, 5.284464991282586510, 41.57142857142856940 ) ) ;
#5251=CARTESIAN_POINT ( 'NONE',  ( 1.737328882695370558, -14.25515036105620581, 5.638816573230711171 ) ) ;
#5253=CARTESIAN_POINT ( 'NONE',  ( 15.89939535829187278, 1.791431617653015174, 8.142857142857145902 ) ) ;
#5254=CARTESIAN_POINT ( 'NONE',  ( 5.420364854932001819, 15.49051278174644430, 7.071428571428569398 ) ) ;
#5255=CARTESIAN_POINT ( 'NONE',  ( -7.639999817571786700, 12.15899005565156266, 24.21428571428571530 ) ) ;
#5256=CARTESIAN_POINT ( 'NONE',  ( 13.51115193377584589, 4.865839792409294873, 39.92453085894499054 ) ) ;
#5259=CARTESIAN_POINT ( 'NONE',  ( -5.404401153735176599, 15.06016580658422477, 20.42453085894499054 ) ) ;
#5260=CARTESIAN_POINT ( 'NONE',  ( -13.54758718765249625, -8.512513224245459753, 10.71428571428571708 ) ) ;
#5265=CARTESIAN_POINT ( 'NONE',  ( -4.503970704919988854, 13.25633410266674517, 34.43261199819786356 ) ) ;
#5269=CARTESIAN_POINT ( 'NONE',  ( 13.25633410266679313, -4.503970704919842305, 4.567388001802134667 ) ) ;
#5272=CARTESIAN_POINT ( 'NONE',  ( 8.731428362939190890, -13.89598863503036164, 27.21428571428572241 ) ) ;
#5274=CARTESIAN_POINT ( 'NONE',  ( 1.441234910513245149, 13.92619789766829008, 14.85310228751642470 ) ) ;
#5280=CARTESIAN_POINT ( 'NONE',  ( -1.567502665446231180, -13.91197093850540334, 39.85714285714286120 ) ) ;
#5281=CARTESIAN_POINT ( 'NONE',  ( -10.24623928997352351, -10.06191849875416899, 2.504040569626438728 ) ) ;
#5284=CARTESIAN_POINT ( 'NONE',  ( -15.88516839912898071, -1.917699372586004980, 7.138816573230711171 ) ) ;
#5289=CARTESIAN_POINT ( 'NONE',  ( 5.420364854932001819, 15.49051278174644430, 25.07142857142858361 ) ) ;
#5296=CARTESIAN_POINT ( 'NONE',  ( 5.164528828830335705, -15.14410076328347543, 19.43261199819785645 ) ) ;
#5297=CARTESIAN_POINT ( 'NONE',  ( 13.89598863503046111, -8.731428362939032795, 38.78571428571429180 ) ) ;
#5300=CARTESIAN_POINT ( 'NONE',  ( -15.91362231745475597, -1.665163862720028254, 15.14689771248357708 ) ) ;
#5301=CARTESIAN_POINT ( 'NONE',  ( -13.91197093850538380, -1.567502665446387278, 29.14285714285714235 ) ) ;
#5302=CARTESIAN_POINT ( 'NONE',  ( 13.89598863503046111, -8.731428362939032795, 8.785714285714293581 ) ) ;
#5303=CARTESIAN_POINT ( 'NONE',  ( 5.284464991282756152, -15.10213328493384743, 45.42857142857143060 ) ) ;
#5307=CARTESIAN_POINT ( 'NONE',  ( -13.54758718765249625, -8.512513224245459753, 46.71428571428571530 ) ) ;
#5309=CARTESIAN_POINT ( 'NONE',  ( 4.619798703721856192, 13.59724543428036725, 9.067388001802141773 ) ) ;
#5311=CARTESIAN_POINT ( 'NONE',  ( 10.13893307789800957, 12.50873118924980609, 47.39553751340654486 ) ) ;
#5313=CARTESIAN_POINT ( 'NONE',  ( -1.607813917173034124, 14.26974319298267346, 30.64285714285714946 ) ) ;
#5315=CARTESIAN_POINT ( 'NONE',  ( -11.92174236212692051, -7.340858601238089420, 26.71832628391215536 ) ) ;
#5318=CARTESIAN_POINT ( 'NONE',  ( 7.750357176954296712, -12.08964793087877787, 41.21024514465928235 ) ) ;
#5321=CARTESIAN_POINT ( 'NONE',  ( -5.297344310588352201, -15.53355953199867301, 24.06738800180213644 ) ) ;
#5325=CARTESIAN_POINT ( 'NONE',  ( 9.809645194533960222, 9.989344678689363377, 51.49595943037355994 ) ) ;
#5329=CARTESIAN_POINT ( 'NONE',  ( 12.08964793087886314, -7.750357176954162597, 24.78975485534072476 ) ) ;
#5332=CARTESIAN_POINT ( 'NONE',  ( 5.297344310588354865, 15.53355953199867301, 51.06738800180214355 ) ) ;
#5336=CARTESIAN_POINT ( 'NONE',  ( 4.743843029824831525, -13.17239914596749095, 11.42453085894499587 ) ) ;
#5340=CARTESIAN_POINT ( 'NONE',  ( -11.22385875690717327, 11.40355824106234550, 46.00404056962644006 ) ) ;
#5341=CARTESIAN_POINT ( 'NONE',  ( -4.623906867372410190, 13.21436662431711895, 42.42857142857143060 ) ) ;
#5343=CARTESIAN_POINT ( 'NONE',  ( 11.92174236212692229, 7.340858601238088532, -0.2816737160878517443 ) ) ;
#5345=CARTESIAN_POINT ( 'NONE',  ( -13.96533075980324234, 8.621071003556515677, 7.781673716087849968 ) ) ;
#5347=CARTESIAN_POINT ( 'NONE',  ( 15.10213328493390783, -5.284464991282587398, 26.57142857142857295 ) ) ;
#5354=CARTESIAN_POINT ( 'NONE',  ( 10.03895970123120307, 12.58845729673829972, 49.39149694378009769 ) ) ;
#5355=CARTESIAN_POINT ( 'NONE',  ( 16.29368510291089223, -1.967016585148476882, 24.36118342676929416 ) ) ;
#5356=CARTESIAN_POINT ( 'NONE',  ( -5.284464991282755264, 15.10213328493384743, 18.42857142857143415 ) ) ;
#5357=CARTESIAN_POINT ( 'NONE',  ( 0.1896486214910092227, 16.00782165069140817, 48.73000000000003951 ) ) ;
#5361=CARTESIAN_POINT ( 'NONE',  ( 1.791431617652837316, 15.89939535829188877, 42.85714285714285410 ) ) ;
#5363=CARTESIAN_POINT ( 'NONE',  ( 13.54758718765249803, 8.512513224245457977, 1.714285714285716855 ) ) ;
#5364=CARTESIAN_POINT ( 'NONE',  ( -13.54758718765249625, -8.512513224245459753, 4.714285714285712636 ) ) ;
#5365=CARTESIAN_POINT ( 'NONE',  ( 12.15899005565164792, -7.639999817571654361, 26.78571428571429180 ) ) ;
#5366=CARTESIAN_POINT ( 'NONE',  ( -1.693770420379220099, -13.89774397934251837, 37.86118342676929416 ) ) ;
#5368=CARTESIAN_POINT ( 'NONE',  ( -12.22833218042443271, 7.529642458189139909, 37.78167371608785174 ) ) ;
#5371=CARTESIAN_POINT ( 'NONE',  ( -11.40355824106246807, 11.22385875690704715, 19.99595943037356349 ) ) ;
#5372=CARTESIAN_POINT ( 'NONE',  ( -1.837501619626327853, 16.30827793483733856, 6.642857142857143238 ) ) ;
#5374=CARTESIAN_POINT ( 'NONE',  ( 13.96533075980324234, -8.621071003556521006, 28.78167371608785174 ) ) ;
#5378=CARTESIAN_POINT ( 'NONE',  ( 8.884063115244108744, 10.93517402715751885, 47.39553751340654486 ) ) ;
#5380=CARTESIAN_POINT ( 'NONE',  ( 13.51115193377584589, 4.865839792409294873, 3.924530858944990541 ) ) ;
#5382=CARTESIAN_POINT ( 'NONE',  ( -4.619798703721853528, -13.59724543428036725, 30.06738800180214355 ) ) ;
#5386=CARTESIAN_POINT ( 'NONE',  ( -4.742819248065502258, -13.55419868402813677, 40.07142857142857650 ) ) ;
#5387=CARTESIAN_POINT ( 'NONE',  ( -13.59724543428031573, -4.619798703722008959, 2.932611998197868886 ) ) ;
#5389=CARTESIAN_POINT ( 'NONE',  ( 15.14410076328353227, -5.164528828830166063, 10.56738800180213644 ) ) ;
#5392=CARTESIAN_POINT ( 'NONE',  ( -11.31370849898482156, 11.31370849898469544, 30.00000000000000355 ) ) ;
#5399=CARTESIAN_POINT ( 'NONE',  ( -1.917699372585823570, -15.88516839912900558, 19.86118342676929416 ) ) ;
#5400=CARTESIAN_POINT ( 'NONE',  ( 16.30827793483735633, -1.837501619626142890, 38.35714285714287541 ) ) ;
#5401=CARTESIAN_POINT ( 'NONE',  ( -15.53355953199861794, -5.297344310588530725, 14.93261199819787066 ) ) ;
#5403=CARTESIAN_POINT ( 'NONE',  ( 13.54758718765249803, 8.512513224245457977, 19.71428571428571175 ) ) ;
#5407=CARTESIAN_POINT ( 'NONE',  ( -11.31370849898482156, 11.31370849898469544, 42.00000000000000000 ) ) ;
#5410=CARTESIAN_POINT ( 'NONE',  ( 8.512513224245308763, 13.54758718765259040, 7.285714285714284699 ) ) ;
#5411=CARTESIAN_POINT ( 'NONE',  ( -15.06016580658428694, 5.404401153735006957, 45.57546914105501656 ) ) ;
#5412=CARTESIAN_POINT ( 'NONE',  ( 10.15407889436379030, 10.15407889436390221, 19.50000000000000355 ) ) ;
#5413=CARTESIAN_POINT ( 'NONE',  ( 13.92619789766827587, 1.441234910513398582, 36.14689771248357886 ) ) ;
#5416=CARTESIAN_POINT ( 'NONE',  ( -1.737328882695368115, 14.25515036105620581, 38.63881657323070584 ) ) ;
#5420=CARTESIAN_POINT ( 'NONE',  ( 16.32287076676382043, -1.707986654103810897, 22.35310228751642114 ) ) ;
#5421=CARTESIAN_POINT ( 'NONE',  ( 16.30827793483735633, -1.837501619626142890, 8.357142857142855874 ) ) ;
#5423=CARTESIAN_POINT ( 'NONE',  ( -1.665163862719845067, -15.91362231745477374, 17.85310228751642114 ) ) ;
#5428=CARTESIAN_POINT ( 'NONE',  ( -4.743843029824828861, 13.17239914596749450, 8.424530858944992318 ) ) ;
#5430=CARTESIAN_POINT ( 'NONE',  ( 16.30827793483735633, -1.837501619626142890, 32.35714285714286120 ) ) ;
#5432=CARTESIAN_POINT ( 'NONE',  ( 13.89774397934249706, 1.693770420379375308, 28.13881657323070939 ) ) ;
#5436=CARTESIAN_POINT ( 'NONE',  ( 11.40355824106234550, 11.22385875690717327, 47.50404056962644006 ) ) ;
#5437=CARTESIAN_POINT ( 'NONE',  ( 1.693770420379222319, 13.89774397934251837, 10.86118342676929238 ) ) ;
#5438=CARTESIAN_POINT ( 'NONE',  ( 13.92619789766827587, 1.441234910513398582, 0.1468977124835755543 ) ) ;
#5441=CARTESIAN_POINT ( 'NONE',  ( 16.32287076676382043, -1.707986654103810897, 4.353102287516421143 ) ) ;
#5444=CARTESIAN_POINT ( 'NONE',  ( 15.49051278174638036, 5.420364854932175014, 37.92857142857143060 ) ) ;
#5451=CARTESIAN_POINT ( 'NONE',  ( 8.621071003556677326, -13.96533075980314287, 19.21832628391215181 ) ) ;
#5455=CARTESIAN_POINT ( 'NONE',  ( -8.512513224245306986, -13.54758718765259218, 16.28571428571428470 ) ) ;
#5457=CARTESIAN_POINT ( 'NONE',  ( -15.49051278174638036, -5.420364854932175902, 4.928571428571430602 ) ) ;
#5459=CARTESIAN_POINT ( 'NONE',  ( 13.89598863503045933, -8.731428362939032795, 44.78571428571429180 ) ) ;
#5464=CARTESIAN_POINT ( 'NONE',  ( -16.30827793483735988, 1.837501619626141780, 5.357142857142856762 ) ) ;
#5465=CARTESIAN_POINT ( 'NONE',  ( 15.10213328493390783, -5.284464991282587398, 2.571428571428571619 ) ) ;
#5466=CARTESIAN_POINT ( 'NONE',  ( 13.21436662431716869, -4.623906867372263640, 38.57142857142857650 ) ) ;
#5468=CARTESIAN_POINT ( 'NONE',  ( -4.865839792409144771, -13.51115193377589740, 32.07546914105502367 ) ) ;
#5473=CARTESIAN_POINT ( 'NONE',  ( 1.737328882695370558, -14.25515036105620581, 35.63881657323071295 ) ) ;
#5475=CARTESIAN_POINT ( 'NONE',  ( -15.14410076328353227, 5.164528828830164287, 25.56738800180213644 ) ) ;
#5476=CARTESIAN_POINT ( 'NONE',  ( 11.31370849898482334, -11.31370849898469366, 9.000000000000001776 ) ) ;
#5477=CARTESIAN_POINT ( 'NONE',  ( 5.297344310588354865, 15.53355953199867301, 21.06738800180213644 ) ) ;
#5483=CARTESIAN_POINT ( 'NONE',  ( 13.89598863503046111, -8.731428362939032795, 32.78571428571430602 ) ) ;
#5486=CARTESIAN_POINT ( 'NONE',  ( 14.28433602490915000, -1.478298951650544479, 4.353102287516421143 ) ) ;
#5488=CARTESIAN_POINT ( 'NONE',  ( -5.284464991282755264, 15.10213328493384743, 12.42857142857142705 ) ) ;
#5493=CARTESIAN_POINT ( 'NONE',  ( 13.17239914596754424, -4.743843029824685864, 6.575469141055007682 ) ) ;
#5495=CARTESIAN_POINT ( 'NONE',  ( -12.08964793087886314, 7.750357176954159932, 15.78975485534072121 ) ) ;
#5496=CARTESIAN_POINT ( 'NONE',  ( 15.44746603149413922, 5.543385399275817527, 9.924530858944988765 ) ) ;
#5498=CARTESIAN_POINT ( 'NONE',  ( 15.49051278174638036, 5.420364854932175014, 43.92857142857143060 ) ) ;
#5505=CARTESIAN_POINT ( 'NONE',  ( -1.707986654103994528, 16.32287076676380266, 22.64689771248357530 ) ) ;
#5507=CARTESIAN_POINT ( 'NONE',  ( -13.61519076058348254, -8.404922754268771001, 38.71832628391214826 ) ) ;
#5508=CARTESIAN_POINT ( 'NONE',  ( -15.89939535829186923, -1.791431617653016062, 17.14285714285713880 ) ) ;
#5510=CARTESIAN_POINT ( 'NONE',  ( 15.89939535829187278, 1.791431617653015174, 8.142857142857145902 ) ) ;
#5515=CARTESIAN_POINT ( 'NONE',  ( -4.865839792409144771, -13.51115193377589740, 44.07546914105503078 ) ) ;
#5516=CARTESIAN_POINT ( 'NONE',  ( -13.54758718765249625, -8.512513224245459753, 10.71428571428571708 ) ) ;
#5517=CARTESIAN_POINT ( 'NONE',  ( -14.26974319298268767, 1.607813917172874696, 35.35714285714286120 ) ) ;
#5518=CARTESIAN_POINT ( 'NONE',  ( -14.25515036105622890, 1.737328882695209575, 39.36118342676930837 ) ) ;
#5522=CARTESIAN_POINT ( 'NONE',  ( 4.619798703721856192, 13.59724543428036725, 51.06738800180214355 ) ) ;
#5524=CARTESIAN_POINT ( 'NONE',  ( -11.51250119794888072, -11.69682198916848037, 30.49595943037356349 ) ) ;
#5525=CARTESIAN_POINT ( 'NONE',  ( -15.89939535829186923, -1.791431617653016062, 17.14285714285713880 ) ) ;
#5526=CARTESIAN_POINT ( 'NONE',  ( 15.14410076328353227, -5.164528828830166063, 22.56738800180214000 ) ) ;
#5530=CARTESIAN_POINT ( 'NONE',  ( 11.31370849898482334, -11.31370849898469366, 33.00000000000000000 ) ) ;
#5532=CARTESIAN_POINT ( 'NONE',  ( -1.441234910513241818, -13.92619789766829008, 17.85310228751642114 ) ) ;
#5536=CARTESIAN_POINT ( 'NONE',  ( -13.25633410266679313, 4.503970704919840529, 25.56738800180213644 ) ) ;
#5540=CARTESIAN_POINT ( 'NONE',  ( -12.08964793087886314, 7.750357176954159932, 3.789754855340718542 ) ) ;
#5541=CARTESIAN_POINT ( 'NONE',  ( -4.503970704919988854, 13.25633410266674517, 16.43261199819786356 ) ) ;
#5543=CARTESIAN_POINT ( 'NONE',  ( 11.40355824106246985, -11.22385875690704538, 16.99595943037355994 ) ) ;
#5545=CARTESIAN_POINT ( 'NONE',  ( 1.791431617652837316, 15.89939535829188877, 48.85714285714286120 ) ) ;
#5551=CARTESIAN_POINT ( 'NONE',  ( -15.53355953199861794, -5.297344310588530725, 26.93261199819786356 ) ) ;
#5553=CARTESIAN_POINT ( 'NONE',  ( -1.917699372585823570, -15.88516839912900558, 37.86118342676929416 ) ) ;
#5555=CARTESIAN_POINT ( 'NONE',  ( 15.89939535829187278, 1.791431617653015174, 14.14285714285714413 ) ) ;
#5557=CARTESIAN_POINT ( 'NONE',  ( -11.31370849898482156, 11.31370849898469544, 5.999999999999998224 ) ) ;
#5558=FILL_AREA_STYLE ('',( #7112 ) ) ;
#5561=CARTESIAN_POINT ( 'NONE',  ( 1.707986654103998303, -16.32287076676380266, 1.646897712483578857 ) ) ;
#5562=CARTESIAN_POINT ( 'NONE',  ( 5.284464991282756152, -15.10213328493384743, 9.428571428571425272 ) ) ;
#5563=CARTESIAN_POINT ( 'NONE',  ( -10.15407889436378852, -10.15407889436390398, 40.50000000000000000 ) ) ;
#5564=CARTESIAN_POINT ( 'NONE',  ( 14.25515036105622535, -1.737328882695210241, 36.36118342676930126 ) ) ;
#5566=CARTESIAN_POINT ( 'NONE',  ( 13.92619789766827587, 1.441234910513398582, 30.14689771248358241 ) ) ;
#5569=CARTESIAN_POINT ( 'NONE',  ( -1.607813917173034124, 14.26974319298267524, 0.6428571428571432378 ) ) ;
#5571=CARTESIAN_POINT ( 'NONE',  ( -1.837501619626327853, 16.30827793483733856, 18.64285714285715301 ) ) ;
#5572=CARTESIAN_POINT ( 'NONE',  ( -15.14410076328353227, 5.164528828830164287, 25.56738800180213644 ) ) ;
#5575=CARTESIAN_POINT ( 'NONE',  ( -7.639999817571786700, 12.15899005565156266, 0.2142857142857168273 ) ) ;
#5578=CARTESIAN_POINT ( 'NONE',  ( 4.619798703721856192, 13.59724543428036725, 15.06738800180213822 ) ) ;
#5580=CARTESIAN_POINT ( 'NONE',  ( 5.284464991282756152, -15.10213328493384743, 9.428571428571425272 ) ) ;
#5585=CARTESIAN_POINT ( 'NONE',  ( 12.08964793087886314, -7.750357176954162597, 12.78975485534072121 ) ) ;
#5588=CARTESIAN_POINT ( 'NONE',  ( 10.24623928997352884, 10.06191849875416899, 11.50404056962644006 ) ) ;
#5591=CARTESIAN_POINT ( 'NONE',  ( -13.89598863503046111, 8.731428362939027465, 41.78571428571430602 ) ) ;
#5597=CARTESIAN_POINT ( 'NONE',  ( 13.61519076058348254, 8.404922754268771001, 23.71832628391215181 ) ) ;
#5599=CARTESIAN_POINT ( 'NONE',  ( -8.621071003556675549, 13.96533075980314642, 40.21832628391215536 ) ) ;
#5602=CARTESIAN_POINT ( 'NONE',  ( -1.837501619626328297, 16.30827793483733856, 24.64285714285714235 ) ) ;
#5603=CARTESIAN_POINT ( 'NONE',  ( 3.890496870457673229, 14.43432932945637504, -1.604941620322696453E-32 ) ) ;
#5605=CARTESIAN_POINT ( 'NONE',  ( 15.10213328493390783, -5.284464991282587398, 8.571428571428569398 ) ) ;
#5610=CARTESIAN_POINT ( 'NONE',  ( -8.620103694221995738, -13.47998361472161299, 2.289754855340722539 ) ) ;
#5612=CARTESIAN_POINT ( 'NONE',  ( 15.10213328493390783, -5.284464991282587398, 20.57142857142857295 ) ) ;
#5614=CARTESIAN_POINT ( 'NONE',  ( -1.607813917173034124, 14.26974319298267346, 36.64285714285714590 ) ) ;
#5615=CARTESIAN_POINT ( 'NONE',  ( 1.478298951650704351, -14.28433602490913579, 37.64689771248358596 ) ) ;
#5616=CARTESIAN_POINT ( 'NONE',  ( 13.91197093850538380, 1.567502665446386390, 8.142857142857145902 ) ) ;
#5620=CARTESIAN_POINT ( 'NONE',  ( -7.639999817571787588, 12.15899005565156266, 6.214285714285717965 ) ) ;
#5625=CARTESIAN_POINT ( 'NONE',  ( 15.89939535829187278, 1.791431617653015174, 20.14285714285714235 ) ) ;
#5626=CARTESIAN_POINT ( 'NONE',  ( -11.40355824106246807, 11.22385875690704715, 43.99595943037355994 ) ) ;
#5631=VECTOR ( 'NONE', #4774, 1000.000000000000114 ) ;
#5633=CARTESIAN_POINT ( 'NONE',  ( -12.22833218042443271, 7.529642458189139909, 19.78167371608784819 ) ) ;
#5635=CARTESIAN_POINT ( 'NONE',  ( -8.512513224245306986, -13.54758718765259218, 16.28571428571428470 ) ) ;
#5637=CARTESIAN_POINT ( 'NONE',  ( -1.737328882695368115, 14.25515036105620581, 44.63881657323071295 ) ) ;
#5641=CARTESIAN_POINT ( 'NONE',  ( 13.92619789766827587, 1.441234910513398582, 0.1468977124835755543 ) ) ;
#5643=CARTESIAN_POINT ( 'NONE',  ( 1.693770420379222319, 13.89774397934251837, 10.86118342676929238 ) ) ;
#5646=CARTESIAN_POINT ( 'NONE',  ( -11.40355824106246807, 11.22385875690704715, 1.995959430373561272 ) ) ;
#5652=CARTESIAN_POINT ( 'NONE',  ( -8.620103694221995738, -13.47998361472161299, 26.28975485534072831 ) ) ;
#5654=CARTESIAN_POINT ( 'NONE',  ( 13.61519076058348254, 8.404922754268771001, 35.71832628391214115 ) ) ;
#5657=CARTESIAN_POINT ( 'NONE',  ( 5.284464991282756152, -15.10213328493384743, 27.42857142857143060 ) ) ;
#5658=CARTESIAN_POINT ( 'NONE',  ( 3.773891550226160518, 14.38788920816386785, -1.793508096673563358E-16 ) ) ;
#5660=CARTESIAN_POINT ( 'NONE',  ( 1.791431617652837316, 15.89939535829188877, 0.8571428571428549859 ) ) ;
#5664=CARTESIAN_POINT ( 'NONE',  ( 9.809645194534072132, -9.989344678689256796, 43.00404056962644717 ) ) ;
#5665=CARTESIAN_POINT ( 'NONE',  ( 13.54758718765249803, 8.512513224245457977, 13.71428571428571352 ) ) ;
#5666=CARTESIAN_POINT ( 'NONE',  ( 14.26974319298268767, -1.607813917172876472, 38.35714285714286831 ) ) ;
#5667=CARTESIAN_POINT ( 'NONE',  ( 1.917699372585825790, 15.88516839912900203, -1.138816573230706286 ) ) ;
#5668=CARTESIAN_POINT ( 'NONE',  ( 11.85413878919593422, 7.448449071214774619, 13.71428571428571352 ) ) ;
#5672=CARTESIAN_POINT ( 'NONE',  ( 1.567502665446232957, 13.91197093850540156, 0.8571428571428549859 ) ) ;
#5676=CARTESIAN_POINT ( 'NONE',  ( -8.731428362939187338, 13.89598863503036164, 24.21428571428571530 ) ) ;
#5677=CARTESIAN_POINT ( 'NONE',  ( 5.297344310588354865, 15.53355953199867301, 39.06738800180213644 ) ) ;
#5680=CARTESIAN_POINT ( 'NONE',  ( 14.26974319298268767, -1.607813917172876472, 2.357142857142856762 ) ) ;
#5684=CARTESIAN_POINT ( 'NONE',  ( -1.441234910513241818, -13.92619789766829008, 35.85310228751641404 ) ) ;
#5688=CARTESIAN_POINT ( 'NONE',  ( 10.24623928997352884, 10.06191849875416899, 17.50404056962643651 ) ) ;
#5690=CARTESIAN_POINT ( 'NONE',  ( 1.478298951650704351, -14.28433602490913579, 13.64689771248357708 ) ) ;
#5693=CARTESIAN_POINT ( 'NONE',  ( 5.297344310588354865, 15.53355953199867301, 15.06738800180213822 ) ) ;
#5699=CARTESIAN_POINT ( 'NONE',  ( 1.707986654103998303, -16.32287076676380266, 25.64689771248357886 ) ) ;
#5700=CARTESIAN_POINT ( 'NONE',  ( 4.742819248065503146, 13.55419868402813677, 31.07142857142857295 ) ) ;
#5701=CARTESIAN_POINT ( 'NONE',  ( 15.53355953199861794, 5.297344310588528060, 35.93261199819787066 ) ) ;
#5703=CARTESIAN_POINT ( 'NONE',  ( -15.49051278174638036, -5.420364854932175902, 28.92857142857143771 ) ) ;
#5705=CARTESIAN_POINT ( 'NONE',  ( -16.30827793483735988, 1.837501619626141780, 17.35714285714286476 ) ) ;
#5708=CARTESIAN_POINT ( 'NONE',  ( 7.556039541191335474, 11.78653521626503320, 47.28975485534072476 ) ) ;
#5709=CARTESIAN_POINT ( 'NONE',  ( -13.89598863503046111, 8.731428362939027465, 17.78571428571428115 ) ) ;
#5711=CARTESIAN_POINT ( 'NONE',  ( -13.17239914596754424, 4.743843029824683200, 39.57546914105500946 ) ) ;
#5712=CARTESIAN_POINT ( 'NONE',  ( 4.623906867372411078, -13.21436662431711717, 9.428571428571425272 ) ) ;
#5717=CARTESIAN_POINT ( 'NONE',  ( -9.899494936611716867, 9.899494936611610285, 11.99999999999999645 ) ) ;
#5721=CARTESIAN_POINT ( 'NONE',  ( -15.10213328493390961, 5.284464991282586510, 17.57142857142856940 ) ) ;
#5722=CARTESIAN_POINT ( 'NONE',  ( 15.88516839912898071, 1.917699372586004092, 40.13881657323070584 ) ) ;
#5726=CARTESIAN_POINT ( 'NONE',  ( 9.899494936611718643, -9.899494936611608509, 15.00000000000000000 ) ) ;
#5729=CARTESIAN_POINT ( 'NONE',  ( -14.28433602490915000, 1.478298951650542481, 13.35310228751641937 ) ) ;
#5732=CARTESIAN_POINT ( 'NONE',  ( 13.51115193377584589, 4.865839792409294873, 33.92453085894499054 ) ) ;
#5737=PLANE ( 'NONE',  #7538 ) ;
#5738=CARTESIAN_POINT ( 'NONE',  ( -15.14410076328353227, 5.164528828830164287, 7.567388001802139108 ) ) ;
#5739=CARTESIAN_POINT ( 'NONE',  ( -13.47998361472151174, -8.620103694222146729, 24.71024514465928235 ) ) ;
#5745=CARTESIAN_POINT ( 'NONE',  ( 1.607813917173038121, -14.26974319298267346, 33.64285714285715301 ) ) ;
#5746=CARTESIAN_POINT ( 'NONE',  ( 13.82664651025767100, -8.841785722321541030, 42.78975485534072476 ) ) ;
#5750=CARTESIAN_POINT ( 'NONE',  ( -1.837501619626328297, 16.30827793483733856, 30.64285714285715301 ) ) ;
#5751=CARTESIAN_POINT ( 'NONE',  ( 2.266096533192709206, 14.38188575653963319, -1.488941479308426028E-16 ) ) ;
#5752=CARTESIAN_POINT ( 'NONE',  ( -1.837501619626328297, 16.30827793483733856, 12.64285714285714235 ) ) ;
#5757=CARTESIAN_POINT ( 'NONE',  ( -11.69682198916834892, -11.51250119794901394, 14.50404056962643651 ) ) ;
#5758=CARTESIAN_POINT ( 'NONE',  ( -5.420364854931999155, -15.49051278174644253, 34.07142857142859071 ) ) ;
#5760=CARTESIAN_POINT ( 'NONE',  ( 15.06016580658428694, -5.404401153735007846, 0.5754691410550027975 ) ) ;
#5761=CARTESIAN_POINT ( 'NONE',  ( 9.899494936611718643, -9.899494936611608509, 15.00000000000000000 ) ) ;
#5765=CARTESIAN_POINT ( 'NONE',  ( -13.91197093850538380, -1.567502665446387278, 23.14285714285714590 ) ) ;
#5767=CARTESIAN_POINT ( 'NONE',  ( -8.512513224245306986, -13.54758718765259218, 28.28571428571428825 ) ) ;
#5769=CARTESIAN_POINT ( 'NONE',  ( -16.32287076676382398, 1.707986654103809343, 31.35310228751642470 ) ) ;
#5773=CARTESIAN_POINT ( 'NONE',  ( -14.26974319298268767, 1.607813917172874696, 11.35714285714285765 ) ) ;
#5777=CARTESIAN_POINT ( 'NONE',  ( 1.441234910513245149, 13.92619789766829008, 32.85310228751642114 ) ) ;
#5780=CARTESIAN_POINT ( 'NONE',  ( -7.750357176954294935, 12.08964793087877787, 44.21024514465928235 ) ) ;
#5786=CARTESIAN_POINT ( 'NONE',  ( 13.59724543428031573, 4.619798703722006294, 17.93261199819786711 ) ) ;
#5789=CARTESIAN_POINT ( 'NONE',  ( -11.51250119794888072, -11.69682198916848037, 42.49595943037355994 ) ) ;
#5793=CARTESIAN_POINT ( 'NONE',  ( 13.47998361472151529, 8.620103694222146729, 9.710245144659278793 ) ) ;
#5800=CARTESIAN_POINT ( 'NONE',  ( -1.607813917173034124, 14.26974319298267524, 30.64285714285715301 ) ) ;
#5802=CARTESIAN_POINT ( 'NONE',  ( -8.512513224245306986, -13.54758718765259218, 46.28571428571429180 ) ) ;
#5803=CARTESIAN_POINT ( 'NONE',  ( 3.607533428936334552, 14.36432425738846419, -9.697396257098264345E-17 ) ) ;
#5804=CARTESIAN_POINT ( 'NONE',  ( -8.731428362939189114, 13.89598863503036341, 18.21428571428571885 ) ) ;
#5809=CARTESIAN_POINT ( 'NONE',  ( 16.29368510291089223, -1.967016585148476882, 12.36118342676929771 ) ) ;
#5810=CARTESIAN_POINT ( 'NONE',  ( -16.30827793483735988, 1.837501619626141780, 23.35714285714286476 ) ) ;
#5811=CARTESIAN_POINT ( 'NONE',  ( 5.164528828830335705, -15.14410076328347543, 7.432611998197861780 ) ) ;
#5813=CARTESIAN_POINT ( 'NONE',  ( -10.15407889436378852, -10.15407889436390576, 16.50000000000000000 ) ) ;
#5818=CARTESIAN_POINT ( 'NONE',  ( 4.623906867372411078, -13.21436662431711717, 15.42857142857143060 ) ) ;
#5820=CARTESIAN_POINT ( 'NONE',  ( 5.284464991282756152, -15.10213328493384743, 33.42857142857143060 ) ) ;
#5821=CARTESIAN_POINT ( 'NONE',  ( 11.40355824106246985, -11.22385875690704538, 40.99595943037355994 ) ) ;
#5824=CARTESIAN_POINT ( 'NONE',  ( 11.85413878919593422, 7.448449071214774619, 7.714285714285715301 ) ) ;
#5825=CARTESIAN_POINT ( 'NONE',  ( -7.750357176954294935, 12.08964793087877787, 32.21024514465928235 ) ) ;
#5827=CARTESIAN_POINT ( 'NONE',  ( 1.595235446793586753, 13.94740710718646248, 48.73000000000003951 ) ) ;
#5828=CARTESIAN_POINT ( 'NONE',  ( -4.743843029824828861, 13.17239914596749450, 38.42453085894499054 ) ) ;
#5834=CARTESIAN_POINT ( 'NONE',  ( -13.17239914596754424, 4.743843029824683200, 27.57546914105500946 ) ) ;
#5836=CARTESIAN_POINT ( 'NONE',  ( 13.47998361472151529, 8.620103694222146729, 33.71024514465927524 ) ) ;
#5838=CARTESIAN_POINT ( 'NONE',  ( -15.10213328493390961, 5.284464991282586510, 17.57142857142856940 ) ) ;
#5839=CARTESIAN_POINT ( 'NONE',  ( -8.404922754268618235, -13.61519076058357491, 6.281673716087846415 ) ) ;
#5844=CARTESIAN_POINT ( 'NONE',  ( 13.61519076058348254, 8.404922754268771001, 35.71832628391214115 ) ) ;
#5845=CARTESIAN_POINT ( 'NONE',  ( -10.15407889436378852, -10.15407889436390576, 34.50000000000000000 ) ) ;
#5846=CARTESIAN_POINT ( 'NONE',  ( -10.15407889436378852, -10.15407889436390576, 34.50000000000000000 ) ) ;
#5848=CARTESIAN_POINT ( 'NONE',  ( 16.30827793483735633, -1.837501619626142890, 38.35714285714287541 ) ) ;
#5850=CARTESIAN_POINT ( 'NONE',  ( -11.31370849898482156, 11.31370849898469544, 18.00000000000000355 ) ) ;
#5855=CARTESIAN_POINT ( 'NONE',  ( -1.917699372585823570, -15.88516839912900558, 13.86118342676929416 ) ) ;
#5856=CARTESIAN_POINT ( 'NONE',  ( 15.10213328493390783, -5.284464991282587398, 26.57142857142857295 ) ) ;
#5858=CARTESIAN_POINT ( 'NONE',  ( -8.621071003556675549, 13.96533075980314642, 4.218326283912150032 ) ) ;
#5859=CARTESIAN_POINT ( 'NONE',  ( -11.85413878919593422, -7.448449071214776396, 22.71428571428571530 ) ) ;
#5860=CARTESIAN_POINT ( 'NONE',  ( -11.60466159355861926, -11.60466159355875249, 10.50000000000000533 ) ) ;
#5863=CARTESIAN_POINT ( 'NONE',  ( 4.742819248065503146, 13.55419868402813677, 19.07142857142856940 ) ) ;
#5865=CARTESIAN_POINT ( 'NONE',  ( 13.89598863503045933, -8.731428362939032795, 32.78571428571429180 ) ) ;
#5866=CARTESIAN_POINT ( 'NONE',  ( -13.89774397934249706, -1.693770420379375974, 7.138816573230711171 ) ) ;
#5869=CARTESIAN_POINT ( 'NONE',  ( -13.91197093850538380, -1.567502665446387278, 17.14285714285713880 ) ) ;
#5872=CARTESIAN_POINT ( 'NONE',  ( -11.78653521626494793, -7.556039541191465148, 30.71024514465928235 ) ) ;
#5875=CARTESIAN_POINT ( 'NONE',  ( 3.470966000225593096, 13.60552200844329285, 48.73000000000002530 ) ) ;
#5877=CARTESIAN_POINT ( 'NONE',  ( 11.85413878919593422, 7.448449071214774619, 1.714285714285716855 ) ) ;
#5882=CARTESIAN_POINT ( 'NONE',  ( -7.529642458189277576, 12.22833218042435455, 16.21832628391214470 ) ) ;
#5884=CARTESIAN_POINT ( 'NONE',  ( 11.40355824106246985, -11.22385875690704538, 34.99595943037355994 ) ) ;
#5885=CARTESIAN_POINT ( 'NONE',  ( -12.50678508136871869, 7.704882173211043295, 48.73000000000002530 ) ) ;
#5886=CARTESIAN_POINT ( 'NONE',  ( -16.30827793483735988, 1.837501619626141780, 23.35714285714286476 ) ) ;
#5888=CARTESIAN_POINT ( 'NONE',  ( 14.28433602490915000, -1.478298951650544479, 10.35310228751642292 ) ) ;
#5892=CARTESIAN_POINT ( 'NONE',  ( -4.742819248065502258, -13.55419868402813677, 28.07142857142857295 ) ) ;
#5894=CARTESIAN_POINT ( 'NONE',  ( 10.15407889436379030, 10.15407889436390576, 43.50000000000000711 ) ) ;
#5897=CARTESIAN_POINT ( 'NONE',  ( -1.837501619626328297, 16.30827793483733856, 48.64285714285716011 ) ) ;
#5899=CARTESIAN_POINT ( 'NONE',  ( 5.420364854932001819, 15.49051278174644430, 13.07142857142857295 ) ) ;
#5906=CARTESIAN_POINT ( 'NONE',  ( -5.164528828830334817, 15.14410076328347543, 10.43261199819786356 ) ) ;
#5907=CARTESIAN_POINT ( 'NONE',  ( -5.284464991282755264, 15.10213328493384743, 24.42857142857143060 ) ) ;
#5909=CARTESIAN_POINT ( 'NONE',  ( -13.55419868402807992, -4.742819248065651472, 46.92857142857143060 ) ) ;
#5910=CARTESIAN_POINT ( 'NONE',  ( 15.53355953199861794, 5.297344310588528060, 11.93261199819786178 ) ) ;
#5912=CARTESIAN_POINT ( 'NONE',  ( -9.899494936611716867, 9.899494936611610285, 18.00000000000000355 ) ) ;
#5913=CARTESIAN_POINT ( 'NONE',  ( 15.49051278174638036, 5.420364854932175014, 1.928571428571430380 ) ) ;
#5916=CARTESIAN_POINT ( 'NONE',  ( -4.742819248065502258, -13.55419868402813677, 16.07142857142857650 ) ) ;
#5917=CARTESIAN_POINT ( 'NONE',  ( 15.49051278174637858, 5.420364854932174126, 31.92857142857143060 ) ) ;
#5918=CARTESIAN_POINT ( 'NONE',  ( -5.297344310588352201, -15.53355953199867301, 48.06738800180213644 ) ) ;
#5921=CARTESIAN_POINT ( 'NONE',  ( 13.91197093850538380, 1.567502665446386390, 8.142857142857145902 ) ) ;
#5923=CARTESIAN_POINT ( 'NONE',  ( -1.441234910513241818, -13.92619789766829008, 29.85310228751642470 ) ) ;
#5927=CARTESIAN_POINT ( 'NONE',  ( -0.3021515714675195863, 13.99673906407701729, 48.73000000000003951 ) ) ;
#5929=CARTESIAN_POINT ( 'NONE',  ( -13.51115193377584589, -4.865839792409295761, 48.92453085894499054 ) ) ;
#5933=CARTESIAN_POINT ( 'NONE',  ( 4.503970704919991519, -13.25633410266674517, 31.43261199819787421 ) ) ;
#5936=CARTESIAN_POINT ( 'NONE',  ( -1.967016585148659846, 16.29368510291087091, 44.63881657323071295 ) ) ;
#5937=CARTESIAN_POINT ( 'NONE',  ( -12.62058114252586805, 7.581620562087779014, 48.73000000000001108 ) ) ;
#5938=CARTESIAN_POINT ( 'NONE',  ( -8.731428362939189114, 13.89598863503036341, 18.21428571428571885 ) ) ;
#5942=CARTESIAN_POINT ( 'NONE',  ( -4.619798703721853528, -13.59724543428036725, 12.06738800180214000 ) ) ;
#5946=CARTESIAN_POINT ( 'NONE',  ( -15.06016580658428694, 5.404401153735006957, 33.57546914105500946 ) ) ;
#5947=CARTESIAN_POINT ( 'NONE',  ( -1.607813917173034124, 14.26974319298267524, 48.64285714285716011 ) ) ;
#5949=CARTESIAN_POINT ( 'NONE',  ( 12.15899005565164792, -7.639999817571655250, 38.78571428571429180 ) ) ;
#5951=CARTESIAN_POINT ( 'NONE',  ( -11.31370849898482156, 11.31370849898469544, 42.00000000000000000 ) ) ;
#5953=CARTESIAN_POINT ( 'NONE',  ( -8.731428362939189114, 13.89598863503036341, 24.21428571428571530 ) ) ;
#5958=UNCERTAINTY_MEASURE_WITH_UNIT (LENGTH_MEASURE( 1.000000000000000082E-05 ), #1611, 'distance_accuracy_value', 'NONE');
#5960=CARTESIAN_POINT ( 'NONE',  ( 15.53355953199861794, 5.297344310588528060, 11.93261199819786178 ) ) ;
#5961=CARTESIAN_POINT ( 'NONE',  ( 11.60466159355862104, 11.60466159355875071, 31.50000000000001421 ) ) ;
#5963=CARTESIAN_POINT ( 'NONE',  ( 15.06016580658428694, -5.404401153735007846, 6.575469141055007682 ) ) ;
#5964=CARTESIAN_POINT ( 'NONE',  ( 13.21436662431716869, -4.623906867372263640, 20.57142857142857295 ) ) ;
#5965=CARTESIAN_POINT ( 'NONE',  ( -1.837501619626328297, 16.30827793483733856, 6.642857142857143238 ) ) ;
#5966=CARTESIAN_POINT ( 'NONE',  ( 15.49051278174638036, 5.420364854932175014, 43.92857142857143060 ) ) ;
#5970=CARTESIAN_POINT ( 'NONE',  ( 13.89598863503045933, -8.731428362939032795, 26.78571428571429180 ) ) ;
#5971=CARTESIAN_POINT ( 'NONE',  ( 5.297344310588354865, 15.53355953199867301, 51.06738800180214355 ) ) ;
#5974=CARTESIAN_POINT ( 'NONE',  ( 1.567502665446232957, 13.91197093850540156, 30.85714285714286120 ) ) ;
#5976=CARTESIAN_POINT ( 'NONE',  ( -7.340858601237953529, -11.92174236212700222, 30.28167371608785530 ) ) ;
#5981=CARTESIAN_POINT ( 'NONE',  ( -1.567502665446231180, -13.91197093850540334, 3.857142857142857650 ) ) ;
#5985=CARTESIAN_POINT ( 'NONE',  ( 10.24623928997352884, 10.06191849875416899, 29.50404056962643295 ) ) ;
#5987=CARTESIAN_POINT ( 'NONE',  ( -15.44746603149413922, -5.543385399275820191, 36.92453085894499765 ) ) ;
#5989=CARTESIAN_POINT ( 'NONE',  ( -12.79983919530466707, 7.405287656185944201, 48.73000000000000398 ) ) ;
#5990=CARTESIAN_POINT ( 'NONE',  ( -16.30827793483735988, 1.837501619626141780, 29.35714285714285765 ) ) ;
#5993=CARTESIAN_POINT ( 'NONE',  ( -11.78653521626494793, -7.556039541191465148, 12.71024514465927879 ) ) ;
#5997=CARTESIAN_POINT ( 'NONE',  ( 11.85413878919593422, 7.448449071214774619, 43.71428571428572241 ) ) ;
#5998=CARTESIAN_POINT ( 'NONE',  ( -12.15899005565164792, 7.639999817571651697, 41.78571428571430602 ) ) ;
#6000=CARTESIAN_POINT ( 'NONE',  ( 8.731428362939190890, -13.89598863503036164, 39.21428571428571530 ) ) ;
#6002=CARTESIAN_POINT ( 'NONE',  ( 15.89939535829187278, 1.791431617653015174, 32.14285714285714590 ) ) ;
#6010=CARTESIAN_POINT ( 'NONE',  ( 5.284464991282756152, -15.10213328493384743, 39.42857142857143060 ) ) ;
#6011=CARTESIAN_POINT ( 'NONE',  ( 13.61519076058348254, 8.404922754268771001, 23.71832628391215181 ) ) ;
#6012=CARTESIAN_POINT ( 'NONE',  ( -1.567502665446231180, -13.91197093850540334, 27.85714285714285765 ) ) ;
#6013=CARTESIAN_POINT ( 'NONE',  ( -1.837501619626328297, 16.30827793483733856, 0.6428571428571432378 ) ) ;
#6014=CARTESIAN_POINT ( 'NONE',  ( -1.837501619626328297, 16.30827793483733856, 42.64285714285715301 ) ) ;
#6018=CARTESIAN_POINT ( 'NONE',  ( -8.512513224245306986, -13.54758718765259218, 40.28571428571428470 ) ) ;
#6019=CARTESIAN_POINT ( 'NONE',  ( 7.750357176954296712, -12.08964793087877787, 5.210245144659280569 ) ) ;
#6021=CARTESIAN_POINT ( 'NONE',  ( -5.284464991282755264, 15.10213328493384743, 6.428571428571429713 ) ) ;
#6022=CARTESIAN_POINT ( 'NONE',  ( 9.899494936611718643, -9.899494936611608509, 27.00000000000000355 ) ) ;
#6024=CARTESIAN_POINT ( 'NONE',  ( 10.06191849875406064, 10.24623928997363187, 39.49595943037357415 ) ) ;
#6027=CARTESIAN_POINT ( 'NONE',  ( 15.44746603149413922, 5.543385399275817527, 27.92453085894499054 ) ) ;
#6033=CARTESIAN_POINT ( 'NONE',  ( -12.08964793087886314, 7.750357176954159932, 33.78975485534073897 ) ) ;
#6038=CARTESIAN_POINT ( 'NONE',  ( -16.32287076676382398, 1.707986654103809343, 49.35310228751642114 ) ) ;
#6039=CARTESIAN_POINT ( 'NONE',  ( -12.86610055725239654, 8.450849116819570739, 48.72999999999998977 ) ) ;
#6041=CARTESIAN_POINT ( 'NONE',  ( 12.22833218042443271, -7.529642458189144349, 22.78167371608784464 ) ) ;
#6046=CARTESIAN_POINT ( 'NONE',  ( 16.29368510291089223, -1.967016585148476882, 42.36118342676930126 ) ) ;
#6047=CARTESIAN_POINT ( 'NONE',  ( 11.85413878919593422, 7.448449071214774619, 37.71428571428571530 ) ) ;
#6048=CARTESIAN_POINT ( 'NONE',  ( 11.92174236212692229, 7.340858601238088532, 5.718326283912152697 ) ) ;
#6050=CARTESIAN_POINT ( 'NONE',  ( 1.872357960115197173, 15.39586052177234521, -2.187087473825155240E-16 ) ) ;
#6051=CARTESIAN_POINT ( 'NONE',  ( 16.30827793483735633, -1.837501619626142890, 32.35714285714286120 ) ) ;
#6059=CARTESIAN_POINT ( 'NONE',  ( 1.791431617652837316, 15.89939535829188877, 48.85714285714286120 ) ) ;
#6062=CARTESIAN_POINT ( 'NONE',  ( -5.543385399275643444, -15.44746603149420494, 14.07546914105500768 ) ) ;
#6063=CARTESIAN_POINT ( 'NONE',  ( -7.448449071214644945, -11.85413878919601771, 28.28571428571428825 ) ) ;
#6064=CARTESIAN_POINT ( 'NONE',  ( -15.10213328493390961, 5.284464991282586510, 5.571428571428574728 ) ) ;
#6065=CARTESIAN_POINT ( 'NONE',  ( -11.31370849898482156, 11.31370849898469544, 42.00000000000000000 ) ) ;
#6069=CARTESIAN_POINT ( 'NONE',  ( -1.791431617652833763, -15.89939535829188877, 39.85714285714286120 ) ) ;
#6070=CARTESIAN_POINT ( 'NONE',  ( -4.743843029824828861, 13.17239914596749450, 8.424530858944992318 ) ) ;
#6072=CARTESIAN_POINT ( 'NONE',  ( 11.31370849898482334, -11.31370849898469366, 3.000000000000002665 ) ) ;
#6073=CARTESIAN_POINT ( 'NONE',  ( 11.40355824106234550, 11.22385875690717327, 47.50404056962644006 ) ) ;
#6074=CARTESIAN_POINT ( 'NONE',  ( 4.742819248065502258, 13.55419868402813499, 19.07142857142856940 ) ) ;
#6075=CARTESIAN_POINT ( 'NONE',  ( -4.503970704919988854, 13.25633410266674517, 22.43261199819786356 ) ) ;
#6076=CARTESIAN_POINT ( 'NONE',  ( 4.743843029824831525, -13.17239914596749095, 41.42453085894499765 ) ) ;
#6079=CARTESIAN_POINT ( 'NONE',  ( -1.665163862719845067, -15.91362231745477374, 29.85310228751642470 ) ) ;
#6080=CARTESIAN_POINT ( 'NONE',  ( -1.837501619626327853, 16.30827793483733856, 0.6428571428571433488 ) ) ;
#6083=CARTESIAN_POINT ( 'NONE',  ( 7.750357176954296712, -12.08964793087877787, 47.21024514465928235 ) ) ;
#6087=CARTESIAN_POINT ( 'NONE',  ( 4.503970704919991519, -13.25633410266674517, 25.43261199819786711 ) ) ;
#6091=CARTESIAN_POINT ( 'NONE',  ( -5.297344310588352201, -15.53355953199867301, 48.06738800180213644 ) ) ;
#6094=CARTESIAN_POINT ( 'NONE',  ( -13.89774397934249706, -1.693770420379375974, 13.13881657323070584 ) ) ;
#6100=CARTESIAN_POINT ( 'NONE',  ( -11.69682198916834892, -11.51250119794901394, 44.50404056962644006 ) ) ;
#6101=CARTESIAN_POINT ( 'NONE',  ( -7.639999817571787588, 12.15899005565156266, 42.21428571428572241 ) ) ;
#6102=CARTESIAN_POINT ( 'NONE',  ( -11.92174236212692051, -7.340858601238089420, 2.718326283912150476 ) ) ;
#6105=CARTESIAN_POINT ( 'NONE',  ( -13.47998361472151174, -8.620103694222146729, 6.710245144659284122 ) ) ;
#6109=CARTESIAN_POINT ( 'NONE',  ( 5.284464991282756152, -15.10213328493384743, 27.42857142857143060 ) ) ;
#6115=CARTESIAN_POINT ( 'NONE',  ( -8.621071003556675549, 13.96533075980314642, 22.21832628391215181 ) ) ;
#6116=CARTESIAN_POINT ( 'NONE',  ( 8.512513224245308763, 13.54758718765259040, 49.28571428571428470 ) ) ;
#6119=CARTESIAN_POINT ( 'NONE',  ( -13.61519076058348254, -8.404922754268771001, 14.71832628391215003 ) ) ;
#6121=CARTESIAN_POINT ( 'NONE',  ( -11.31370849898482156, 11.31370849898469544, 18.00000000000000355 ) ) ;
#6122=CARTESIAN_POINT ( 'NONE',  ( 10.35987736339271770, 11.82290011998975388, 48.73000000000001819 ) ) ;
#6126=CARTESIAN_POINT ( 'NONE',  ( -1.837501619626327853, 16.30827793483733856, 42.64285714285714590 ) ) ;
#6129=CARTESIAN_POINT ( 'NONE',  ( -15.49051278174638036, -5.420364854932175902, 4.928571428571430602 ) ) ;
#6130=CARTESIAN_POINT ( 'NONE',  ( 14.26974319298268767, -1.607813917172876472, 26.35714285714286120 ) ) ;
#6133=CARTESIAN_POINT ( 'NONE',  ( -10.06191849875405531, -10.24623928997363542, 36.49595943037355994 ) ) ;
#6136=CARTESIAN_POINT ( 'NONE',  ( -11.40355824106246807, 11.22385875690704715, 25.99595943037356349 ) ) ;
#6137=CARTESIAN_POINT ( 'NONE',  ( -11.60466159355861748, -11.60466159355874893, 4.500000000000003553 ) ) ;
#6139=CARTESIAN_POINT ( 'NONE',  ( -8.841785722321695573, 13.82664651025757152, 20.21024514465928235 ) ) ;
#6143=CARTESIAN_POINT ( 'NONE',  ( 1.693770420379222319, 13.89774397934251837, 28.86118342676929416 ) ) ;
#6145=CARTESIAN_POINT ( 'NONE',  ( -4.743843029824828861, 13.17239914596749450, 2.424530858944988321 ) ) ;
#6147=CARTESIAN_POINT ( 'NONE',  ( 8.512513224245308763, 13.54758718765259040, 31.28571428571428470 ) ) ;
#6150=CARTESIAN_POINT ( 'NONE',  ( 7.750357176954296712, -12.08964793087877787, 29.21024514465927879 ) ) ;
#6154=CARTESIAN_POINT ( 'NONE',  ( -1.567502665446231180, -13.91197093850540334, 45.85714285714286120 ) ) ;
#6155=CARTESIAN_POINT ( 'NONE',  ( -13.55419868402807992, -4.742819248065651472, 46.92857142857142350 ) ) ;
#6157=CARTESIAN_POINT ( 'NONE',  ( -1.665163862719845067, -15.91362231745477374, 5.853102287516418478 ) ) ;
#6159=CARTESIAN_POINT ( 'NONE',  ( 11.60466159355862104, 11.60466159355875071, 31.50000000000001421 ) ) ;
#6167=CARTESIAN_POINT ( 'NONE',  ( -8.731428362939189114, 13.89598863503036341, 42.21428571428572241 ) ) ;
#6169=CARTESIAN_POINT ( 'NONE',  ( 11.22385875690717683, -11.40355824106234373, 25.00404056962644006 ) ) ;
#6170=CARTESIAN_POINT ( 'NONE',  ( 9.563412070810842991, 12.55071356310834219, 48.73000000000002530 ) ) ;
#6173=ORIENTED_EDGE ( 'NONE', *, *, #1838, .T. ) ;
#6174=CARTESIAN_POINT ( 'NONE',  ( 11.31370849898482334, -11.31370849898469366, 45.00000000000000711 ) ) ;
#6176=CARTESIAN_POINT ( 'NONE',  ( 8.512513224245308763, 13.54758718765259040, 7.285714285714284699 ) ) ;
#6178=CARTESIAN_POINT ( 'NONE',  ( 11.85413878919593422, 7.448449071214774619, 25.71428571428571885 ) ) ;
#6179=CARTESIAN_POINT ( 'NONE',  ( 4.503970704919991519, -13.25633410266674517, 37.43261199819787066 ) ) ;
#6181=VERTEX_POINT ( 'NONE', #10037 ) ;
#6182=CARTESIAN_POINT ( 'NONE',  ( -4.619798703721853528, -13.59724543428036725, 48.06738800180213644 ) ) ;
#6185=CARTESIAN_POINT ( 'NONE',  ( 13.96533075980324234, -8.621071003556521006, 16.78167371608784819 ) ) ;
#6186=CARTESIAN_POINT ( 'NONE',  ( -8.731428362939187338, 13.89598863503036164, 6.214285714285717077 ) ) ;
#6189=CARTESIAN_POINT ( 'NONE',  ( 8.841785722321695573, -13.82664651025757152, 29.21024514465927879 ) ) ;
#6194=CARTESIAN_POINT ( 'NONE',  ( -4.503970704919988854, 13.25633410266674517, 40.43261199819787066 ) ) ;
#6196=CARTESIAN_POINT ( 'NONE',  ( 1.441234910513245149, 13.92619789766829008, 8.853102287516419366 ) ) ;
#6198=CARTESIAN_POINT ( 'NONE',  ( 15.89939535829187278, 1.791431617653015174, 32.14285714285714590 ) ) ;
#6200=CARTESIAN_POINT ( 'NONE',  ( -7.340858601237953529, -11.92174236212700222, 30.28167371608785530 ) ) ;
#6204=CARTESIAN_POINT ( 'NONE',  ( -13.61519076058348254, -8.404922754268771001, 44.71832628391215536 ) ) ;
#6205=CARTESIAN_POINT ( 'NONE',  ( -4.503970704919988854, 13.25633410266674517, 10.43261199819786356 ) ) ;
#6206=CARTESIAN_POINT ( 'NONE',  ( -10.15407889436378852, -10.15407889436390576, 46.50000000000002132 ) ) ;
#6208=CARTESIAN_POINT ( 'NONE',  ( 5.297344310588354865, 15.53355953199867301, 15.06738800180213822 ) ) ;
#6210=CARTESIAN_POINT ( 'NONE',  ( -8.731428362939189114, 13.89598863503036341, 42.21428571428572241 ) ) ;
#6217=CARTESIAN_POINT ( 'NONE',  ( 1.791431617652837316, 15.89939535829188877, 36.85714285714286120 ) ) ;
#6219=CARTESIAN_POINT ( 'NONE',  ( 1.917699372585825790, 15.88516839912900203, 22.86118342676929061 ) ) ;
#6220=CARTESIAN_POINT ( 'NONE',  ( 11.31370849898482334, -11.31370849898469366, 15.00000000000000000 ) ) ;
#6223=CARTESIAN_POINT ( 'NONE',  ( -1.837501619626328297, 16.30827793483733856, 0.6428571428571432378 ) ) ;
#6224=CARTESIAN_POINT ( 'NONE',  ( 5.420364854932000931, 15.49051278174644075, 43.07142857142857650 ) ) ;
#6227=CARTESIAN_POINT ( 'NONE',  ( 5.420364854932001819, 15.49051278174644430, 1.071428571428570287 ) ) ;
#6229=CARTESIAN_POINT ( 'NONE',  ( -13.55419868402807992, -4.742819248065651472, 34.92857142857143771 ) ) ;
#6232=CARTESIAN_POINT ( 'NONE',  ( 7.340858601237956194, 11.92174236212700045, 39.28167371608785174 ) ) ;
#6233=CARTESIAN_POINT ( 'NONE',  ( 15.89939535829187278, 1.791431617653015174, 2.142857142857140573 ) ) ;
#6235=CARTESIAN_POINT ( 'NONE',  ( -15.44746603149413922, -5.543385399275820191, 18.92453085894499409 ) ) ;
#6236=CARTESIAN_POINT ( 'NONE',  ( -8.512513224245306986, -13.54758718765259218, 10.28571428571428648 ) ) ;
#6238=CARTESIAN_POINT ( 'NONE',  ( 1.967016585148662289, -16.29368510291087091, 29.63881657323071295 ) ) ;
#6244=CARTESIAN_POINT ( 'NONE',  ( 4.619798703721856192, 13.59724543428036725, 3.067388001802140884 ) ) ;
#6245=APPLICATION_CONTEXT ( 'automotive_design' ) ;
#6247=CARTESIAN_POINT ( 'NONE',  ( 13.54758718765249803, 8.512513224245457977, 13.71428571428571352 ) ) ;
#6253=CARTESIAN_POINT ( 'NONE',  ( 11.92174236212692229, 7.340858601238088532, 5.718326283912152697 ) ) ;
#6254=CARTESIAN_POINT ( 'NONE',  ( 13.17239914596754424, -4.743843029824685864, 0.5754691410550027975 ) ) ;
#6256=CARTESIAN_POINT ( 'NONE',  ( 13.96533075980324234, -8.621071003556521006, 4.781673716087850856 ) ) ;
#6258=CARTESIAN_POINT ( 'NONE',  ( -8.512513224245306986, -13.54758718765259218, 46.28571428571429180 ) ) ;
#6263=CARTESIAN_POINT ( 'NONE',  ( -1.917699372585823570, -15.88516839912900558, 31.86118342676929416 ) ) ;
#6264=CARTESIAN_POINT ( 'NONE',  ( 1.707986654103998303, -16.32287076676380266, 37.64689771248358596 ) ) ;
#6268=CARTESIAN_POINT ( 'NONE',  ( 1.791431617652837316, 15.89939535829188877, 12.85714285714285943 ) ) ;
#6271=CARTESIAN_POINT ( 'NONE',  ( 16.30827793483735633, -1.837501619626142890, 2.357142857142856762 ) ) ;
#6273=MECHANICAL_DESIGN_GEOMETRIC_PRESENTATION_REPRESENTATION('',(#9437),#4476);
#6277=CARTESIAN_POINT ( 'NONE',  ( 11.60466159355862104, 11.60466159355875071, 7.500000000000005329 ) ) ;
#6278=CARTESIAN_POINT ( 'NONE',  ( 8.731428362939190890, -13.89598863503036164, 15.21428571428571530 ) ) ;
#6279=CARTESIAN_POINT ( 'NONE',  ( -10.15407889436378852, -10.15407889436390398, 34.50000000000000000 ) ) ;
#6283=CARTESIAN_POINT ( 'NONE',  ( 9.899494936611718643, -9.899494936611608509, 9.000000000000001776 ) ) ;
#6286=CARTESIAN_POINT ( 'NONE',  ( -16.32287076676382398, 1.707986654103809343, 31.35310228751642470 ) ) ;
#6287=CARTESIAN_POINT ( 'NONE',  ( 1.837501619626329630, -16.30827793483733501, 9.642857142857144126 ) ) ;
#6288=CARTESIAN_POINT ( 'NONE',  ( 5.404401153735178376, -15.06016580658422477, 23.42453085894499409 ) ) ;
#6296=CARTESIAN_POINT ( 'NONE',  ( 7.750357176954296712, -12.08964793087877787, 17.21024514465927879 ) ) ;
#6298=CARTESIAN_POINT ( 'NONE',  ( -15.89939535829186923, -1.791431617653016062, 11.14285714285714235 ) ) ;
#6300=CARTESIAN_POINT ( 'NONE',  ( -7.750357176954294935, 12.08964793087877787, 32.21024514465928235 ) ) ;
#6304=CARTESIAN_POINT ( 'NONE',  ( -4.865839792409144771, -13.51115193377589740, 2.075469141055009015 ) ) ;
#6306=CARTESIAN_POINT ( 'NONE',  ( 9.809645194534072132, -9.989344678689256796, 19.00404056962642940 ) ) ;
#6307=EDGE_LOOP ( 'NONE', ( #2766, #9048, #6585, #2139 ) ) ;
#6308=CARTESIAN_POINT ( 'NONE',  ( 15.14410076328353227, -5.164528828830166063, 16.56738800180213289 ) ) ;
#6310=CARTESIAN_POINT ( 'NONE',  ( -8.731428362939189114, 13.89598863503036341, 48.21428571428570820 ) ) ;
#6317=CARTESIAN_POINT ( 'NONE',  ( -16.29368510291090288, 1.967016585148476215, 39.36118342676930837 ) ) ;
#6319=CARTESIAN_POINT ( 'NONE',  ( -13.89598863503046111, 8.731428362939027465, 17.78571428571428115 ) ) ;
#6321=CARTESIAN_POINT ( 'NONE',  ( 11.09109556827038467, 11.02177121192640818, 48.73000000000001819 ) ) ;
#6323=CARTESIAN_POINT ( 'NONE',  ( -11.31370849898482156, 11.31370849898469544, 0.000000000000000000 ) ) ;
#6328=CARTESIAN_POINT ( 'NONE',  ( 15.53355953199861794, 5.297344310588528060, -0.06738800180213055935 ) ) ;
#6329=CARTESIAN_POINT ( 'NONE',  ( 15.49051278174638036, 5.420364854932175014, 19.92857142857143771 ) ) ;
#6331=CARTESIAN_POINT ( 'NONE',  ( 7.448449071214646722, 11.85413878919601594, 37.28571428571429180 ) ) ;
#6332=CARTESIAN_POINT ( 'NONE',  ( -1.478298951650703019, 14.28433602490913579, 34.64689771248358596 ) ) ;
#6336=CARTESIAN_POINT ( 'NONE',  ( -9.899494936611716867, 9.899494936611610285, 0.000000000000000000 ) ) ;
#6339=CARTESIAN_POINT ( 'NONE',  ( 8.731428362939189114, -13.89598863503035986, 15.21428571428571708 ) ) ;
#6340=CARTESIAN_POINT ( 'NONE',  ( -11.51250119794888072, -11.69682198916848037, 24.49595943037356705 ) ) ;
#6346=CARTESIAN_POINT ( 'NONE',  ( 15.10213328493390783, -5.284464991282587398, 32.57142857142856940 ) ) ;
#6348=CARTESIAN_POINT ( 'NONE',  ( -10.06191849875405531, -10.24623928997363542, 18.49595943037356705 ) ) ;
#6350=CARTESIAN_POINT ( 'NONE',  ( 15.89939535829187278, 1.791431617653015174, 14.14285714285714413 ) ) ;
#6356=CARTESIAN_POINT ( 'NONE',  ( 7.529642458189280241, -12.22833218042435099, 7.218326283912148256 ) ) ;
#6357=CARTESIAN_POINT ( 'NONE',  ( -13.92619789766827054, -1.441234910513399470, 9.146897712483580634 ) ) ;
#6361=CARTESIAN_POINT ( 'NONE',  ( -5.284464991282755264, 15.10213328493384743, 48.42857142857143060 ) ) ;
#6366=CARTESIAN_POINT ( 'NONE',  ( 13.82664651025767100, -8.841785722321541030, 24.78975485534072476 ) ) ;
#6368=CARTESIAN_POINT ( 'NONE',  ( -13.82664651025767100, 8.841785722321537477, 39.78975485534073186 ) ) ;
#6371=CARTESIAN_POINT ( 'NONE',  ( -11.31370849898482156, 11.31370849898469544, 36.00000000000000711 ) ) ;
#6372=CARTESIAN_POINT ( 'NONE',  ( -7.848420429648667707, 11.63161085820113527, -5.255698201876048165E-17 ) ) ;
#6373=ORIENTED_EDGE ( 'NONE', *, *, #6893, .T. ) ;
#6374=CARTESIAN_POINT ( 'NONE',  ( 15.49051278174638036, 5.420364854932175014, 7.928571428571430602 ) ) ;
#6375=PRESENTATION_STYLE_ASSIGNMENT (( #82 ) ) ;
#6378=CARTESIAN_POINT ( 'NONE',  ( -7.529642458189277576, 12.22833218042435455, 40.21832628391215536 ) ) ;
#6379=CARTESIAN_POINT ( 'NONE',  ( 5.420364854932001819, 15.49051278174644430, 19.07142857142856940 ) ) ;
#6380=CARTESIAN_POINT ( 'NONE',  ( 4.623906867372411078, -13.21436662431711717, 39.42857142857143060 ) ) ;
#6381=CARTESIAN_POINT ( 'NONE',  ( -1.707986654103994528, 16.32287076676380266, -1.353102287516420921 ) ) ;
#6382=CARTESIAN_POINT ( 'NONE',  ( -10.15407889436378852, -10.15407889436390576, 10.50000000000000533 ) ) ;
#6386=CARTESIAN_POINT ( 'NONE',  ( -12.15899005565164792, 7.639999817571651697, 5.785714285714282035 ) ) ;
#6388=CARTESIAN_POINT ( 'NONE',  ( -10.60660171779826833, 10.60660171779815286, 0.000000000000000000 ) ) ;
#6389=( GEOMETRIC_REPRESENTATION_CONTEXT ( 3 ) GLOBAL_UNCERTAINTY_ASSIGNED_CONTEXT ( ( #3287 ) ) GLOBAL_UNIT_ASSIGNED_CONTEXT ( ( #7007, #6897, #1440 ) ) REPRESENTATION_CONTEXT ( 'NONE', 'WORKASPACE' ) );
#6390=CARTESIAN_POINT ( 'NONE',  ( 8.512513224245308763, 13.54758718765259040, 19.28571428571428825 ) ) ;
#6391=CARTESIAN_POINT ( 'NONE',  ( -15.14410076328353227, 5.164528828830164287, 43.56738800180213644 ) ) ;
#6396=CARTESIAN_POINT ( 'NONE',  ( 13.47998361472151529, 8.620103694222146729, 27.71024514465928235 ) ) ;
#6398=CARTESIAN_POINT ( 'NONE',  ( -7.340858601237953529, -11.92174236212700222, 18.28167371608785174 ) ) ;
#6400=CARTESIAN_POINT ( 'NONE',  ( -15.49051278174638036, -5.420364854932175902, 10.92857142857142883 ) ) ;
#6402=CARTESIAN_POINT ( 'NONE',  ( -14.28433602490915000, 1.478298951650542481, 43.35310228751642825 ) ) ;
#6406=CARTESIAN_POINT ( 'NONE',  ( 4.503970704919991519, -13.25633410266674517, 1.432611998197868219 ) ) ;
#6408=CARTESIAN_POINT ( 'NONE',  ( -14.25515036105622890, 1.737328882695209575, 9.361183426769292382 ) ) ;
#6411=CARTESIAN_POINT ( 'NONE',  ( 5.284464991282756152, -15.10213328493384743, 39.42857142857143060 ) ) ;
#6417=CARTESIAN_POINT ( 'NONE',  ( -5.543385399275643444, -15.44746603149420494, 26.07546914105500235 ) ) ;
#6420=CARTESIAN_POINT ( 'NONE',  ( -15.53355953199861794, -5.297344310588530725, 26.93261199819786356 ) ) ;
#6423=CARTESIAN_POINT ( 'NONE',  ( -5.284464991282755264, 15.10213328493384743, 36.42857142857143060 ) ) ;
#6424=CARTESIAN_POINT ( 'NONE',  ( 3.834211569871422309, 14.40628620492435630, -1.793508096673564591E-16 ) ) ;
#6425=CARTESIAN_POINT ( 'NONE',  ( -8.731428362939189114, 13.89598863503036341, 6.214285714285717965 ) ) ;
#6429=CARTESIAN_POINT ( 'NONE',  ( -13.17239914596754424, 4.743843029824683200, 45.57546914105501656 ) ) ;
#6431=CARTESIAN_POINT ( 'NONE',  ( -8.731428362939189114, 13.89598863503036341, 18.21428571428571885 ) ) ;
#6432=CARTESIAN_POINT ( 'NONE',  ( -13.21436662431716869, 4.623906867372262752, 41.57142857142856940 ) ) ;
#6433=CARTESIAN_POINT ( 'NONE',  ( -13.92619789766827054, -1.441234910513399470, 39.14689771248358596 ) ) ;
#6434=CARTESIAN_POINT ( 'NONE',  ( -7.639999817571787588, 12.15899005565156266, 6.214285714285717965 ) ) ;
#6438=CARTESIAN_POINT ( 'NONE',  ( -12.22833218042443271, 7.529642458189139909, 49.78167371608785885 ) ) ;
#6444=CARTESIAN_POINT ( 'NONE',  ( -5.284464991282755264, 15.10213328493384743, 18.42857142857143415 ) ) ;
#6445=CARTESIAN_POINT ( 'NONE',  ( -15.88516839912898071, -1.917699372586004980, 31.13881657323070939 ) ) ;
#6451=CARTESIAN_POINT ( 'NONE',  ( -7.750357176954294935, 12.08964793087877787, 20.21024514465928235 ) ) ;
#6454=CARTESIAN_POINT ( 'NONE',  ( 8.512513224245308763, 13.54758718765259040, 37.28571428571429180 ) ) ;
#6455=CARTESIAN_POINT ( 'NONE',  ( 10.06191849875406064, 10.24623928997363187, 45.49595943037356705 ) ) ;
#6459=CARTESIAN_POINT ( 'NONE',  ( 7.556039541191335474, 11.78653521626503320, 17.28975485534072121 ) ) ;
#6461=CARTESIAN_POINT ( 'NONE',  ( -7.529642458189277576, 12.22833218042435455, 10.21832628391215358 ) ) ;
#6464=CARTESIAN_POINT ( 'NONE',  ( -11.51250119794888072, -11.69682198916848037, 12.49595943037356349 ) ) ;
#6471=CARTESIAN_POINT ( 'NONE',  ( 13.55419868402807992, 4.742819248065648807, 31.92857142857143415 ) ) ;
#6472=CARTESIAN_POINT ( 'NONE',  ( -5.164528828830334817, 15.14410076328347543, 28.43261199819786356 ) ) ;
#6474=CARTESIAN_POINT ( 'NONE',  ( 15.49051278174638036, 5.420364854932175014, 25.92857142857142705 ) ) ;
#6476=CARTESIAN_POINT ( 'NONE',  ( -8.512513224245306986, -13.54758718765259218, 16.28571428571428470 ) ) ;
#6480=CARTESIAN_POINT ( 'NONE',  ( 4.865839792409144771, 13.51115193377589740, 47.07546914105501656 ) ) ;
#6481=CARTESIAN_POINT ( 'NONE',  ( 1.837501619626330074, -16.30827793483733501, 15.64285714285714235 ) ) ;
#6483=CARTESIAN_POINT ( 'NONE',  ( -7.529642458189277576, 12.22833218042435455, 40.21832628391215536 ) ) ;
#6485=CARTESIAN_POINT ( 'NONE',  ( 12.15899005565164792, -7.639999817571655250, 14.78571428571429358 ) ) ;
#6489=CARTESIAN_POINT ( 'NONE',  ( 10.15407889436379030, 10.15407889436390576, 1.500000000000003553 ) ) ;
#6492=CARTESIAN_POINT ( 'NONE',  ( 16.30827793483735633, -1.837501619626142890, 14.35714285714285587 ) ) ;
#6493=CARTESIAN_POINT ( 'NONE',  ( -11.51250119794888072, -11.69682198916848037, 36.49595943037355994 ) ) ;
#6496=CARTESIAN_POINT ( 'NONE',  ( -4.742819248065500481, -13.55419868402813499, 4.071428571428569398 ) ) ;
#6497=CARTESIAN_POINT ( 'NONE',  ( 9.989344678689365153, -9.809645194533958446, 16.99595943037355994 ) ) ;
#6500=CARTESIAN_POINT ( 'NONE',  ( -9.989344678689363377, 9.809645194533960222, 43.99595943037355994 ) ) ;
#6503=EDGE_CURVE ( 'NONE', #3093, #7090, #4692, .T. ) ;
#6505=CARTESIAN_POINT ( 'NONE',  ( 13.59724543428031573, 4.619798703722006294, 23.93261199819786711 ) ) ;
#6506=CARTESIAN_POINT ( 'NONE',  ( 13.92619789766827587, 1.441234910513398582, 12.14689771248358063 ) ) ;
#6509=CARTESIAN_POINT ( 'NONE',  ( 8.841785722321695573, -13.82664651025757152, 11.21024514465928235 ) ) ;
#6515=CARTESIAN_POINT ( 'NONE',  ( -15.06016580658428694, 5.404401153735006957, 39.57546914105500946 ) ) ;
#6516=CARTESIAN_POINT ( 'NONE',  ( -12.15899005565164792, 7.639999817571651697, 23.78571428571429536 ) ) ;
#6517=CARTESIAN_POINT ( 'NONE',  ( 16.29368510291089223, -1.967016585148476882, 42.36118342676930126 ) ) ;
#6519=CARTESIAN_POINT ( 'NONE',  ( -8.512513224245306986, -13.54758718765259218, 28.28571428571428825 ) ) ;
#6520=CARTESIAN_POINT ( 'NONE',  ( 3.104357715559908915, 14.35744100736050655, 7.004981435163800088E-16 ) ) ;
#6521=CARTESIAN_POINT ( 'NONE',  ( -1.791431617652833763, -15.89939535829188877, 15.85714285714286120 ) ) ;
#6523=CARTESIAN_POINT ( 'NONE',  ( 1.027016091380565710, 17.97067716999126219, 48.73000000000001819 ) ) ;
#6526=CARTESIAN_POINT ( 'NONE',  ( -9.809645194534070356, 9.989344678689256796, 40.00404056962644006 ) ) ;
#6527=CARTESIAN_POINT ( 'NONE',  ( 13.54758718765249803, 8.512513224245457977, 25.71428571428571885 ) ) ;
#6529=CARTESIAN_POINT ( 'NONE',  ( -7.639999817571786700, 12.15899005565156266, 48.21428571428571530 ) ) ;
#6530=CARTESIAN_POINT ( 'NONE',  ( -4.865839792409144771, -13.51115193377589740, 44.07546914105503078 ) ) ;
#6531=CARTESIAN_POINT ( 'NONE',  ( 1.607813917173038121, -14.26974319298267346, 15.64285714285714235 ) ) ;
#6535=CARTESIAN_POINT ( 'NONE',  ( -10.15407889436378852, -10.15407889436390576, 22.50000000000000000 ) ) ;
#6537=FACE_OUTER_BOUND ( 'NONE', #378, .T. ) ;
#6538=CARTESIAN_POINT ( 'NONE',  ( -15.49051278174637858, -5.420364854932175014, 16.92857142857143060 ) ) ;
#6540=CARTESIAN_POINT ( 'NONE',  ( -5.404401153735176599, 15.06016580658422477, 38.42453085894499054 ) ) ;
#6543=CARTESIAN_POINT ( 'NONE',  ( 14.26974319298268767, -1.607813917172876472, 14.35714285714285587 ) ) ;
#6544=CARTESIAN_POINT ( 'NONE',  ( -13.25633410266679313, 4.503970704919840529, 31.56738800180213644 ) ) ;
#6546=CARTESIAN_POINT ( 'NONE',  ( -16.30827793483735988, 1.837501619626141780, 17.35714285714286476 ) ) ;
#6548=CARTESIAN_POINT ( 'NONE',  ( -4.619798703721853528, -13.59724543428036725, 36.06738800180213644 ) ) ;
#6553=CARTESIAN_POINT ( 'NONE',  ( -1.693770420379220099, -13.89774397934251837, 25.86118342676929416 ) ) ;
#6558=CARTESIAN_POINT ( 'NONE',  ( 13.47998361472151529, 8.620103694222146729, 3.710245144659281458 ) ) ;
#6564=CARTESIAN_POINT ( 'NONE',  ( 13.91197093850538380, 1.567502665446386390, 32.14285714285714590 ) ) ;
#6566=VERTEX_POINT ( 'NONE', #5170 ) ;
#6567=CARTESIAN_POINT ( 'NONE',  ( -13.89598863503046111, 8.731428362939027465, 29.78571428571428825 ) ) ;
#6569=CARTESIAN_POINT ( 'NONE',  ( -15.49051278174638036, -5.420364854932175902, 16.92857142857143771 ) ) ;
#6575=CARTESIAN_POINT ( 'NONE',  ( -5.543385399275643444, -15.44746603149420494, 8.075469141055007682 ) ) ;
#6576=CARTESIAN_POINT ( 'NONE',  ( 1.837501619626330074, -16.30827793483733501, 33.64285714285715301 ) ) ;
#6578=CARTESIAN_POINT ( 'NONE',  ( 1.917699372585825790, 15.88516839912900203, 4.861183426769296823 ) ) ;
#6580=CARTESIAN_POINT ( 'NONE',  ( -13.21436662431716869, 4.623906867372262752, 11.57142857142857295 ) ) ;
#6584=CARTESIAN_POINT ( 'NONE',  ( 12.15899005565164792, -7.639999817571655250, 14.78571428571429358 ) ) ;
#6585=ORIENTED_EDGE ( 'NONE', *, *, #3459, .T. ) ;
#6586=CARTESIAN_POINT ( 'NONE',  ( 11.31370849898482334, -11.31370849898469366, 33.00000000000000000 ) ) ;
#6589=CARTESIAN_POINT ( 'NONE',  ( -13.96533075980324234, 8.621071003556515677, 37.78167371608785174 ) ) ;
#6591=CARTESIAN_POINT ( 'NONE',  ( 7.639999817571788476, -12.15899005565156266, 15.21428571428571708 ) ) ;
#6595=CARTESIAN_POINT ( 'NONE',  ( 10.06191849875406064, 10.24623928997363187, 33.49595943037355994 ) ) ;
#6598=CARTESIAN_POINT ( 'NONE',  ( -13.51115193377584589, -4.865839792409295761, 36.92453085894499765 ) ) ;
#6604=CARTESIAN_POINT ( 'NONE',  ( -13.96533075980324234, 8.621071003556515677, 37.78167371608785174 ) ) ;
#6605=CARTESIAN_POINT ( 'NONE',  ( -13.13091431946350163, 7.193069072976622458, 48.73000000000003240 ) ) ;
#6607=CARTESIAN_POINT ( 'NONE',  ( 5.297344310588354865, 15.53355953199867301, 3.067388001802140884 ) ) ;
#6612=CARTESIAN_POINT ( 'NONE',  ( -1.917699372585823570, -15.88516839912900558, 37.86118342676929416 ) ) ;
#6613=CARTESIAN_POINT ( 'NONE',  ( 4.623906867372411078, -13.21436662431711717, 27.42857142857143060 ) ) ;
#6615=CARTESIAN_POINT ( 'NONE',  ( -13.55419868402807992, -4.742819248065651472, 40.92857142857145192 ) ) ;
#6617=CARTESIAN_POINT ( 'NONE',  ( -15.49051278174638036, -5.420364854932175902, 40.92857142857145192 ) ) ;
#6618=CARTESIAN_POINT ( 'NONE',  ( 2.511715608995780613, 15.22804288820251806, -2.187087473825319915E-16 ) ) ;
#6619=CARTESIAN_POINT ( 'NONE',  ( 8.731428362939190890, -13.89598863503036164, 21.21428571428571885 ) ) ;
#6624=CARTESIAN_POINT ( 'NONE',  ( -1.707986654103994528, 16.32287076676380266, 4.646897712483579745 ) ) ;
#6625=CARTESIAN_POINT ( 'NONE',  ( -13.54758718765249625, -8.512513224245459753, 28.71428571428571530 ) ) ;
#6627=CARTESIAN_POINT ( 'NONE',  ( -11.69682198916834892, -11.51250119794901394, 8.504040569626438284 ) ) ;
#6630=CARTESIAN_POINT ( 'NONE',  ( -1.607813917173034124, 14.26974319298267524, 24.64285714285714235 ) ) ;
#6631=CARTESIAN_POINT ( 'NONE',  ( -11.31370849898482156, 11.31370849898469544, 5.999999999999998224 ) ) ;
#6634=CARTESIAN_POINT ( 'NONE',  ( -12.15899005565164792, 7.639999817571651697, 11.78571428571428115 ) ) ;
#6636=CARTESIAN_POINT ( 'NONE',  ( -15.89939535829186923, -1.791431617653016062, 29.14285714285714235 ) ) ;
#6637=CARTESIAN_POINT ( 'NONE',  ( -4.743843029824828861, 13.17239914596749450, 2.424530858944988321 ) ) ;
#6640=CARTESIAN_POINT ( 'NONE',  ( -1.607813917173034124, 14.26974319298267346, 12.64285714285714235 ) ) ;
#6641=CARTESIAN_POINT ( 'NONE',  ( 13.89774397934249706, 1.693770420379375308, 34.13881657323070584 ) ) ;
#6646=CARTESIAN_POINT ( 'NONE',  ( 1.567502665446232957, 13.91197093850540156, 0.8571428571428549859 ) ) ;
#6651=CARTESIAN_POINT ( 'NONE',  ( -7.556039541191334585, -11.78653521626503320, 20.28975485534072121 ) ) ;
#6653=CARTESIAN_POINT ( 'NONE',  ( 1.967016585148662289, -16.29368510291087091, 41.63881657323070584 ) ) ;
#6655=CARTESIAN_POINT ( 'NONE',  ( -1.639859883600667700, 13.92277000329989534, 48.73000000000004661 ) ) ;
#6657=EDGE_CURVE ( 'NONE', #7090, #6853, #7307, .T. ) ;
#6662=CARTESIAN_POINT ( 'NONE',  ( -1.607813917173034124, 14.26974319298267524, 24.64285714285714235 ) ) ;
#6663=CARTESIAN_POINT ( 'NONE',  ( 13.55419868402807992, 4.742819248065648807, 43.92857142857143060 ) ) ;
#6665=CARTESIAN_POINT ( 'NONE',  ( -8.731428362939189114, 13.89598863503036341, 42.21428571428572241 ) ) ;
#6667=CARTESIAN_POINT ( 'NONE',  ( -5.420364854931999155, -15.49051278174644253, 16.07142857142857650 ) ) ;
#6671=CARTESIAN_POINT ( 'NONE',  ( -13.82664651025767100, 8.841785722321537477, 9.789754855340722983 ) ) ;
#6672=CARTESIAN_POINT ( 'NONE',  ( -15.49051278174638036, -5.420364854932175902, 28.92857142857143771 ) ) ;
#6673=CARTESIAN_POINT ( 'NONE',  ( -15.91362231745475597, -1.665163862720028254, 9.146897712483580634 ) ) ;
#6674=CARTESIAN_POINT ( 'NONE',  ( 13.21436662431716869, -4.623906867372263640, 26.57142857142857295 ) ) ;
#6675=CARTESIAN_POINT ( 'NONE',  ( 5.420364854932001819, 15.49051278174644430, 1.071428571428570287 ) ) ;
#6678=CARTESIAN_POINT ( 'NONE',  ( 7.448449071214646722, 11.85413878919601594, 13.28571428571429003 ) ) ;
#6681=CARTESIAN_POINT ( 'NONE',  ( -5.284464991282755264, 15.10213328493384743, 36.42857142857143060 ) ) ;
#6682=CARTESIAN_POINT ( 'NONE',  ( -9.989344678689363377, 9.809645194533960222, 1.995959430373561272 ) ) ;
#6685=CARTESIAN_POINT ( 'NONE',  ( 9.899494936611718643, -9.899494936611608509, 9.000000000000001776 ) ) ;
#6688=CARTESIAN_POINT ( 'NONE',  ( 4.619798703721856192, 13.59724543428036725, 21.06738800180213644 ) ) ;
#6696=CARTESIAN_POINT ( 'NONE',  ( -1.693770420379220099, -13.89774397934251837, 31.86118342676929416 ) ) ;
#6699=CARTESIAN_POINT ( 'NONE',  ( -5.297344310588352201, -15.53355953199867301, 36.06738800180213644 ) ) ;
#6700=CARTESIAN_POINT ( 'NONE',  ( -3.566842584106372893, 15.58126113556745551, 48.73000000000023135 ) ) ;
#6701=CARTESIAN_POINT ( 'NONE',  ( -13.54758718765249625, -8.512513224245459753, 22.71428571428571530 ) ) ;
#6705=CARTESIAN_POINT ( 'NONE',  ( -1.441234910513241818, -13.92619789766829008, 17.85310228751642114 ) ) ;
#6709=CARTESIAN_POINT ( 'NONE',  ( -4.623906867372410190, 13.21436662431711895, 48.42857142857143060 ) ) ;
#6710=CARTESIAN_POINT ( 'NONE',  ( 13.21436662431716869, -4.623906867372263640, 32.57142857142856940 ) ) ;
#6713=CARTESIAN_POINT ( 'NONE',  ( 15.89939535829187278, 1.791431617653015174, 38.14285714285714590 ) ) ;
#6715=CARTESIAN_POINT ( 'NONE',  ( 1.791431617652837316, 15.89939535829188877, 30.85714285714286120 ) ) ;
#6722=CARTESIAN_POINT ( 'NONE',  ( -8.620103694221995738, -13.47998361472161299, 8.289754855340721207 ) ) ;
#6723=CARTESIAN_POINT ( 'NONE',  ( -11.31370849898482156, 11.31370849898469544, 30.00000000000000355 ) ) ;
#6724=CARTESIAN_POINT ( 'NONE',  ( -13.61519076058348254, -8.404922754268771001, 2.718326283912150476 ) ) ;
#6725=CARTESIAN_POINT ( 'NONE',  ( 1.607813917173038121, -14.26974319298267346, 21.64285714285714590 ) ) ;
#6726=CARTESIAN_POINT ( 'NONE',  ( 11.60466159355862104, 11.60466159355875071, 7.500000000000005329 ) ) ;
#6727=CARTESIAN_POINT ( 'NONE',  ( 5.420364854932001819, 15.49051278174644430, 43.07142857142858361 ) ) ;
#6729=CARTESIAN_POINT ( 'NONE',  ( 13.21436662431716869, -4.623906867372263640, 20.57142857142857295 ) ) ;
#6731=CARTESIAN_POINT ( 'NONE',  ( -13.54758718765249625, -8.512513224245459753, 28.71428571428571530 ) ) ;
#6732=CARTESIAN_POINT ( 'NONE',  ( 5.297344310588354865, 15.53355953199867301, 45.06738800180215065 ) ) ;
#6735=CARTESIAN_POINT ( 'NONE',  ( -4.623906867372410190, 13.21436662431711895, 12.42857142857142705 ) ) ;
#6736=CARTESIAN_POINT ( 'NONE',  ( 13.25633410266679313, -4.503970704919842305, 22.56738800180214000 ) ) ;
#6739=CARTESIAN_POINT ( 'NONE',  ( 8.672099987835544255, 11.29616555842733661, 48.73000000000003951 ) ) ;
#6741=CARTESIAN_POINT ( 'NONE',  ( 14.28433602490915000, -1.478298951650544479, 46.35310228751641404 ) ) ;
#6745=CARTESIAN_POINT ( 'NONE',  ( -9.809645194534070356, 9.989344678689256796, 34.00404056962644006 ) ) ;
#6751=CARTESIAN_POINT ( 'NONE',  ( -15.14410076328353227, 5.164528828830164287, 37.56738800180213644 ) ) ;
#6752=CARTESIAN_POINT ( 'NONE',  ( -11.48558320758131401, 8.816166900624141434, 48.73000000000002530 ) ) ;
#6753=CARTESIAN_POINT ( 'NONE',  ( 1.837501619626330074, -16.30827793483733501, 21.64285714285714590 ) ) ;
#6757=CARTESIAN_POINT ( 'NONE',  ( -11.78653521626494793, -7.556039541191465148, 18.71024514465927879 ) ) ;
#6761=CARTESIAN_POINT ( 'NONE',  ( 1.917699372585825790, 15.88516839912900203, 40.86118342676929416 ) ) ;
#6762=CARTESIAN_POINT ( 'NONE',  ( 1.693770420379222319, 13.89774397934251837, -1.138816573230706286 ) ) ;
#6764=CARTESIAN_POINT ( 'NONE',  ( 13.55419868402807992, 4.742819248065648807, 31.92857142857143415 ) ) ;
#6766=CARTESIAN_POINT ( 'NONE',  ( -16.30827793483735988, 1.837501619626141780, 41.35714285714286120 ) ) ;
#6768=CARTESIAN_POINT ( 'NONE',  ( -15.10213328493390961, 5.284464991282586510, 23.57142857142857650 ) ) ;
#6779=CARTESIAN_POINT ( 'NONE',  ( -13.61519076058348254, -8.404922754268771001, 20.71832628391214826 ) ) ;
#6780=CARTESIAN_POINT ( 'NONE',  ( 15.10213328493390783, -5.284464991282587398, 44.57142857142857650 ) ) ;
#6782=CARTESIAN_POINT ( 'NONE',  ( 13.82664651025767100, -8.841785722321541030, 18.78975485534072121 ) ) ;
#6783=CARTESIAN_POINT ( 'NONE',  ( -11.85413878919593422, -7.448449071214776396, 28.71428571428571530 ) ) ;
#6785=CARTESIAN_POINT ( 'NONE',  ( -13.54758718765249625, -8.512513224245459753, 10.71428571428571708 ) ) ;
#6786=CARTESIAN_POINT ( 'NONE',  ( -15.89939535829186923, -1.791431617653016062, 47.14285714285714590 ) ) ;
#6792=CARTESIAN_POINT ( 'NONE',  ( 13.96533075980324234, -8.621071003556521006, 46.78167371608785885 ) ) ;
#6794=CARTESIAN_POINT ( 'NONE',  ( -1.791431617652833763, -15.89939535829188877, 3.857142857142857650 ) ) ;
#6797=CARTESIAN_POINT ( 'NONE',  ( -7.448449071214644945, -11.85413878919601771, 28.28571428571428825 ) ) ;
#6798=CARTESIAN_POINT ( 'NONE',  ( -1.737328882695368115, 14.25515036105620581, 44.63881657323071295 ) ) ;
#6799=ORIENTED_EDGE ( 'NONE', *, *, #1838, .F. ) ;
#6801=CARTESIAN_POINT ( 'NONE',  ( 15.14410076328353227, -5.164528828830166063, 4.567388001802134667 ) ) ;
#6804=CARTESIAN_POINT ( 'NONE',  ( -4.623906867372410190, 13.21436662431711895, 0.4285714285714309346 ) ) ;
#6808=CARTESIAN_POINT ( 'NONE',  ( -10.24623928997352351, -10.06191849875416899, 32.50404056962644006 ) ) ;
#6811=CARTESIAN_POINT ( 'NONE',  ( 11.40355824106246985, -11.22385875690704538, 40.99595943037355994 ) ) ;
#6812=CARTESIAN_POINT ( 'NONE',  ( -13.19966323802950114, 7.266400725181457965, 48.73000000000003240 ) ) ;
#6813=CARTESIAN_POINT ( 'NONE',  ( -1.791431617652833763, -15.89939535829188877, 27.85714285714285765 ) ) ;
#6817=CARTESIAN_POINT ( 'NONE',  ( 13.51115193377584589, 4.865839792409294873, 21.92453085894500120 ) ) ;
#6821=CARTESIAN_POINT ( 'NONE',  ( -7.448449071214644945, -11.85413878919601771, 46.28571428571429180 ) ) ;
#6822=CARTESIAN_POINT ( 'NONE',  ( -9.809645194534070356, 9.989344678689256796, 4.004040569626432067 ) ) ;
#6824=CARTESIAN_POINT ( 'NONE',  ( 1.837501619626330074, -16.30827793483733501, 45.64285714285716011 ) ) ;
#6826=CARTESIAN_POINT ( 'NONE',  ( -5.284464991282755264, 15.10213328493384743, 24.42857142857143060 ) ) ;
#6832=CARTESIAN_POINT ( 'NONE',  ( -11.69682198916834892, -11.51250119794901394, 20.50404056962644006 ) ) ;
#6833=CARTESIAN_POINT ( 'NONE',  ( -1.837501619626328297, 16.30827793483733856, 36.64285714285714590 ) ) ;
#6834=CARTESIAN_POINT ( 'NONE',  ( -11.69682198916834892, -11.51250119794901394, 26.50404056962643651 ) ) ;
#6835=CARTESIAN_POINT ( 'NONE',  ( -7.639999817571787588, 12.15899005565156266, 18.21428571428571885 ) ) ;
#6838=CARTESIAN_POINT ( 'NONE',  ( 8.512513224245308763, 13.54758718765259040, 49.28571428571428470 ) ) ;
#6844=CARTESIAN_POINT ( 'NONE',  ( -15.88516839912898071, -1.917699372586004980, 49.13881657323070584 ) ) ;
#6846=CARTESIAN_POINT ( 'NONE',  ( -1.837501619626328297, 16.30827793483733856, 0.6428571428571432378 ) ) ;
#6847=CARTESIAN_POINT ( 'NONE',  ( 13.89598863503046111, -8.731428362939032795, 8.785714285714293581 ) ) ;
#6849=CARTESIAN_POINT ( 'NONE',  ( -13.55419868402807992, -4.742819248065651472, 28.92857142857143415 ) ) ;
#6850=CARTESIAN_POINT ( 'NONE',  ( 14.25515036105622535, -1.737328882695210241, 24.36118342676929416 ) ) ;
#6852=CARTESIAN_POINT ( 'NONE',  ( -4.619798703721853528, -13.59724543428036725, 42.06738800180214355 ) ) ;
#6853=VERTEX_POINT ( 'NONE', #4556 ) ;
#6855=CARTESIAN_POINT ( 'NONE',  ( -13.47998361472151174, -8.620103694222146729, 18.71024514465927879 ) ) ;
#6856=CARTESIAN_POINT ( 'NONE',  ( -1.791431617652833763, -15.89939535829188877, 3.857142857142857650 ) ) ;
#6861=CARTESIAN_POINT ( 'NONE',  ( -7.556039541191334585, -11.78653521626503320, 26.28975485534072831 ) ) ;
#6863=CARTESIAN_POINT ( 'NONE',  ( -7.750357176954294935, 12.08964793087877787, 2.210245144659280569 ) ) ;
#6865=CARTESIAN_POINT ( 'NONE',  ( 15.49051278174638036, 5.420364854932175014, 25.92857142857142705 ) ) ;
#6868=CARTESIAN_POINT ( 'NONE',  ( -10.06191849875405531, -10.24623928997363542, 12.49595943037356349 ) ) ;
#6872=CARTESIAN_POINT ( 'NONE',  ( 5.164528828830335705, -15.14410076328347543, 43.43261199819787066 ) ) ;
#6873=CARTESIAN_POINT ( 'NONE',  ( 1.607813917173038121, -14.26974319298267346, 45.64285714285716011 ) ) ;
#6874=CARTESIAN_POINT ( 'NONE',  ( 4.865839792409144771, 13.51115193377589740, -0.9245308589449906522 ) ) ;
#6876=CARTESIAN_POINT ( 'NONE',  ( -11.51250119794888072, -11.69682198916848037, 6.495959430373559051 ) ) ;
#6878=CARTESIAN_POINT ( 'NONE',  ( 16.30827793483735633, -1.837501619626142890, 26.35714285714285765 ) ) ;
#6879=MECHANICAL_DESIGN_GEOMETRIC_PRESENTATION_REPRESENTATION('',(#4253),#6389);
#6886=CARTESIAN_POINT ( 'NONE',  ( -8.512513224245306986, -13.54758718765259218, 46.28571428571429180 ) ) ;
#6888=CARTESIAN_POINT ( 'NONE',  ( 1.707986654103998303, -16.32287076676380266, 19.64689771248358596 ) ) ;
#6890=CARTESIAN_POINT ( 'NONE',  ( -8.512513224245306986, -13.54758718765259218, 22.28571428571428470 ) ) ;
#6891=CARTESIAN_POINT ( 'NONE',  ( -1.837501619626328297, 16.30827793483733856, 48.64285714285716011 ) ) ;
#6893=EDGE_CURVE ( 'NONE', #6181, #7160, #3498, .T. ) ;
#6896=CARTESIAN_POINT ( 'NONE',  ( -16.30827793483735988, 1.837501619626141558, 41.35714285714286120 ) ) ;
#6897=( NAMED_UNIT ( * ) PLANE_ANGLE_UNIT ( ) SI_UNIT ( $, .RADIAN. ) );
#6899=CARTESIAN_POINT ( 'NONE',  ( 8.731428362939190890, -13.89598863503036164, 9.214285714285717077 ) ) ;
#6900=CARTESIAN_POINT ( 'NONE',  ( 8.731428362939190890, -13.89598863503036164, 3.214285714285716633 ) ) ;
#6902=CARTESIAN_POINT ( 'NONE',  ( 13.91197093850538380, 1.567502665446386390, 26.14285714285714590 ) ) ;
#6903=CARTESIAN_POINT ( 'NONE',  ( -9.809645194534070356, 9.989344678689256796, 34.00404056962644006 ) ) ;
#6904=CARTESIAN_POINT ( 'NONE',  ( 13.89774397934249706, 1.693770420379375308, 40.13881657323070584 ) ) ;
#6907=CARTESIAN_POINT ( 'NONE',  ( 11.40355824106246985, -11.22385875690704538, 16.99595943037355994 ) ) ;
#6908=CARTESIAN_POINT ( 'NONE',  ( -8.512513224245306986, -13.54758718765259218, 4.285714285714288252 ) ) ;
#6910=CARTESIAN_POINT ( 'NONE',  ( 1.665163862719847732, 15.91362231745477374, 26.85310228751642470 ) ) ;
#6914=CARTESIAN_POINT ( 'NONE',  ( -11.92174236212692051, -7.340858601238089420, 32.71832628391215536 ) ) ;
#6916=CARTESIAN_POINT ( 'NONE',  ( -13.25633410266679313, 4.503970704919840529, 7.567388001802139108 ) ) ;
#6918=CARTESIAN_POINT ( 'NONE',  ( -8.731428362939189114, 13.89598863503036341, 30.21428571428572596 ) ) ;
#6920=CARTESIAN_POINT ( 'NONE',  ( 10.06191849875406064, 10.24623928997363187, 21.49595943037356705 ) ) ;
#6926=CARTESIAN_POINT ( 'NONE',  ( -8.621071003556675549, 13.96533075980314642, 46.21832628391216247 ) ) ;
#6927=CARTESIAN_POINT ( 'NONE',  ( 13.91197093850538380, 1.567502665446386390, 38.14285714285714590 ) ) ;
#6928=CARTESIAN_POINT ( 'NONE',  ( 7.639999817571789364, -12.15899005565156266, 45.21428571428572951 ) ) ;
#6931=CARTESIAN_POINT ( 'NONE',  ( -11.51250119794888072, -11.69682198916848037, 12.49595943037356349 ) ) ;
#6935=CARTESIAN_POINT ( 'NONE',  ( -15.10213328493390961, 5.284464991282586510, 29.57142857142857650 ) ) ;
#6942=CARTESIAN_POINT ( 'NONE',  ( 15.06016580658428694, -5.404401153735007846, 18.57546914105500235 ) ) ;
#6943=CARTESIAN_POINT ( 'NONE',  ( -8.731428362939189114, 13.89598863503036341, 48.21428571428570820 ) ) ;
#6947=CARTESIAN_POINT ( 'NONE',  ( -1.917699372585823570, -15.88516839912900558, 19.86118342676929416 ) ) ;
#6948=CARTESIAN_POINT ( 'NONE',  ( 15.10213328493390783, -5.284464991282587398, 20.57142857142857295 ) ) ;
#6949=CARTESIAN_POINT ( 'NONE',  ( 7.833366173951416656, 13.80014417467472398, 48.72999999999998977 ) ) ;
#6953=CARTESIAN_POINT ( 'NONE',  ( -8.512513224245306986, -13.54758718765259218, 46.28571428571429180 ) ) ;
#6956=CARTESIAN_POINT ( 'NONE',  ( -13.89598863503046111, 8.731428362939027465, 5.785714285714282035 ) ) ;
#6957=CARTESIAN_POINT ( 'NONE',  ( -1.837501619626328297, 16.30827793483733856, 6.642857142857143238 ) ) ;
#6959=CARTESIAN_POINT ( 'NONE',  ( 4.742819248065502258, 13.55419868402813499, 25.07142857142857650 ) ) ;
#6960=CARTESIAN_POINT ( 'NONE',  ( -4.865839792409144771, -13.51115193377589740, 38.07546914105502367 ) ) ;
#6963=CARTESIAN_POINT ( 'NONE',  ( 7.750357176954296712, -12.08964793087877787, 47.21024514465928235 ) ) ;
#6965=PLANE ( 'NONE',  #4911 ) ;
#6966=CARTESIAN_POINT ( 'NONE',  ( 1.967016585148662289, -16.29368510291087091, 23.63881657323070939 ) ) ;
#6967=CARTESIAN_POINT ( 'NONE',  ( 5.420364854932000931, 15.49051278174644075, 7.071428571428569398 ) ) ;
#6969=CARTESIAN_POINT ( 'NONE',  ( 8.404922754268618235, 13.61519076058357491, 27.28167371608785174 ) ) ;
#6973=CARTESIAN_POINT ( 'NONE',  ( 13.59724543428031573, 4.619798703722006294, 41.93261199819787066 ) ) ;
#6975=CARTESIAN_POINT ( 'NONE',  ( 7.340858601237956194, 11.92174236212700045, 3.281673716087854409 ) ) ;
#6979=CARTESIAN_POINT ( 'NONE',  ( 16.30827793483735633, -1.837501619626142890, 26.35714285714285765 ) ) ;
#6984=CARTESIAN_POINT ( 'NONE',  ( 13.61519076058348254, 8.404922754268771001, 41.71832628391215536 ) ) ;
#6985=CARTESIAN_POINT ( 'NONE',  ( -12.08964793087886314, 7.750357176954159932, 9.789754855340722983 ) ) ;
#6986=CARTESIAN_POINT ( 'NONE',  ( -12.15899005565164792, 7.639999817571651697, 47.78571428571430602 ) ) ;
#6988=CARTESIAN_POINT ( 'NONE',  ( -5.404401153735176599, 15.06016580658422477, 14.42453085894499232 ) ) ;
#6991=CARTESIAN_POINT ( 'NONE',  ( 11.60466159355862104, 11.60466159355875071, 43.50000000000000711 ) ) ;
#6999=CARTESIAN_POINT ( 'NONE',  ( -15.49051278174638036, -5.420364854932175902, 40.92857142857145192 ) ) ;
#7001=CARTESIAN_POINT ( 'NONE',  ( 5.164528828830335705, -15.14410076328347543, 19.43261199819785645 ) ) ;
#7002=CARTESIAN_POINT ( 'NONE',  ( -1.837501619626328297, 16.30827793483733856, 18.64285714285715656 ) ) ;
#7003=CARTESIAN_POINT ( 'NONE',  ( 6.421061802350969572, 14.56668498259507949, 48.73000000000001108 ) ) ;
#7006=CARTESIAN_POINT ( 'NONE',  ( 13.54758718765249803, 8.512513224245457977, 43.71428571428572241 ) ) ;
#7007=( LENGTH_UNIT ( ) NAMED_UNIT ( * ) SI_UNIT ( .MILLI., .METRE. ) );
#7010=CARTESIAN_POINT ( 'NONE',  ( 8.731428362939190890, -13.89598863503036164, 3.214285714285716633 ) ) ;
#7011=CARTESIAN_POINT ( 'NONE',  ( 8.512513224245308763, 13.54758718765259040, 1.285714285714285809 ) ) ;
#7013=CARTESIAN_POINT ( 'NONE',  ( 13.55419868402807992, 4.742819248065649695, 43.92857142857143771 ) ) ;
#7015=CARTESIAN_POINT ( 'NONE',  ( 1.478298951650704351, -14.28433602490913579, 37.64689771248358596 ) ) ;
#7017=CARTESIAN_POINT ( 'NONE',  ( 1.737328882695370558, -14.25515036105620581, 41.63881657323070584 ) ) ;
#7020=CARTESIAN_POINT ( 'NONE',  ( 8.841785722321695573, -13.82664651025757152, 23.21024514465928235 ) ) ;
#7021=B_SPLINE_CURVE_WITH_KNOTS ( 'NONE', 3,
 ( #3375, #4925, #6655, #1199, #2845, #9064, #2789, #3679, #1149, #4402, #3617, #4349, #475, #379, #6752, #9940, #4297, #5885, #5937, #5989, #3529, #322, #2075, #5224, #9169, #1972, #6605, #3569, #9838, #6812, #8329, #9989, #8170, #7609, #5125, #8378, #1301, #6039, #5071, #4453, #8222, #4248, #3469, #9793, #8277, #7502, #1923, #2740, #530, #1878, #426, #2895, #6700, #5026, #9117, #2022, #1105, #7399 ),
 .UNSPECIFIED., .F., .F.,
 ( 4, 2, 2, 2, 2, 2, 2, 2, 2, 2, 2, 2, 2, 2, 2, 2, 2, 2, 2, 2, 2, 2, 2, 2, 2, 2, 2, 2, 4 ),
 ( 0.01152039134867053824, 0.01353100581402706323, 0.01554162027938358823, 0.01755223474474011322, 0.01956284921009664168, 0.02157346367545316668, 0.02358407814080969514, 0.02458938537348795417, 0.02559469260616621666, 0.02609734622250534097, 0.02634867303067491007, 0.02647433643475969114, 0.02653716813680208342, 0.02659999983884447222, 0.02666283154088686450, 0.02672566324292925677, 0.02685132664701404132, 0.02710265345518360694, 0.02760530707152273819, 0.02861061430420100068, 0.02961592153687926665, 0.03162653600223580552, 0.03363715046759233745, 0.03464245770027060689, 0.03564776493294886939, 0.03966899386366194713, 0.04067430109634020963, 0.04167960832901848600, 0.04369022279437502487 ),
 .UNSPECIFIED. ) ;
#7022=CARTESIAN_POINT ( 'NONE',  ( 11.60466159355861926, 11.60466159355874716, 1.500000000000003553 ) ) ;
#7024=CARTESIAN_POINT ( 'NONE',  ( -5.404401153735176599, 15.06016580658422477, 20.42453085894499054 ) ) ;
#7030=CARTESIAN_POINT ( 'NONE',  ( -1.665163862719845067, -15.91362231745477374, 47.85310228751642114 ) ) ;
#7034=CARTESIAN_POINT ( 'NONE',  ( -12.22833218042443271, 7.529642458189139909, 31.78167371608784819 ) ) ;
#7038=CARTESIAN_POINT ( 'NONE',  ( -10.24623928997352351, -10.06191849875416899, 8.504040569626438284 ) ) ;
#7039=CARTESIAN_POINT ( 'NONE',  ( -13.91197093850538380, -1.567502665446387278, 47.14285714285714590 ) ) ;
#7041=CARTESIAN_POINT ( 'NONE',  ( 16.32287076676382043, -1.707986654103810897, 10.35310228751642292 ) ) ;
#7044=CARTESIAN_POINT ( 'NONE',  ( -5.420364854931999155, -15.49051278174644253, 40.07142857142857650 ) ) ;
#7050=CARTESIAN_POINT ( 'NONE',  ( 15.06016580658428694, -5.404401153735007846, 30.57546914105500946 ) ) ;
#7053=CARTESIAN_POINT ( 'NONE',  ( 5.543385399275644332, 15.44746603149420494, 29.07546914105501301 ) ) ;
#7054=CARTESIAN_POINT ( 'NONE',  ( -1.791431617652833763, -15.89939535829188877, 21.85714285714286120 ) ) ;
#7055=CARTESIAN_POINT ( 'NONE',  ( 9.147417256656757090, 12.88790924271200566, 48.73000000000002530 ) ) ;
#7056=CARTESIAN_POINT ( 'NONE',  ( 8.731428362939190890, -13.89598863503036164, 9.214285714285717077 ) ) ;
#7059=CARTESIAN_POINT ( 'NONE',  ( -11.31370849898482156, 11.31370849898469544, 5.999999999999998224 ) ) ;
#7060=CARTESIAN_POINT ( 'NONE',  ( 11.31370849898482334, -11.31370849898469366, 9.000000000000001776 ) ) ;
#7061=CARTESIAN_POINT ( 'NONE',  ( 1.607813917173037899, -14.26974319298267169, 45.64285714285715301 ) ) ;
#7062=CARTESIAN_POINT ( 'NONE',  ( 4.865839792409144771, 13.51115193377589740, 35.07546914105501656 ) ) ;
#7066=CARTESIAN_POINT ( 'NONE',  ( 13.21436662431716869, -4.623906867372263640, 2.571428571428571619 ) ) ;
#7070=CARTESIAN_POINT ( 'NONE',  ( 8.404922754268618235, 13.61519076058357491, 27.28167371608785174 ) ) ;
#7071=CARTESIAN_POINT ( 'NONE',  ( 8.512513224245308763, 13.54758718765259040, 1.285714285714285809 ) ) ;
#7072=CARTESIAN_POINT ( 'NONE',  ( 16.32287076676382043, -1.707986654103810897, 22.35310228751642114 ) ) ;
#7077=MANIFOLD_SOLID_BREP ( 'Cavity1', #2342 ) ;
#7078=CARTESIAN_POINT ( 'NONE',  ( -8.512513224245306986, -13.54758718765259218, 34.28571428571428470 ) ) ;
#7081=CARTESIAN_POINT ( 'NONE',  ( -5.420364854931999155, -15.49051278174644253, 10.07142857142856940 ) ) ;
#7083=CARTESIAN_POINT ( 'NONE',  ( -11.78653521626494793, -7.556039541191465148, 24.71024514465928235 ) ) ;
#7087=CARTESIAN_POINT ( 'NONE',  ( -14.25515036105622890, 1.737328882695209575, 3.361183426769288385 ) ) ;
#7089=CARTESIAN_POINT ( 'NONE',  ( 14.25515036105622535, -1.737328882695210241, 18.36118342676929771 ) ) ;
#7090=VERTEX_POINT ( 'NONE', #8829 ) ;
#7091=CARTESIAN_POINT ( 'NONE',  ( 15.44746603149413922, 5.543385399275817527, 3.924530858944990541 ) ) ;
#7093=CARTESIAN_POINT ( 'NONE',  ( -13.89598863503046111, 8.731428362939027465, 47.78571428571430602 ) ) ;
#7099=CARTESIAN_POINT ( 'NONE',  ( -5.164528828830334817, 15.14410076328347543, 22.43261199819786356 ) ) ;
#7101=CARTESIAN_POINT ( 'NONE',  ( -15.53355953199861794, -5.297344310588530725, 38.93261199819787777 ) ) ;
#7107=CARTESIAN_POINT ( 'NONE',  ( 15.89939535829187278, 1.791431617653015174, 20.14285714285714235 ) ) ;
#7110=CARTESIAN_POINT ( 'NONE',  ( 5.420364854932001819, 15.49051278174644430, 1.071428571428570287 ) ) ;
#7112=FILL_AREA_STYLE_COLOUR ( '', #16 ) ;
#7119=CARTESIAN_POINT ( 'NONE',  ( 13.82664651025767100, -8.841785722321541030, 0.7897548553407187644 ) ) ;
#7120=CARTESIAN_POINT ( 'NONE',  ( -16.30827793483735988, 1.837501619626141780, 17.35714285714286476 ) ) ;
#7121=CARTESIAN_POINT ( 'NONE',  ( -9.899494936611716867, 9.899494936611610285, 36.00000000000000711 ) ) ;
#7123=CARTESIAN_POINT ( 'NONE',  ( 1.478298951650704351, -14.28433602490913579, 31.64689771248358241 ) ) ;
#7126=EDGE_LOOP ( 'NONE', ( #3935, #3975, #6373, #6173, #1209, #673 ) ) ;
#7127=CARTESIAN_POINT ( 'NONE',  ( -14.28433602490915000, 1.478298951650542481, 49.35310228751642114 ) ) ;
#7130=CARTESIAN_POINT ( 'NONE',  ( -11.40355824106246807, 11.22385875690704715, 31.99595943037357060 ) ) ;
#7131=CARTESIAN_POINT ( 'NONE',  ( -1.791431617652833763, -15.89939535829188877, 15.85714285714286120 ) ) ;
#7132=CARTESIAN_POINT ( 'NONE',  ( 15.44746603149413922, 5.543385399275817527, 21.92453085894500120 ) ) ;
#7139=CARTESIAN_POINT ( 'NONE',  ( -16.30827793483735988, 1.837501619626141780, 11.35714285714285943 ) ) ;
#7141=CARTESIAN_POINT ( 'NONE',  ( 9.989344678689365153, -9.809645194533958446, 28.99595943037357060 ) ) ;
#7145=CARTESIAN_POINT ( 'NONE',  ( 14.25515036105622535, -1.737328882695210241, 12.36118342676929771 ) ) ;
#7147=CARTESIAN_POINT ( 'NONE',  ( -4.503970704919988854, 13.25633410266674517, 10.43261199819786356 ) ) ;
#7152=CARTESIAN_POINT ( 'NONE',  ( -1.967016585148659846, 16.29368510291087091, 2.638816573230710727 ) ) ;
#7153=CARTESIAN_POINT ( 'NONE',  ( 9.934157114783658926, 9.864832758439671778, 48.73000000000001819 ) ) ;
#7157=CARTESIAN_POINT ( 'NONE',  ( 5.543385399275644332, 15.44746603149420494, 29.07546914105501301 ) ) ;
#7159=CARTESIAN_POINT ( 'NONE',  ( 5.164528828830335705, -15.14410076328347543, 37.43261199819787066 ) ) ;
#7160=VERTEX_POINT ( 'NONE', #7467 ) ;
#7161=CARTESIAN_POINT ( 'NONE',  ( -8.512513224245306986, -13.54758718765259218, 34.28571428571428470 ) ) ;
#7163=CARTESIAN_POINT ( 'NONE',  ( -13.54758718765249625, -8.512513224245459753, 4.714285714285712636 ) ) ;
#7167=CARTESIAN_POINT ( 'NONE',  ( -5.164528828830334817, 15.14410076328347543, -1.567388001802134223 ) ) ;
#7168=CARTESIAN_POINT ( 'NONE',  ( 11.60466159355862104, 11.60466159355875071, 19.50000000000000355 ) ) ;
#7169=CARTESIAN_POINT ( 'NONE',  ( -7.448449071214644945, -11.85413878919601771, 34.28571428571428470 ) ) ;
#7170=CARTESIAN_POINT ( 'NONE',  ( 9.989344678689260348, 9.809645194534072132, 47.50404056962644006 ) ) ;
#7172=CARTESIAN_POINT ( 'NONE',  ( -11.85413878919593422, -7.448449071214776396, 4.714285714285712636 ) ) ;
#7175=ORIENTED_EDGE ( 'NONE', *, *, #4241, .F. ) ;
#7176=CARTESIAN_POINT ( 'NONE',  ( 11.85413878919593422, 7.448449071214774619, 1.714285714285716855 ) ) ;
#7180=CARTESIAN_POINT ( 'NONE',  ( -15.89939535829186923, -1.791431617653016062, 23.14285714285714590 ) ) ;
#7181=CARTESIAN_POINT ( 'NONE',  ( -15.88516839912898071, -1.917699372586004980, 43.13881657323070584 ) ) ;
#7185=CARTESIAN_POINT ( 'NONE',  ( -1.607813917173034124, 14.26974319298267346, 0.6428571428571433488 ) ) ;
#7187=CARTESIAN_POINT ( 'NONE',  ( 14.28433602490915000, -1.478298951650544479, 16.35310228751641759 ) ) ;
#7189=CARTESIAN_POINT ( 'NONE',  ( -1.791431617652833763, -15.89939535829188877, 15.85714285714286120 ) ) ;
#7195=CARTESIAN_POINT ( 'NONE',  ( 11.92174236212692229, 7.340858601238088532, -0.2816737160878517443 ) ) ;
#7196=CARTESIAN_POINT ( 'NONE',  ( 4.865839792409144771, 13.51115193377589740, 17.07546914105500591 ) ) ;
#7199=CARTESIAN_POINT ( 'NONE',  ( 13.54758718765249803, 8.512513224245457977, 43.71428571428572241 ) ) ;
#7205=CARTESIAN_POINT ( 'NONE',  ( 11.69682198916835070, 11.51250119794901394, 29.50404056962643295 ) ) ;
#7207=CARTESIAN_POINT ( 'NONE',  ( -13.82664651025767100, 8.841785722321537477, 27.78975485534072121 ) ) ;
#7210=CARTESIAN_POINT ( 'NONE',  ( -13.54758718765249625, -8.512513224245459753, 28.71428571428571530 ) ) ;
#7211=CARTESIAN_POINT ( 'NONE',  ( 3.824282371705687744, 14.64065971923091602, 7.152024097632292178E-17 ) ) ;
#7217=CARTESIAN_POINT ( 'NONE',  ( -13.59724543428031573, -4.619798703722008959, 44.93261199819787777 ) ) ;
#7218=CARTESIAN_POINT ( 'NONE',  ( -15.89939535829186923, -1.791431617653016062, 17.14285714285713880 ) ) ;
#7219=CARTESIAN_POINT ( 'NONE',  ( 7.448449071214646722, 11.85413878919601594, 43.28571428571429180 ) ) ;
#7220=CARTESIAN_POINT ( 'NONE',  ( -12.08964793087886314, 7.750357176954159932, 39.78975485534073186 ) ) ;
#7222=CARTESIAN_POINT ( 'NONE',  ( -13.91197093850538380, -1.567502665446387278, 5.142857142857143238 ) ) ;
#7226=CARTESIAN_POINT ( 'NONE',  ( -13.89774397934249706, -1.693770420379375974, 49.13881657323070584 ) ) ;
#7228=CARTESIAN_POINT ( 'NONE',  ( 5.420364854932000931, 15.49051278174644075, 19.07142857142856940 ) ) ;
#7229=CARTESIAN_POINT ( 'NONE',  ( -13.96533075980324234, 8.621071003556515677, 31.78167371608784819 ) ) ;
#7232=CARTESIAN_POINT ( 'NONE',  ( 1.567502665446232957, 13.91197093850540156, 0.8571428571428549859 ) ) ;
#7236=CARTESIAN_POINT ( 'NONE',  ( 7.340858601237956194, 11.92174236212700045, 15.28167371608785174 ) ) ;
#7239=CARTESIAN_POINT ( 'NONE',  ( 15.49051278174638036, 5.420364854932175014, 37.92857142857143060 ) ) ;
#7240=CARTESIAN_POINT ( 'NONE',  ( 1.441234910513245149, 13.92619789766829008, 44.85310228751641404 ) ) ;
#7244=CARTESIAN_POINT ( 'NONE',  ( 7.556039541191335474, 11.78653521626503320, 23.28975485534072121 ) ) ;
#7245=CARTESIAN_POINT ( 'NONE',  ( -10.24623928997352351, -10.06191849875416899, 8.504040569626438284 ) ) ;
#7247=CARTESIAN_POINT ( 'NONE',  ( -16.32287076676382398, 1.707986654103809343, 13.35310228751641937 ) ) ;
#7254=CARTESIAN_POINT ( 'NONE',  ( 1.917699372585825790, 15.88516839912900203, 28.86118342676929416 ) ) ;
#7256=CARTESIAN_POINT ( 'NONE',  ( -5.543385399275643444, -15.44746603149420494, 32.07546914105502367 ) ) ;
#7259=CARTESIAN_POINT ( 'NONE',  ( 15.49051278174638036, 5.420364854932175014, 37.92857142857143060 ) ) ;
#7261=CARTESIAN_POINT ( 'NONE',  ( 15.10213328493390783, -5.284464991282587398, 20.57142857142857295 ) ) ;
#7265=CARTESIAN_POINT ( 'NONE',  ( -12.08964793087886314, 7.750357176954159932, 39.78975485534073186 ) ) ;
#7267=CARTESIAN_POINT ( 'NONE',  ( 15.10213328493390783, -5.284464991282587398, 14.57142857142856940 ) ) ;
#7270=CARTESIAN_POINT ( 'NONE',  ( 8.620103694221997515, 13.47998361472160767, -0.7102451446592792372 ) ) ;
#7271=ADVANCED_FACE ( 'NONE', ( #2659 ), #3389, .T. ) ;
#7272=CARTESIAN_POINT ( 'NONE',  ( 9.899494936611718643, -9.899494936611608509, 9.000000000000001776 ) ) ;
#7276=CARTESIAN_POINT ( 'NONE',  ( -14.26974319298268767, 1.607813917172874918, 5.357142857142856762 ) ) ;
#7283=CARTESIAN_POINT ( 'NONE',  ( 1.791431617652837316, 15.89939535829188877, 12.85714285714285943 ) ) ;
#7284=CARTESIAN_POINT ( 'NONE',  ( -1.967016585148659846, 16.29368510291087091, 38.63881657323070584 ) ) ;
#7289=CARTESIAN_POINT ( 'NONE',  ( -1.737328882695368115, 14.25515036105620581, 14.63881657323070939 ) ) ;
#7292=CARTESIAN_POINT ( 'NONE',  ( 9.989344678689365153, -9.809645194533958446, 34.99595943037355994 ) ) ;
#7296=CARTESIAN_POINT ( 'NONE',  ( -11.92174236212692051, -7.340858601238089420, 14.71832628391215003 ) ) ;
#7298=CARTESIAN_POINT ( 'NONE',  ( -13.59724543428031573, -4.619798703722008959, 14.93261199819787066 ) ) ;
#7301=CARTESIAN_POINT ( 'NONE',  ( 11.51250119794888249, 11.69682198916847682, 3.495959430373559940 ) ) ;
#7307=B_SPLINE_CURVE_WITH_KNOTS ( 'NONE', 3,
 ( #3455, #3666, #2779, #6739, #9931, #9782, #1140, #2835, #4286, #5875, #2683, #5827, #9003, #5927 ),
 .UNSPECIFIED., .F., .F.,
 ( 4, 2, 2, 2, 2, 2, 4 ),
 ( 0.000000000000000000, 0.001440048918583816629, 0.002880097837167633259, 0.005760195674335269987, 0.007200244592919087701, 0.008640293511502904547, 0.01152039134867053824 ),
 .UNSPECIFIED. ) ;
#7308=CARTESIAN_POINT ( 'NONE',  ( 14.26974319298268767, -1.607813917172876916, 26.35714285714285765 ) ) ;
#7309=CARTESIAN_POINT ( 'NONE',  ( 1.917699372585825790, 15.88516839912900203, 40.86118342676929416 ) ) ;
#7311=CARTESIAN_POINT ( 'NONE',  ( 5.284464991282756152, -15.10213328493384743, 33.42857142857143060 ) ) ;
#7312=CARTESIAN_POINT ( 'NONE',  ( -6.139641135253190107, 12.65605934851316228, 2.357314452189447182E-16 ) ) ;
#7314=CARTESIAN_POINT ( 'NONE',  ( 1.837501619626330074, -16.30827793483733501, 15.64285714285714235 ) ) ;
#7320=CARTESIAN_POINT ( 'NONE',  ( 9.989344678689260348, 9.809645194534072132, 47.50404056962644006 ) ) ;
#7321=CARTESIAN_POINT ( 'NONE',  ( 16.30827793483735633, -1.837501619626142890, 32.35714285714286120 ) ) ;
#7322=CARTESIAN_POINT ( 'NONE',  ( -10.15407889436378852, -10.15407889436390398, 46.50000000000001421 ) ) ;
#7323=CARTESIAN_POINT ( 'NONE',  ( 13.92619789766827587, 1.441234910513398582, 36.14689771248357886 ) ) ;
#7324=CARTESIAN_POINT ( 'NONE',  ( -7.448449071214644945, -11.85413878919601771, 16.28571428571428470 ) ) ;
#7328=CARTESIAN_POINT ( 'NONE',  ( -4.742819248065502258, -13.55419868402813677, 22.07142857142858006 ) ) ;
#7332=CARTESIAN_POINT ( 'NONE',  ( -8.731428362939187338, 13.89598863503036164, 12.21428571428571708 ) ) ;
#7333=CARTESIAN_POINT ( 'NONE',  ( -5.297344310588352201, -15.53355953199867301, 42.06738800180214355 ) ) ;
#7336=CARTESIAN_POINT ( 'NONE',  ( 4.623906867372411078, -13.21436662431711717, 9.428571428571425272 ) ) ;
#7338=CARTESIAN_POINT ( 'NONE',  ( 7.750357176954296712, -12.08964793087877787, 23.21024514465928235 ) ) ;
#7342=CARTESIAN_POINT ( 'NONE',  ( -13.89774397934249706, -1.693770420379375974, 37.13881657323070584 ) ) ;
#7346=CARTESIAN_POINT ( 'NONE',  ( 13.17239914596754424, -4.743843029824685864, 18.57546914105500235 ) ) ;
#7348=CARTESIAN_POINT ( 'NONE',  ( 4.865839792409144771, 13.51115193377589740, 23.07546914105501301 ) ) ;
#7351=CARTESIAN_POINT ( 'NONE',  ( -11.31370849898482156, 11.31370849898469544, 18.00000000000000355 ) ) ;
#7352=CARTESIAN_POINT ( 'NONE',  ( 15.44746603149413922, 5.543385399275817527, 15.92453085894499409 ) ) ;
#7358=CARTESIAN_POINT ( 'NONE',  ( 5.543385399275644332, 15.44746603149420494, 35.07546914105501656 ) ) ;
#7359=CARTESIAN_POINT ( 'NONE',  ( 1.607813917173038121, -14.26974319298267346, 27.64285714285714590 ) ) ;
#7360=CARTESIAN_POINT ( 'NONE',  ( 13.91197093850538380, 1.567502665446386390, 32.14285714285714590 ) ) ;
#7362=CARTESIAN_POINT ( 'NONE',  ( 11.31370849898482334, -11.31370849898469366, 27.00000000000000355 ) ) ;
#7364=CARTESIAN_POINT ( 'NONE',  ( 13.54758718765249803, 8.512513224245457977, 13.71428571428571352 ) ) ;
#7365=DIRECTION ( 'NONE',  ( 0.9983709538884036894, -0.05705644952114250629, 5.938629746412706501E-18 ) ) ;
#7368=CARTESIAN_POINT ( 'NONE',  ( -8.620103694221995738, -13.47998361472161299, 14.28975485534072298 ) ) ;
#7369=CARTESIAN_POINT ( 'NONE',  ( 5.420364854932001819, 15.49051278174644430, 25.07142857142858361 ) ) ;
#7370=CARTESIAN_POINT ( 'NONE',  ( -2.525158672622311418, 13.94875038000408374, 48.57768213684325787 ) ) ;
#7371=CARTESIAN_POINT ( 'NONE',  ( -5.543385399275643444, -15.44746603149420494, 2.075469141055009015 ) ) ;
#7372=CARTESIAN_POINT ( 'NONE',  ( 13.21436662431716869, -4.623906867372263640, 8.571428571428569398 ) ) ;
#7376=CARTESIAN_POINT ( 'NONE',  ( -1.607813917173034124, 14.26974319298267524, 18.64285714285715656 ) ) ;
#7379=CARTESIAN_POINT ( 'NONE',  ( -13.89598863503045933, 8.731428362939027465, 29.78571428571428825 ) ) ;
#7380=CARTESIAN_POINT ( 'NONE',  ( 11.51250119794888249, 11.69682198916847682, 39.49595943037357415 ) ) ;
#7382=CARTESIAN_POINT ( 'NONE',  ( 4.623906867372411078, -13.21436662431711717, 15.42857142857143060 ) ) ;
#7383=CARTESIAN_POINT ( 'NONE',  ( -4.619798703721853528, -13.59724543428036725, 30.06738800180214355 ) ) ;
#7385=( BOUNDED_SURFACE ( )  B_SPLINE_SURFACE ( 3, 2, ( 
 ( #3594, #2870, #2764, #6013, #8400, #6675, #8305, #8353, #9192, #5913, #1176, #1325, #5155, #9859, #7578, #10009, #2050, #7528, #5203, #4273, #8459, #2919, #4481, #1227, #1271, #7636, #6064, #555, #6631, #4377, #4430, #5965, #453, #9238, #2156, #6726, #9914, #7424, #3704, #352, #7476, #5302, #3500, #9143, #2820, #501, #9815, #2716, #3648, #5860, #6785, #1948, #9963, #5097, #8247, #4325, #10215, #2971, #8616, #30, #6268, #4686, #7741, #610, #3961, #9345, #5555, #4537, #7883, #2255, #6220, #9296, #7691, #2309, #660, #1384, #5455, #8666, #1588, #8560, #5508, #4735, #2210, #6319, #6121, #9452, #5356, #7002, #2357, #809, #7833, #1539, #5403, #1485, #7107, #10114, #6948, #3908, #3184, #9501, #8510, #2407, #7054, #3757, #6890, #713, #10059, #3028, #3811, #4636, #7794, #3862, #10162, #3076, #9397, #5602, #235, #3280, #914, #1785, #4210, #6474, #1738, #9654, #8714, #2656, #7362, #2606, #5657, #2559, #9698, #287, #6519, #864, #7210, #5703, #184, #9604, #3430, #6567, #7987, #2508, #1636, #5750, #4783, #1693, #1835, #8918, #3338, #8825, #4063, #3386, #7935, #4888, #9750, #128, #7311, #8871, #4937, #4014, #7161, #4990, #79, #8084, #3232, #8134, #1015, #4834, #6371, #9549, #6423, #2456, #8767, #8036, #963, #4165, #4113, #7259, #6713, #5848, #9998, #9897, #2855, #6000, #2752, #9951, #9179, #3487, #541, #337, #3631, #6617, #1210, #6766, #2085, #9130, #5951, #6665, #389, #5233, #4313, #1161, #2032, #7564, #8388, #9802, #1310, #2803, #4463, #7620, #8289, #3690, #3581, #6824, #9025, #7410, #5802, #7463, #4361, #8979, #7514, #1890, #5190, #439, #3539, #5141, #5038, #5897, #8338, #8184, #5083, #1256, #1117 ),
 ( #4415, #486, #4261, #2706, #1936, #8234, #9848, #751, #7729, #7091, #3013, #5441, #2906, #6256, #3741, #1369, #10201, #9283, #6157, #4724, #2140, #6876, #6105, #9224, #5284, #8444, #7870, #5345, #796, #2346, #595, #8498, #2958, #9436, #3898, #9333, #4521, #5496, #8655, #7041, #5389, #7679, #4622, #10046, #8549, #2297, #2197, #1424, #3946, #6931, #4674, #648, #3797, #10103, #1474, #7780, #703, #3850, #6988, #10151, #3064, #6208, #9383, #8601, #7824, #15, #2394, #3171, #6308, #9489, #5543, #3928, #1503, #3148, #5423, #827, #3206, #9520, #7757, #7902, #778, #630, #9364, #48, #7809, #6139, #7024, #3983, #3831, #5477, #4758, #8638, #733, #7132, #9416, #7072, #5526, #8530, #4656, #10182, #6288, #1607, #1456, #3047, #9315, #6340, #5739, #682, #3881, #2426, #5572, #2375, #8735, #10080, #8685, #8580, #6910, #4606, #6969, #4558, #7709, #3778, #3098, #2996, #2229, #5374, #10131, #6189, #2276, #6238, #2328, #1559, #4705, #7854, #9474, #2528, #6445, #5769, #149, #7229, #1803, #3404, #8944, #2472, #1857, #8891, #4229, #306, #4132, #2623, #9671, #5007, #4857, #3251, #8154, #3304, #208, #9772, #3358, #3447, #1039, #6493, #9625, #983, #1088, #8846, #2580, #6589, #934, #4183, #6540, #7284, #256, #5677, #9719, #7380, #4079, #1756, #5722, #2675, #4907, #8792, #5821, #8053, #4958, #8110, #1655, #7333, #4805, #7956, #886, #4036, #7181, #97, #6391, #9569, #5626, #1711, #8004, #1134, #7482, #6732, #461, #9866, #3710, #562, #8255, #2771, #1907, #6792, #5056, #1954, #2108, #9969, #3600, #5918, #1182, #3655, #2927, #9094, #6844, #410, #7584, #9923, #9149, #8202, #8998, #509, #360, #5971, #7642, #2877, #2056 ),
 ( #6682, #2826, #6637, #4279, #5209, #9044, #7431, #8359, #5161, #4331, #8312, #9821, #3507, #2723, #1232, #6019, #4383, #5251, #7534, #1280, #4438, #9198, #8407, #3554, #5866, #2007, #1334, #5103, #4488, #10015, #6070, #1391, #2165, #5309, #9245, #8466, #9889, #9122, #1975, #5888, #5133, #4567, #8331, #641, #5336, #3571, #1249, #5942, #2950, #6868, #5993, #4353, #6094, #9275, #10038, #9172, #430, #7612, #2792, #2078, #5274, #5182, #8280, #1417, #9943, #4514, #2189, #8491, #3790, #4455, #2024, #3620, #1202, #7505, #6705, #2848, #1303, #4406, #6757, #5226, #9067, #3682, #7555, #7671, #478, #587, #8437, #8380, #3732, #533, #7721, #6920, #10095, #6817, #9991, #2132, #2897, #6041, #9217, #1361, #4614, #8647, #1667, #2289, #3939, #3215, #7083, #9426, #9530, #5, #5536, #3996, #10142, #10194, #1570, #4765, #59, #3056, #1518, #7769, #4816, #8695, #5432, #2337, #7966, #896, #7141, #6150, #1465, #9326, #3890, #5382, #6200, #4665, #2236, #696, #7816, #3843, #3162, #7034, #4716, #6300, #1617, #4237, #8013, #5063, #4868, #8161, #945, #5732, #1096, #7388, #3412, #265, #7292, #4919, #315, #8854, #5684, #6548, #1867, #3456, #4091, #6598, #7342, #2685, #9004, #2587, #9783, #8119, #5828, #3315, #1722, #1915, #1764, #8899, #8211, #1813, #1141, #9731, #4970, #8064, #9680, #107, #215, #1049, #3260, #9634, #2632, #5015, #4193, #8954, #3366, #6402, #9578, #2538, #6500, #5780, #2483, #5637, #7240, #8804, #158, #6455, #522, #10030, #1290, #6741, #4446, #7442, #1405, #6083, #1349, #4394, #7597, #4504, #2940, #7658, #9831, #5929, #3670, #9160, #8322, #2182, #9260, #9877, #1240, #368, #576, #3518, #419, #3721, #5325 ),
 ( #9107, #2121, #6804, #9981, #6646, #2731, #8481, #9055, #5877, #5113, #8267, #1190, #3562, #4340, #7493, #5172, #9934, #2837, #5981, #2067, #8882, #1702, #7172, #8100, #7222, #89, #4028, #3244, #2668, #6434, #8989, #3440, #4847, #9617, #4073, #1081, #5000, #4123, #5616, #4223, #7372, #8146, #7272, #8784, #5712, #7997, #198, #3396, #3293, #6382, #9764, #8046, #2616, #299, #6580, #1900, #2571, #140, #1749, #9561, #925, #2519, #975, #9663, #5668, #4898, #3350, #8836, #1796, #6485, #5761, #1029, #8933, #6531, #4175, #1850, #7324, #5813, #5049, #8194, #247, #9710, #7577, #7422, #5912, #6835, #4376, #2715, #3593, #554, #404, #2049, #1324, #8352, #7527, #4480, #5964, #3647, #2099, #5096, #8304, #6725, #2868, #8399, #8246, #9858, #5859, #10008, #500, #7475, #1226, #7635, #3703, #9191, #2155, #6630, #5244, #2000, #3499, #1174, #3547, #2918, #351, #452, #6674, #9913, #1947, #9814, #9036, #2819, #6012, #1270, #6063, #4429, #6783, #9237, #5301, #1126, #9086, #4272, #4324, #2763, #5153, #608, #8458, #1383, #4536, #3756, #7690, #6764, #7360, #1887, #6710, #9747, #5139, #9949, #2799, #1208, #4258, #284, #484, #5846, #2083, #1066, #4413, #1934, #2750, #8977, #4208, #9072, #8182, #8132, #1981, #5188, #8336, #5080, #2030, #1254, #5036, #2853, #1115, #5949, #7408, #3537, #9128, #7561, #4359, #8287, #8232, #2704, #3627, #6615, #3484, #7512, #9895, #5998, #334, #9177, #437, #3428, #1158, #387, #4311, #5894, #7461, #6663, #9846, #3579, #593, #3795, #3114, #6928, #3896, #4620, #10101, #10044, #4572, #6206, #2195, #6155, #7039, #4519, #7777, #6986, #7727, #3848, #3739, #10149, #3062, #7677, #9281, #9331, #9381 ),
 ( #9996, #3011, #9222, #8496, #701, #6874, #1308, #749, #5343, #2295, #5438, #8599, #6254, #2242, #1367, #2956, #7618, #3688, #2904, #1422, #646, #5281, #6102, #5387, #8386, #8547, #539, #1524, #6822, #4672, #7822, #1471, #10199, #9433, #5231, #4460, #6048, #8442, #2138, #8812, #9535, #3267, #4149, #4770, #4874, #4099, #1675, #950, #846, #7245, #165, #7917, #6357, #6408, #3325, #4001, #2392, #6461, #7147, #64, #5643, #4924, #114, #5588, #9585, #2343, #6506, #998, #9640, #2442, #2492, #2546, #8071, #5690, #4722, #3220, #1728, #4049, #8750, #7298, #220, #4821, #7972, #5495, #1771, #8653, #5541, #3373, #1575, #7196, #901, #8019, #7868, #794, #3944, #7089, #12, #3168, #6306, #8701, #8905, #2593, #8274, #1056, #6651, #8472, #4345, #2737, #8962, #1819, #2173, #7396, #3770, #4976, #6075, #3465, #4294, #7348, #4198, #375, #9736, #271, #3526, #6850, #10021, #2692, #2933, #9251, #3417, #622, #6553, #7499, #5022, #5068, #5315, #8166, #9061, #1969, #5834, #4244, #1102, #9011, #1920, #5121, #1195, #8219, #671, #818, #3917, #9512, #5566, #9406, #7893, #4697, #39, #10122, #1447, #7123, #2266, #5468, #4795, #1550, #8727, #9464, #7844, #7802, #770, #3197, #6903, #876, #1648, #6332, #3872, #7062, #2418, #7948, #4748, #9307, #5413, #10225, #3135, #724, #10070, #2220, #6179, #7015, #5366, #6960, #3039, #9356, #10172, #3087, #2366, #5518, #1599, #7265, #6526, #6378, #4171, #871, #971, #3288, #2515, #1594, #2362, #4120, #3968, #9613, #1023, #194, #5664, #8722, #4744, #4944, #85, #5515, #8675, #8879, #3240, #7217, #35, #7890, #6429, #2415, #815, #8832, #9659, #2567, #9557, #6480, #5708, #3192, #7320 ),
 ( #1744, #2462, #7167, #1792, #4023, #7943, #4894, #3346, #8092, #6328, #243, #8042, #3392, #7119, #4843, #9509, #136, #5561, #1644, #4788, #5610, #8780, #921, #1698, #4069, #7993, #9081, #1168, #4268, #9031, #447, #6624, #399, #1266, #8985, #1992, #1221, #1942, #8299, #8190, #4372, #7524, #1896, #3495, #3544, #3589, #7417, #6575, #6722, #344, #5045, #2758, #2043, #7470, #2711, #6671, #9907, #9854, #5906, #8925, #9705, #2814, #1077, #5149, #8349, #5960, #9139, #5809, #1845, #5199, #9810, #3641, #2612, #4425, #5855, #4321, #7368, #5757, #7574, #9757, #4996, #496, #8142, #4217, #5092, #294, #3437, #2664, #8241, #551, #7790, #3698, #4582, #10159, #2305, #3024, #6942, #3750, #1380, #8612, #5296, #2149, #5399, #1536, #759, #6832, #6779, #2864, #9188, #2914, #9293, #9233, #10056, #6115, #7099, #5505, #4109, #9497, #2451, #1780, #5597, #2555, #3276, #8760, #8710, #6366, #4884, #858, #4830, #5699, #2403, #6417, #5652, #9544, #2503, #5551, #8821, #8029, #1632, #7929, #7983, #959, #4010, #3954, #7254, #7157, #1688, #7205, #4933, #910, #4059, #124, #7050, #10211, #3123, #176, #9596, #3334, #6263, #9448, #2354, #8663, #1585, #4732, #7879, #5034, #5946, #2797, #281, #8179, #4158, #8284, #229, #7358, #4357, #7510, #5844, #7406, #3426, #435, #1009, #332, #9126, #2651, #3480, #9844, #6612, #3575, #9022, #8230, #7458, #2028, #3382, #8975, #6515, #2602, #4985, #7559, #1469, #537, #6761, #4618, #3686, #7675, #6984, #482, #2901, #6046, #2136, #591, #3736, #10147, #6872, #3060, #7775, #10042, #2954, #6100, #6204, #2240, #9279, #2193, #9379, #2293, #5340, #6926, #10099, #4669, #8597, #1522, #7820, #747, #5436 ),
 ( #1393, #2983, #7644, #6846, #2929, #2217, #668, #8468, #5363, #8519, #8409, #3035, #564, #3867, #6072, #7010, #721, #1443, #10168, #3821, #1546, #3913, #10221, #4546, #8625, #5464, #1336, #6956, #7059, #9352, #9247, #2262, #7840, #7699, #5410, #6277, #8568, #9460, #5253, #4490, #2167, #618, #3765, #6899, #5580, #4865, #9632, #7081, #1615, #4714, #4915, #6400, #6298, #7139, #8062, #990, #4088, #10192, #5488, #3107, #56, #1568, #2, #9482, #6247, #787, #6350, #2385, #9528, #3159, #7910, #8743, #7964, #4043, #7189, #2481, #5635, #9728, #3364, #9678, #4191, #6546, #5838, #8278, #7351, #5938, #1879, #5027, #2790, #8172, #9015, #4403, #1106, #4249, #323, #2696, #1924, #5072, #476, #8223, #3618, #6753, #1150, #4298, #7453, #9118, #6701, #3530, #9839, #5886, #9065, #9887, #1973, #5126, #1200, #4350, #7503, #427, #2130, #9170, #8590, #6865, #7767, #6979, #10140, #742, #1415, #5272, #584, #3680, #6813, #8432, #9271, #8489, #7668, #3730, #4565, #5990, #638, #7718, #693, #6918, #3841, #8539, #3004, #3054, #6147, #2285, #1515, #2076, #6198, #5430, #6346, #5483, #5530, #1564, #9524, #1612, #783, #3934, #7078, #7877, #2401, #804, #1583, #1533, #3179, #10209, #3121, #25, #4918, #8803, #1721, #4867, #6454, #944, #4090, #7239, #4949, #8099, #8932, #8876, #241, #8139, #2002, #454, #1228, #2102, #9193, #9915, #3595, #2920, #7529, #4378, #5246, #556, #6065, #9860, #9239, #6014, #5156, #6727, #2821, #8401, #1326, #5966, #9144, #2157, #2051, #5204, #4482, #3705, #5303, #2765, #8460, #7637, #1385, #7692, #1272, #10010, #6786, #4538, #8306, #406, #611, #8354, #7579, #6891, #502, #3758, #6838, #3649, #4431 ) ),
 .UNSPECIFIED., .T., .F., .F. ) 
 B_SPLINE_SURFACE_WITH_KNOTS ( ( 4, 3, 4 ),
 ( 3, 2, 2, 2, 2, 2, 2, 2, 2, 2, 2, 2, 2, 2, 2, 2, 2, 2, 2, 2, 2, 2, 2, 2, 2, 2, 2, 2, 2, 2, 2, 2, 2, 2, 2, 2, 2, 2, 2, 2, 2, 2, 2, 2, 2, 2, 2, 2, 2, 2, 2, 2, 2, 2, 2, 2, 2, 2, 2, 2, 2, 2, 2, 2, 2, 2, 2, 2, 2, 2, 2, 2, 2, 2, 2, 2, 2, 2, 2, 2, 2, 2, 2, 2, 2, 2, 2, 2, 2, 2, 2, 2, 2, 2, 2, 2, 2, 2, 2, 2, 2, 2, 2, 2, 2, 2, 2, 2, 2, 2, 2, 2, 2, 2, 2, 2, 3 ),
 ( 0.000000000000000000, 0.5000000000000000000, 1.000000000000000000 ),
 ( 0.000000000000000000, 0.007936507936507936067, 0.01587301587301587213, 0.02380952380952380820, 0.03174603174603174427, 0.03968253968253968034, 0.04761904761904761640, 0.05555555555555555247, 0.06349206349206348854, 0.07142857142857142461, 0.07936507936507936067, 0.08730158730158729674, 0.09523809523809523281, 0.1031746031746031689, 0.1111111111111111049, 0.1190476190476190410, 0.1269841269841269771, 0.1349206349206349131, 0.1428571428571428492, 0.1507936507936507853, 0.1587301587301587213, 0.1666666666666666574, 0.1746031746031745935, 0.1825396825396825295, 0.1904761904761904656, 0.1984126984126984017, 0.2063492063492063378, 0.2142857142857142738, 0.2222222222222222099, 0.2301587301587301460, 0.2380952380952380820, 0.2460317460317460181, 0.2539682539682539542, 0.2619047619047619180, 0.2698412698412698263, 0.2777777777777777901, 0.2857142857142856984, 0.2936507936507936622, 0.3015873015873015706, 0.3095238095238095344, 0.3174603174603174427, 0.3253968253968254065, 0.3333333333333333148, 0.3412698412698412787, 0.3492063492063491870, 0.3571428571428571508, 0.3650793650793650591, 0.3730158730158730229, 0.3809523809523809312, 0.3888888888888888951, 0.3968253968253968034, 0.4047619047619047672, 0.4126984126984126755, 0.4206349206349206393, 0.4285714285714285476, 0.4365079365079365115, 0.4444444444444444198, 0.4523809523809523836, 0.4603174603174602919, 0.4682539682539682557, 0.4761904761904761640, 0.4841269841269841279, 0.4920634920634920362, 0.5000000000000000000, 0.5079365079365079083, 0.5158730158730159276, 0.5238095238095238360, 0.5317460317460317443, 0.5396825396825396526, 0.5476190476190476719, 0.5555555555555555802, 0.5634920634920634885, 0.5714285714285713969, 0.5793650793650794162, 0.5873015873015873245, 0.5952380952380952328, 0.6031746031746031411, 0.6111111111111111605, 0.6190476190476190688, 0.6269841269841269771, 0.6349206349206348854, 0.6428571428571429047, 0.6507936507936508130, 0.6587301587301587213, 0.6666666666666666297, 0.6746031746031746490, 0.6825396825396825573, 0.6904761904761904656, 0.6984126984126983739, 0.7063492063492063933, 0.7142857142857143016, 0.7222222222222222099, 0.7301587301587301182, 0.7380952380952381375, 0.7460317460317460458, 0.7539682539682539542, 0.7619047619047618625, 0.7698412698412698818, 0.7777777777777777901, 0.7857142857142856984, 0.7936507936507936067, 0.8015873015873016261, 0.8095238095238095344, 0.8174603174603174427, 0.8253968253968253510, 0.8333333333333333703, 0.8412698412698412787, 0.8492063492063491870, 0.8571428571428570953, 0.8650793650793651146, 0.8730158730158730229, 0.8809523809523809312, 0.8888888888888888395, 0.8968253968253968589, 0.9047619047619047672, 0.9126984126984126755, 0.9166666666666666297 ),
 .UNSPECIFIED. ) 
 GEOMETRIC_REPRESENTATION_ITEM ( )  RATIONAL_B_SPLINE_SURFACE ( (
 ( 1.000000000000000000, 0.9749279121818236193, 1.000000000000000000, 0.9749279121818236193, 1.000000000000000000, 0.9749279121818236193, 1.000000000000000000, 0.9749279121818236193, 1.000000000000000000, 0.9749279121818236193, 1.000000000000000000, 0.9749279121818236193, 1.000000000000000000, 0.9749279121818236193, 1.000000000000000000, 0.9749279121818236193, 1.000000000000000000, 0.9749279121818236193, 1.000000000000000000, 0.9749279121818236193, 1.000000000000000000, 0.9749279121818236193, 1.000000000000000000, 0.9749279121818236193, 1.000000000000000000, 0.9749279121818236193, 1.000000000000000000, 0.9749279121818236193, 1.000000000000000000, 0.9749279121818236193, 1.000000000000000000, 0.9749279121818236193, 1.000000000000000000, 0.9749279121818236193, 1.000000000000000000, 0.9749279121818236193, 1.000000000000000000, 0.9749279121818236193, 1.000000000000000000, 0.9749279121818236193, 1.000000000000000000, 0.9749279121818236193, 1.000000000000000000, 0.9749279121818236193, 1.000000000000000000, 0.9749279121818236193, 1.000000000000000000, 0.9749279121818236193, 1.000000000000000000, 0.9749279121818236193, 1.000000000000000000, 0.9749279121818236193, 1.000000000000000000, 0.9749279121818236193, 1.000000000000000000, 0.9749279121818236193, 1.000000000000000000, 0.9749279121818236193, 1.000000000000000000, 0.9749279121818236193, 1.000000000000000000, 0.9749279121818236193, 1.000000000000000000, 0.9749279121818236193, 1.000000000000000000, 0.9749279121818236193, 1.000000000000000000, 0.9749279121818236193, 1.000000000000000000, 0.9749279121818236193, 1.000000000000000000, 0.9749279121818236193, 1.000000000000000000, 0.9749279121818236193, 1.000000000000000000, 0.9749279121818236193, 1.000000000000000000, 0.9749279121818236193, 1.000000000000000000, 0.9749279121818236193, 1.000000000000000000, 0.9749279121818236193, 1.000000000000000000, 0.9749279121818236193, 1.000000000000000000, 0.9749279121818236193, 1.000000000000000000, 0.9749279121818236193, 1.000000000000000000, 0.9749279121818236193, 1.000000000000000000, 0.9749279121818236193, 1.000000000000000000, 0.9749279121818236193, 1.000000000000000000, 0.9749279121818236193, 1.000000000000000000, 0.9749279121818236193, 1.000000000000000000, 0.9749279121818236193, 1.000000000000000000, 0.9749279121818236193, 1.000000000000000000, 0.9749279121818236193, 1.000000000000000000, 0.9749279121818236193, 1.000000000000000000, 0.9749279121818236193, 1.000000000000000000, 0.9749279121818236193, 1.000000000000000000, 0.9749279121818236193, 1.000000000000000000, 0.9749279121818236193, 1.000000000000000000, 0.9749279121818236193, 1.000000000000000000, 0.9749279121818236193, 1.000000000000000000, 0.9749279121818236193, 1.000000000000000000, 0.9749279121818236193, 1.000000000000000000, 0.9749279121818236193, 1.000000000000000000, 0.9749279121818236193, 1.000000000000000000, 0.9749279121818236193, 1.000000000000000000, 0.9749279121818236193, 1.000000000000000000, 0.9749279121818236193, 1.000000000000000000, 0.9749279121818236193, 1.000000000000000000, 0.9749279121818236193, 1.000000000000000000, 0.9749279121818236193, 1.000000000000000000, 0.9749279121818236193, 1.000000000000000000, 0.9749279121818236193, 1.000000000000000000, 0.9749279121818236193, 1.000000000000000000, 0.9749279121818236193, 1.000000000000000000, 0.9749279121818236193, 1.000000000000000000, 0.9749279121818236193, 1.000000000000000000, 0.9749279121818236193, 1.000000000000000000, 0.9749279121818236193, 1.000000000000000000, 0.9749279121818236193, 1.000000000000000000, 0.9749279121818236193, 1.000000000000000000, 0.9749279121818236193, 1.000000000000000000, 0.9749279121818236193, 1.000000000000000000, 0.9749279121818236193, 1.000000000000000000, 0.9749279121818236193, 1.000000000000000000, 0.9749279121818236193, 1.000000000000000000, 0.9749279121818236193, 1.000000000000000000, 0.9749279121818236193, 1.000000000000000000, 0.9749279121818236193, 1.000000000000000000, 0.9749279121818236193, 1.000000000000000000, 0.9749279121818236193, 1.000000000000000000, 0.9749279121818236193, 1.000000000000000000, 0.9749279121818236193, 1.000000000000000000, 0.9749279121818236193, 1.000000000000000000, 0.9749279121818236193, 1.000000000000000000, 0.9749279121818236193, 1.000000000000000000, 0.9749279121818236193, 1.000000000000000000, 0.9749279121818236193, 1.000000000000000000, 0.9749279121818236193, 1.000000000000000000, 0.9749279121818236193, 1.000000000000000000, 0.9749279121818236193, 1.000000000000000000, 0.9749279121818236193, 1.000000000000000000, 0.9749279121818236193, 1.000000000000000000, 0.9749279121818236193, 1.000000000000000000, 0.9749279121818236193, 1.000000000000000000, 0.9749279121818236193, 1.000000000000000000, 0.9749279121818236193, 1.000000000000000000, 0.9749279121818236193, 1.000000000000000000, 0.9749279121818236193, 1.000000000000000000, 0.9749279121818236193, 1.000000000000000000, 0.9749279121818236193, 1.000000000000000000, 0.9749279121818236193, 1.000000000000000000, 0.9749279121818236193, 1.000000000000000000, 0.9749279121818236193, 1.000000000000000000, 0.9749279121818236193, 1.000000000000000000, 0.9749279121818236193, 1.000000000000000000, 0.9749279121818236193, 1.000000000000000000, 0.9874639560909117542, 0.9874639560909117542),
 ( 0.3333333333333333703, 0.3249759707272745768, 0.3333333333333333703, 0.3249759707272745768, 0.3333333333333333703, 0.3249759707272745768, 0.3333333333333333703, 0.3249759707272745768, 0.3333333333333333703, 0.3249759707272745768, 0.3333333333333333703, 0.3249759707272745768, 0.3333333333333333703, 0.3249759707272745768, 0.3333333333333333703, 0.3249759707272745768, 0.3333333333333333703, 0.3249759707272745768, 0.3333333333333333703, 0.3249759707272745768, 0.3333333333333333703, 0.3249759707272745768, 0.3333333333333333703, 0.3249759707272745768, 0.3333333333333333703, 0.3249759707272745768, 0.3333333333333333703, 0.3249759707272745768, 0.3333333333333333703, 0.3249759707272745768, 0.3333333333333333703, 0.3249759707272745768, 0.3333333333333333703, 0.3249759707272745768, 0.3333333333333333703, 0.3249759707272745768, 0.3333333333333333703, 0.3249759707272745768, 0.3333333333333333703, 0.3249759707272745768, 0.3333333333333333703, 0.3249759707272745768, 0.3333333333333333703, 0.3249759707272745768, 0.3333333333333333703, 0.3249759707272745768, 0.3333333333333333703, 0.3249759707272745768, 0.3333333333333333703, 0.3249759707272745768, 0.3333333333333333703, 0.3249759707272745768, 0.3333333333333333703, 0.3249759707272745768, 0.3333333333333333703, 0.3249759707272745768, 0.3333333333333333703, 0.3249759707272745768, 0.3333333333333333703, 0.3249759707272745768, 0.3333333333333333703, 0.3249759707272745768, 0.3333333333333333703, 0.3249759707272745768, 0.3333333333333333703, 0.3249759707272745768, 0.3333333333333333703, 0.3249759707272745768, 0.3333333333333333703, 0.3249759707272745768, 0.3333333333333333703, 0.3249759707272745768, 0.3333333333333333703, 0.3249759707272745768, 0.3333333333333333703, 0.3249759707272745768, 0.3333333333333333703, 0.3249759707272745768, 0.3333333333333333703, 0.3249759707272745768, 0.3333333333333333703, 0.3249759707272745768, 0.3333333333333333703, 0.3249759707272745768, 0.3333333333333333703, 0.3249759707272745768, 0.3333333333333333703, 0.3249759707272745768, 0.3333333333333333703, 0.3249759707272745768, 0.3333333333333333703, 0.3249759707272745768, 0.3333333333333333703, 0.3249759707272745768, 0.3333333333333333703, 0.3249759707272745768, 0.3333333333333333703, 0.3249759707272745768, 0.3333333333333333703, 0.3249759707272745768, 0.3333333333333333703, 0.3249759707272745768, 0.3333333333333333703, 0.3249759707272745768, 0.3333333333333333703, 0.3249759707272745768, 0.3333333333333333703, 0.3249759707272745768, 0.3333333333333333703, 0.3249759707272745768, 0.3333333333333333703, 0.3249759707272745768, 0.3333333333333333703, 0.3249759707272745768, 0.3333333333333333703, 0.3249759707272745768, 0.3333333333333333703, 0.3249759707272745768, 0.3333333333333333703, 0.3249759707272745768, 0.3333333333333333703, 0.3249759707272745768, 0.3333333333333333703, 0.3249759707272745768, 0.3333333333333333703, 0.3249759707272745768, 0.3333333333333333703, 0.3249759707272745768, 0.3333333333333333703, 0.3249759707272745768, 0.3333333333333333703, 0.3249759707272745768, 0.3333333333333333703, 0.3249759707272745768, 0.3333333333333333703, 0.3249759707272745768, 0.3333333333333333703, 0.3249759707272745768, 0.3333333333333333703, 0.3249759707272745768, 0.3333333333333333703, 0.3249759707272745768, 0.3333333333333333703, 0.3249759707272745768, 0.3333333333333333703, 0.3249759707272745768, 0.3333333333333333703, 0.3249759707272745768, 0.3333333333333333703, 0.3249759707272745768, 0.3333333333333333703, 0.3249759707272745768, 0.3333333333333333703, 0.3249759707272745768, 0.3333333333333333703, 0.3249759707272745768, 0.3333333333333333703, 0.3249759707272745768, 0.3333333333333333703, 0.3249759707272745768, 0.3333333333333333703, 0.3249759707272745768, 0.3333333333333333703, 0.3249759707272745768, 0.3333333333333333703, 0.3249759707272745768, 0.3333333333333333703, 0.3249759707272745768, 0.3333333333333333703, 0.3249759707272745768, 0.3333333333333333703, 0.3249759707272745768, 0.3333333333333333703, 0.3249759707272745768, 0.3333333333333333703, 0.3249759707272745768, 0.3333333333333333703, 0.3249759707272745768, 0.3333333333333333703, 0.3249759707272745768, 0.3333333333333333703, 0.3249759707272745768, 0.3333333333333333703, 0.3249759707272745768, 0.3333333333333333703, 0.3249759707272745768, 0.3333333333333333703, 0.3249759707272745768, 0.3333333333333333703, 0.3249759707272745768, 0.3333333333333333703, 0.3249759707272745768, 0.3333333333333333703, 0.3249759707272745768, 0.3333333333333333703, 0.3249759707272745768, 0.3333333333333333703, 0.3249759707272745768, 0.3333333333333333703, 0.3249759707272745768, 0.3333333333333333703, 0.3249759707272745768, 0.3333333333333333703, 0.3249759707272745768, 0.3333333333333333703, 0.3249759707272745768, 0.3333333333333333703, 0.3249759707272745768, 0.3333333333333333703, 0.3249759707272745768, 0.3333333333333333703, 0.3249759707272745768, 0.3333333333333333703, 0.3249759707272745768, 0.3333333333333333703, 0.3249759707272745768, 0.3333333333333333703, 0.3249759707272745768, 0.3333333333333333703, 0.3249759707272745768, 0.3333333333333333703, 0.3249759707272745768, 0.3333333333333333703, 0.3249759707272745768, 0.3333333333333333703, 0.3249759707272745768, 0.3333333333333333703, 0.3249759707272745768, 0.3333333333333333703, 0.3249759707272745768, 0.3333333333333333703, 0.3291546520303039736, 0.3291546520303039736),
 ( 0.3333333333333333703, 0.3249759707272745768, 0.3333333333333333703, 0.3249759707272745768, 0.3333333333333333703, 0.3249759707272745768, 0.3333333333333333703, 0.3249759707272745768, 0.3333333333333333703, 0.3249759707272745768, 0.3333333333333333703, 0.3249759707272745768, 0.3333333333333333703, 0.3249759707272745768, 0.3333333333333333703, 0.3249759707272745768, 0.3333333333333333703, 0.3249759707272745768, 0.3333333333333333703, 0.3249759707272745768, 0.3333333333333333703, 0.3249759707272745768, 0.3333333333333333703, 0.3249759707272745768, 0.3333333333333333703, 0.3249759707272745768, 0.3333333333333333703, 0.3249759707272745768, 0.3333333333333333703, 0.3249759707272745768, 0.3333333333333333703, 0.3249759707272745768, 0.3333333333333333703, 0.3249759707272745768, 0.3333333333333333703, 0.3249759707272745768, 0.3333333333333333703, 0.3249759707272745768, 0.3333333333333333703, 0.3249759707272745768, 0.3333333333333333703, 0.3249759707272745768, 0.3333333333333333703, 0.3249759707272745768, 0.3333333333333333703, 0.3249759707272745768, 0.3333333333333333703, 0.3249759707272745768, 0.3333333333333333703, 0.3249759707272745768, 0.3333333333333333703, 0.3249759707272745768, 0.3333333333333333703, 0.3249759707272745768, 0.3333333333333333703, 0.3249759707272745768, 0.3333333333333333703, 0.3249759707272745768, 0.3333333333333333703, 0.3249759707272745768, 0.3333333333333333703, 0.3249759707272745768, 0.3333333333333333703, 0.3249759707272745768, 0.3333333333333333703, 0.3249759707272745768, 0.3333333333333333703, 0.3249759707272745768, 0.3333333333333333703, 0.3249759707272745768, 0.3333333333333333703, 0.3249759707272745768, 0.3333333333333333703, 0.3249759707272745768, 0.3333333333333333703, 0.3249759707272745768, 0.3333333333333333703, 0.3249759707272745768, 0.3333333333333333703, 0.3249759707272745768, 0.3333333333333333703, 0.3249759707272745768, 0.3333333333333333703, 0.3249759707272745768, 0.3333333333333333703, 0.3249759707272745768, 0.3333333333333333703, 0.3249759707272745768, 0.3333333333333333703, 0.3249759707272745768, 0.3333333333333333703, 0.3249759707272745768, 0.3333333333333333703, 0.3249759707272745768, 0.3333333333333333703, 0.3249759707272745768, 0.3333333333333333703, 0.3249759707272745768, 0.3333333333333333703, 0.3249759707272745768, 0.3333333333333333703, 0.3249759707272745768, 0.3333333333333333703, 0.3249759707272745768, 0.3333333333333333703, 0.3249759707272745768, 0.3333333333333333703, 0.3249759707272745768, 0.3333333333333333703, 0.3249759707272745768, 0.3333333333333333703, 0.3249759707272745768, 0.3333333333333333703, 0.3249759707272745768, 0.3333333333333333703, 0.3249759707272745768, 0.3333333333333333703, 0.3249759707272745768, 0.3333333333333333703, 0.3249759707272745768, 0.3333333333333333703, 0.3249759707272745768, 0.3333333333333333703, 0.3249759707272745768, 0.3333333333333333703, 0.3249759707272745768, 0.3333333333333333703, 0.3249759707272745768, 0.3333333333333333703, 0.3249759707272745768, 0.3333333333333333703, 0.3249759707272745768, 0.3333333333333333703, 0.3249759707272745768, 0.3333333333333333703, 0.3249759707272745768, 0.3333333333333333703, 0.3249759707272745768, 0.3333333333333333703, 0.3249759707272745768, 0.3333333333333333703, 0.3249759707272745768, 0.3333333333333333703, 0.3249759707272745768, 0.3333333333333333703, 0.3249759707272745768, 0.3333333333333333703, 0.3249759707272745768, 0.3333333333333333703, 0.3249759707272745768, 0.3333333333333333703, 0.3249759707272745768, 0.3333333333333333703, 0.3249759707272745768, 0.3333333333333333703, 0.3249759707272745768, 0.3333333333333333703, 0.3249759707272745768, 0.3333333333333333703, 0.3249759707272745768, 0.3333333333333333703, 0.3249759707272745768, 0.3333333333333333703, 0.3249759707272745768, 0.3333333333333333703, 0.3249759707272745768, 0.3333333333333333703, 0.3249759707272745768, 0.3333333333333333703, 0.3249759707272745768, 0.3333333333333333703, 0.3249759707272745768, 0.3333333333333333703, 0.3249759707272745768, 0.3333333333333333703, 0.3249759707272745768, 0.3333333333333333703, 0.3249759707272745768, 0.3333333333333333703, 0.3249759707272745768, 0.3333333333333333703, 0.3249759707272745768, 0.3333333333333333703, 0.3249759707272745768, 0.3333333333333333703, 0.3249759707272745768, 0.3333333333333333703, 0.3249759707272745768, 0.3333333333333333703, 0.3249759707272745768, 0.3333333333333333703, 0.3249759707272745768, 0.3333333333333333703, 0.3249759707272745768, 0.3333333333333333703, 0.3249759707272745768, 0.3333333333333333703, 0.3249759707272745768, 0.3333333333333333703, 0.3249759707272745768, 0.3333333333333333703, 0.3249759707272745768, 0.3333333333333333703, 0.3249759707272745768, 0.3333333333333333703, 0.3249759707272745768, 0.3333333333333333703, 0.3249759707272745768, 0.3333333333333333703, 0.3249759707272745768, 0.3333333333333333703, 0.3249759707272745768, 0.3333333333333333703, 0.3249759707272745768, 0.3333333333333333703, 0.3249759707272745768, 0.3333333333333333703, 0.3249759707272745768, 0.3333333333333333703, 0.3249759707272745768, 0.3333333333333333703, 0.3249759707272745768, 0.3333333333333333703, 0.3249759707272745768, 0.3333333333333333703, 0.3249759707272745768, 0.3333333333333333703, 0.3249759707272745768, 0.3333333333333333703, 0.3249759707272745768, 0.3333333333333333703, 0.3291546520303039736, 0.3291546520303039736),
 ( 1.000000000000000000, 0.9749279121818236193, 1.000000000000000000, 0.9749279121818236193, 1.000000000000000000, 0.9749279121818236193, 1.000000000000000000, 0.9749279121818236193, 1.000000000000000000, 0.9749279121818236193, 1.000000000000000000, 0.9749279121818236193, 1.000000000000000000, 0.9749279121818236193, 1.000000000000000000, 0.9749279121818236193, 1.000000000000000000, 0.9749279121818236193, 1.000000000000000000, 0.9749279121818236193, 1.000000000000000000, 0.9749279121818236193, 1.000000000000000000, 0.9749279121818236193, 1.000000000000000000, 0.9749279121818236193, 1.000000000000000000, 0.9749279121818236193, 1.000000000000000000, 0.9749279121818236193, 1.000000000000000000, 0.9749279121818236193, 1.000000000000000000, 0.9749279121818236193, 1.000000000000000000, 0.9749279121818236193, 1.000000000000000000, 0.9749279121818236193, 1.000000000000000000, 0.9749279121818236193, 1.000000000000000000, 0.9749279121818236193, 1.000000000000000000, 0.9749279121818236193, 1.000000000000000000, 0.9749279121818236193, 1.000000000000000000, 0.9749279121818236193, 1.000000000000000000, 0.9749279121818236193, 1.000000000000000000, 0.9749279121818236193, 1.000000000000000000, 0.9749279121818236193, 1.000000000000000000, 0.9749279121818236193, 1.000000000000000000, 0.9749279121818236193, 1.000000000000000000, 0.9749279121818236193, 1.000000000000000000, 0.9749279121818236193, 1.000000000000000000, 0.9749279121818236193, 1.000000000000000000, 0.9749279121818236193, 1.000000000000000000, 0.9749279121818236193, 1.000000000000000000, 0.9749279121818236193, 1.000000000000000000, 0.9749279121818236193, 1.000000000000000000, 0.9749279121818236193, 1.000000000000000000, 0.9749279121818236193, 1.000000000000000000, 0.9749279121818236193, 1.000000000000000000, 0.9749279121818236193, 1.000000000000000000, 0.9749279121818236193, 1.000000000000000000, 0.9749279121818236193, 1.000000000000000000, 0.9749279121818236193, 1.000000000000000000, 0.9749279121818236193, 1.000000000000000000, 0.9749279121818236193, 1.000000000000000000, 0.9749279121818236193, 1.000000000000000000, 0.9749279121818236193, 1.000000000000000000, 0.9749279121818236193, 1.000000000000000000, 0.9749279121818236193, 1.000000000000000000, 0.9749279121818236193, 1.000000000000000000, 0.9749279121818236193, 1.000000000000000000, 0.9749279121818236193, 1.000000000000000000, 0.9749279121818236193, 1.000000000000000000, 0.9749279121818236193, 1.000000000000000000, 0.9749279121818236193, 1.000000000000000000, 0.9749279121818236193, 1.000000000000000000, 0.9749279121818236193, 1.000000000000000000, 0.9749279121818236193, 1.000000000000000000, 0.9749279121818236193, 1.000000000000000000, 0.9749279121818236193, 1.000000000000000000, 0.9749279121818236193, 1.000000000000000000, 0.9749279121818236193, 1.000000000000000000, 0.9749279121818236193, 1.000000000000000000, 0.9749279121818236193, 1.000000000000000000, 0.9749279121818236193, 1.000000000000000000, 0.9749279121818236193, 1.000000000000000000, 0.9749279121818236193, 1.000000000000000000, 0.9749279121818236193, 1.000000000000000000, 0.9749279121818236193, 1.000000000000000000, 0.9749279121818236193, 1.000000000000000000, 0.9749279121818236193, 1.000000000000000000, 0.9749279121818236193, 1.000000000000000000, 0.9749279121818236193, 1.000000000000000000, 0.9749279121818236193, 1.000000000000000000, 0.9749279121818236193, 1.000000000000000000, 0.9749279121818236193, 1.000000000000000000, 0.9749279121818236193, 1.000000000000000000, 0.9749279121818236193, 1.000000000000000000, 0.9749279121818236193, 1.000000000000000000, 0.9749279121818236193, 1.000000000000000000, 0.9749279121818236193, 1.000000000000000000, 0.9749279121818236193, 1.000000000000000000, 0.9749279121818236193, 1.000000000000000000, 0.9749279121818236193, 1.000000000000000000, 0.9749279121818236193, 1.000000000000000000, 0.9749279121818236193, 1.000000000000000000, 0.9749279121818236193, 1.000000000000000000, 0.9749279121818236193, 1.000000000000000000, 0.9749279121818236193, 1.000000000000000000, 0.9749279121818236193, 1.000000000000000000, 0.9749279121818236193, 1.000000000000000000, 0.9749279121818236193, 1.000000000000000000, 0.9749279121818236193, 1.000000000000000000, 0.9749279121818236193, 1.000000000000000000, 0.9749279121818236193, 1.000000000000000000, 0.9749279121818236193, 1.000000000000000000, 0.9749279121818236193, 1.000000000000000000, 0.9749279121818236193, 1.000000000000000000, 0.9749279121818236193, 1.000000000000000000, 0.9749279121818236193, 1.000000000000000000, 0.9749279121818236193, 1.000000000000000000, 0.9749279121818236193, 1.000000000000000000, 0.9749279121818236193, 1.000000000000000000, 0.9749279121818236193, 1.000000000000000000, 0.9749279121818236193, 1.000000000000000000, 0.9749279121818236193, 1.000000000000000000, 0.9749279121818236193, 1.000000000000000000, 0.9749279121818236193, 1.000000000000000000, 0.9749279121818236193, 1.000000000000000000, 0.9749279121818236193, 1.000000000000000000, 0.9749279121818236193, 1.000000000000000000, 0.9749279121818236193, 1.000000000000000000, 0.9749279121818236193, 1.000000000000000000, 0.9749279121818236193, 1.000000000000000000, 0.9749279121818236193, 1.000000000000000000, 0.9874639560909117542, 0.9874639560909117542),
 ( 0.3333333333333333703, 0.3249759707272745768, 0.3333333333333333703, 0.3249759707272745768, 0.3333333333333333703, 0.3249759707272745768, 0.3333333333333333703, 0.3249759707272745768, 0.3333333333333333703, 0.3249759707272745768, 0.3333333333333333703, 0.3249759707272745768, 0.3333333333333333703, 0.3249759707272745768, 0.3333333333333333703, 0.3249759707272745768, 0.3333333333333333703, 0.3249759707272745768, 0.3333333333333333703, 0.3249759707272745768, 0.3333333333333333703, 0.3249759707272745768, 0.3333333333333333703, 0.3249759707272745768, 0.3333333333333333703, 0.3249759707272745768, 0.3333333333333333703, 0.3249759707272745768, 0.3333333333333333703, 0.3249759707272745768, 0.3333333333333333703, 0.3249759707272745768, 0.3333333333333333703, 0.3249759707272745768, 0.3333333333333333703, 0.3249759707272745768, 0.3333333333333333703, 0.3249759707272745768, 0.3333333333333333703, 0.3249759707272745768, 0.3333333333333333703, 0.3249759707272745768, 0.3333333333333333703, 0.3249759707272745768, 0.3333333333333333703, 0.3249759707272745768, 0.3333333333333333703, 0.3249759707272745768, 0.3333333333333333703, 0.3249759707272745768, 0.3333333333333333703, 0.3249759707272745768, 0.3333333333333333703, 0.3249759707272745768, 0.3333333333333333703, 0.3249759707272745768, 0.3333333333333333703, 0.3249759707272745768, 0.3333333333333333703, 0.3249759707272745768, 0.3333333333333333703, 0.3249759707272745768, 0.3333333333333333703, 0.3249759707272745768, 0.3333333333333333703, 0.3249759707272745768, 0.3333333333333333703, 0.3249759707272745768, 0.3333333333333333703, 0.3249759707272745768, 0.3333333333333333703, 0.3249759707272745768, 0.3333333333333333703, 0.3249759707272745768, 0.3333333333333333703, 0.3249759707272745768, 0.3333333333333333703, 0.3249759707272745768, 0.3333333333333333703, 0.3249759707272745768, 0.3333333333333333703, 0.3249759707272745768, 0.3333333333333333703, 0.3249759707272745768, 0.3333333333333333703, 0.3249759707272745768, 0.3333333333333333703, 0.3249759707272745768, 0.3333333333333333703, 0.3249759707272745768, 0.3333333333333333703, 0.3249759707272745768, 0.3333333333333333703, 0.3249759707272745768, 0.3333333333333333703, 0.3249759707272745768, 0.3333333333333333703, 0.3249759707272745768, 0.3333333333333333703, 0.3249759707272745768, 0.3333333333333333703, 0.3249759707272745768, 0.3333333333333333703, 0.3249759707272745768, 0.3333333333333333703, 0.3249759707272745768, 0.3333333333333333703, 0.3249759707272745768, 0.3333333333333333703, 0.3249759707272745768, 0.3333333333333333703, 0.3249759707272745768, 0.3333333333333333703, 0.3249759707272745768, 0.3333333333333333703, 0.3249759707272745768, 0.3333333333333333703, 0.3249759707272745768, 0.3333333333333333703, 0.3249759707272745768, 0.3333333333333333703, 0.3249759707272745768, 0.3333333333333333703, 0.3249759707272745768, 0.3333333333333333703, 0.3249759707272745768, 0.3333333333333333703, 0.3249759707272745768, 0.3333333333333333703, 0.3249759707272745768, 0.3333333333333333703, 0.3249759707272745768, 0.3333333333333333703, 0.3249759707272745768, 0.3333333333333333703, 0.3249759707272745768, 0.3333333333333333703, 0.3249759707272745768, 0.3333333333333333703, 0.3249759707272745768, 0.3333333333333333703, 0.3249759707272745768, 0.3333333333333333703, 0.3249759707272745768, 0.3333333333333333703, 0.3249759707272745768, 0.3333333333333333703, 0.3249759707272745768, 0.3333333333333333703, 0.3249759707272745768, 0.3333333333333333703, 0.3249759707272745768, 0.3333333333333333703, 0.3249759707272745768, 0.3333333333333333703, 0.3249759707272745768, 0.3333333333333333703, 0.3249759707272745768, 0.3333333333333333703, 0.3249759707272745768, 0.3333333333333333703, 0.3249759707272745768, 0.3333333333333333703, 0.3249759707272745768, 0.3333333333333333703, 0.3249759707272745768, 0.3333333333333333703, 0.3249759707272745768, 0.3333333333333333703, 0.3249759707272745768, 0.3333333333333333703, 0.3249759707272745768, 0.3333333333333333703, 0.3249759707272745768, 0.3333333333333333703, 0.3249759707272745768, 0.3333333333333333703, 0.3249759707272745768, 0.3333333333333333703, 0.3249759707272745768, 0.3333333333333333703, 0.3249759707272745768, 0.3333333333333333703, 0.3249759707272745768, 0.3333333333333333703, 0.3249759707272745768, 0.3333333333333333703, 0.3249759707272745768, 0.3333333333333333703, 0.3249759707272745768, 0.3333333333333333703, 0.3249759707272745768, 0.3333333333333333703, 0.3249759707272745768, 0.3333333333333333703, 0.3249759707272745768, 0.3333333333333333703, 0.3249759707272745768, 0.3333333333333333703, 0.3249759707272745768, 0.3333333333333333703, 0.3249759707272745768, 0.3333333333333333703, 0.3249759707272745768, 0.3333333333333333703, 0.3249759707272745768, 0.3333333333333333703, 0.3249759707272745768, 0.3333333333333333703, 0.3249759707272745768, 0.3333333333333333703, 0.3249759707272745768, 0.3333333333333333703, 0.3249759707272745768, 0.3333333333333333703, 0.3249759707272745768, 0.3333333333333333703, 0.3249759707272745768, 0.3333333333333333703, 0.3249759707272745768, 0.3333333333333333703, 0.3249759707272745768, 0.3333333333333333703, 0.3249759707272745768, 0.3333333333333333703, 0.3249759707272745768, 0.3333333333333333703, 0.3249759707272745768, 0.3333333333333333703, 0.3249759707272745768, 0.3333333333333333703, 0.3291546520303039736, 0.3291546520303039736),
 ( 0.3333333333333333703, 0.3249759707272745768, 0.3333333333333333703, 0.3249759707272745768, 0.3333333333333333703, 0.3249759707272745768, 0.3333333333333333703, 0.3249759707272745768, 0.3333333333333333703, 0.3249759707272745768, 0.3333333333333333703, 0.3249759707272745768, 0.3333333333333333703, 0.3249759707272745768, 0.3333333333333333703, 0.3249759707272745768, 0.3333333333333333703, 0.3249759707272745768, 0.3333333333333333703, 0.3249759707272745768, 0.3333333333333333703, 0.3249759707272745768, 0.3333333333333333703, 0.3249759707272745768, 0.3333333333333333703, 0.3249759707272745768, 0.3333333333333333703, 0.3249759707272745768, 0.3333333333333333703, 0.3249759707272745768, 0.3333333333333333703, 0.3249759707272745768, 0.3333333333333333703, 0.3249759707272745768, 0.3333333333333333703, 0.3249759707272745768, 0.3333333333333333703, 0.3249759707272745768, 0.3333333333333333703, 0.3249759707272745768, 0.3333333333333333703, 0.3249759707272745768, 0.3333333333333333703, 0.3249759707272745768, 0.3333333333333333703, 0.3249759707272745768, 0.3333333333333333703, 0.3249759707272745768, 0.3333333333333333703, 0.3249759707272745768, 0.3333333333333333703, 0.3249759707272745768, 0.3333333333333333703, 0.3249759707272745768, 0.3333333333333333703, 0.3249759707272745768, 0.3333333333333333703, 0.3249759707272745768, 0.3333333333333333703, 0.3249759707272745768, 0.3333333333333333703, 0.3249759707272745768, 0.3333333333333333703, 0.3249759707272745768, 0.3333333333333333703, 0.3249759707272745768, 0.3333333333333333703, 0.3249759707272745768, 0.3333333333333333703, 0.3249759707272745768, 0.3333333333333333703, 0.3249759707272745768, 0.3333333333333333703, 0.3249759707272745768, 0.3333333333333333703, 0.3249759707272745768, 0.3333333333333333703, 0.3249759707272745768, 0.3333333333333333703, 0.3249759707272745768, 0.3333333333333333703, 0.3249759707272745768, 0.3333333333333333703, 0.3249759707272745768, 0.3333333333333333703, 0.3249759707272745768, 0.3333333333333333703, 0.3249759707272745768, 0.3333333333333333703, 0.3249759707272745768, 0.3333333333333333703, 0.3249759707272745768, 0.3333333333333333703, 0.3249759707272745768, 0.3333333333333333703, 0.3249759707272745768, 0.3333333333333333703, 0.3249759707272745768, 0.3333333333333333703, 0.3249759707272745768, 0.3333333333333333703, 0.3249759707272745768, 0.3333333333333333703, 0.3249759707272745768, 0.3333333333333333703, 0.3249759707272745768, 0.3333333333333333703, 0.3249759707272745768, 0.3333333333333333703, 0.3249759707272745768, 0.3333333333333333703, 0.3249759707272745768, 0.3333333333333333703, 0.3249759707272745768, 0.3333333333333333703, 0.3249759707272745768, 0.3333333333333333703, 0.3249759707272745768, 0.3333333333333333703, 0.3249759707272745768, 0.3333333333333333703, 0.3249759707272745768, 0.3333333333333333703, 0.3249759707272745768, 0.3333333333333333703, 0.3249759707272745768, 0.3333333333333333703, 0.3249759707272745768, 0.3333333333333333703, 0.3249759707272745768, 0.3333333333333333703, 0.3249759707272745768, 0.3333333333333333703, 0.3249759707272745768, 0.3333333333333333703, 0.3249759707272745768, 0.3333333333333333703, 0.3249759707272745768, 0.3333333333333333703, 0.3249759707272745768, 0.3333333333333333703, 0.3249759707272745768, 0.3333333333333333703, 0.3249759707272745768, 0.3333333333333333703, 0.3249759707272745768, 0.3333333333333333703, 0.3249759707272745768, 0.3333333333333333703, 0.3249759707272745768, 0.3333333333333333703, 0.3249759707272745768, 0.3333333333333333703, 0.3249759707272745768, 0.3333333333333333703, 0.3249759707272745768, 0.3333333333333333703, 0.3249759707272745768, 0.3333333333333333703, 0.3249759707272745768, 0.3333333333333333703, 0.3249759707272745768, 0.3333333333333333703, 0.3249759707272745768, 0.3333333333333333703, 0.3249759707272745768, 0.3333333333333333703, 0.3249759707272745768, 0.3333333333333333703, 0.3249759707272745768, 0.3333333333333333703, 0.3249759707272745768, 0.3333333333333333703, 0.3249759707272745768, 0.3333333333333333703, 0.3249759707272745768, 0.3333333333333333703, 0.3249759707272745768, 0.3333333333333333703, 0.3249759707272745768, 0.3333333333333333703, 0.3249759707272745768, 0.3333333333333333703, 0.3249759707272745768, 0.3333333333333333703, 0.3249759707272745768, 0.3333333333333333703, 0.3249759707272745768, 0.3333333333333333703, 0.3249759707272745768, 0.3333333333333333703, 0.3249759707272745768, 0.3333333333333333703, 0.3249759707272745768, 0.3333333333333333703, 0.3249759707272745768, 0.3333333333333333703, 0.3249759707272745768, 0.3333333333333333703, 0.3249759707272745768, 0.3333333333333333703, 0.3249759707272745768, 0.3333333333333333703, 0.3249759707272745768, 0.3333333333333333703, 0.3249759707272745768, 0.3333333333333333703, 0.3249759707272745768, 0.3333333333333333703, 0.3249759707272745768, 0.3333333333333333703, 0.3249759707272745768, 0.3333333333333333703, 0.3249759707272745768, 0.3333333333333333703, 0.3249759707272745768, 0.3333333333333333703, 0.3249759707272745768, 0.3333333333333333703, 0.3249759707272745768, 0.3333333333333333703, 0.3249759707272745768, 0.3333333333333333703, 0.3249759707272745768, 0.3333333333333333703, 0.3249759707272745768, 0.3333333333333333703, 0.3249759707272745768, 0.3333333333333333703, 0.3249759707272745768, 0.3333333333333333703, 0.3291546520303039736, 0.3291546520303039736),
 ( 1.000000000000000000, 0.9749279121818236193, 1.000000000000000000, 0.9749279121818236193, 1.000000000000000000, 0.9749279121818236193, 1.000000000000000000, 0.9749279121818236193, 1.000000000000000000, 0.9749279121818236193, 1.000000000000000000, 0.9749279121818236193, 1.000000000000000000, 0.9749279121818236193, 1.000000000000000000, 0.9749279121818236193, 1.000000000000000000, 0.9749279121818236193, 1.000000000000000000, 0.9749279121818236193, 1.000000000000000000, 0.9749279121818236193, 1.000000000000000000, 0.9749279121818236193, 1.000000000000000000, 0.9749279121818236193, 1.000000000000000000, 0.9749279121818236193, 1.000000000000000000, 0.9749279121818236193, 1.000000000000000000, 0.9749279121818236193, 1.000000000000000000, 0.9749279121818236193, 1.000000000000000000, 0.9749279121818236193, 1.000000000000000000, 0.9749279121818236193, 1.000000000000000000, 0.9749279121818236193, 1.000000000000000000, 0.9749279121818236193, 1.000000000000000000, 0.9749279121818236193, 1.000000000000000000, 0.9749279121818236193, 1.000000000000000000, 0.9749279121818236193, 1.000000000000000000, 0.9749279121818236193, 1.000000000000000000, 0.9749279121818236193, 1.000000000000000000, 0.9749279121818236193, 1.000000000000000000, 0.9749279121818236193, 1.000000000000000000, 0.9749279121818236193, 1.000000000000000000, 0.9749279121818236193, 1.000000000000000000, 0.9749279121818236193, 1.000000000000000000, 0.9749279121818236193, 1.000000000000000000, 0.9749279121818236193, 1.000000000000000000, 0.9749279121818236193, 1.000000000000000000, 0.9749279121818236193, 1.000000000000000000, 0.9749279121818236193, 1.000000000000000000, 0.9749279121818236193, 1.000000000000000000, 0.9749279121818236193, 1.000000000000000000, 0.9749279121818236193, 1.000000000000000000, 0.9749279121818236193, 1.000000000000000000, 0.9749279121818236193, 1.000000000000000000, 0.9749279121818236193, 1.000000000000000000, 0.9749279121818236193, 1.000000000000000000, 0.9749279121818236193, 1.000000000000000000, 0.9749279121818236193, 1.000000000000000000, 0.9749279121818236193, 1.000000000000000000, 0.9749279121818236193, 1.000000000000000000, 0.9749279121818236193, 1.000000000000000000, 0.9749279121818236193, 1.000000000000000000, 0.9749279121818236193, 1.000000000000000000, 0.9749279121818236193, 1.000000000000000000, 0.9749279121818236193, 1.000000000000000000, 0.9749279121818236193, 1.000000000000000000, 0.9749279121818236193, 1.000000000000000000, 0.9749279121818236193, 1.000000000000000000, 0.9749279121818236193, 1.000000000000000000, 0.9749279121818236193, 1.000000000000000000, 0.9749279121818236193, 1.000000000000000000, 0.9749279121818236193, 1.000000000000000000, 0.9749279121818236193, 1.000000000000000000, 0.9749279121818236193, 1.000000000000000000, 0.9749279121818236193, 1.000000000000000000, 0.9749279121818236193, 1.000000000000000000, 0.9749279121818236193, 1.000000000000000000, 0.9749279121818236193, 1.000000000000000000, 0.9749279121818236193, 1.000000000000000000, 0.9749279121818236193, 1.000000000000000000, 0.9749279121818236193, 1.000000000000000000, 0.9749279121818236193, 1.000000000000000000, 0.9749279121818236193, 1.000000000000000000, 0.9749279121818236193, 1.000000000000000000, 0.9749279121818236193, 1.000000000000000000, 0.9749279121818236193, 1.000000000000000000, 0.9749279121818236193, 1.000000000000000000, 0.9749279121818236193, 1.000000000000000000, 0.9749279121818236193, 1.000000000000000000, 0.9749279121818236193, 1.000000000000000000, 0.9749279121818236193, 1.000000000000000000, 0.9749279121818236193, 1.000000000000000000, 0.9749279121818236193, 1.000000000000000000, 0.9749279121818236193, 1.000000000000000000, 0.9749279121818236193, 1.000000000000000000, 0.9749279121818236193, 1.000000000000000000, 0.9749279121818236193, 1.000000000000000000, 0.9749279121818236193, 1.000000000000000000, 0.9749279121818236193, 1.000000000000000000, 0.9749279121818236193, 1.000000000000000000, 0.9749279121818236193, 1.000000000000000000, 0.9749279121818236193, 1.000000000000000000, 0.9749279121818236193, 1.000000000000000000, 0.9749279121818236193, 1.000000000000000000, 0.9749279121818236193, 1.000000000000000000, 0.9749279121818236193, 1.000000000000000000, 0.9749279121818236193, 1.000000000000000000, 0.9749279121818236193, 1.000000000000000000, 0.9749279121818236193, 1.000000000000000000, 0.9749279121818236193, 1.000000000000000000, 0.9749279121818236193, 1.000000000000000000, 0.9749279121818236193, 1.000000000000000000, 0.9749279121818236193, 1.000000000000000000, 0.9749279121818236193, 1.000000000000000000, 0.9749279121818236193, 1.000000000000000000, 0.9749279121818236193, 1.000000000000000000, 0.9749279121818236193, 1.000000000000000000, 0.9749279121818236193, 1.000000000000000000, 0.9749279121818236193, 1.000000000000000000, 0.9749279121818236193, 1.000000000000000000, 0.9749279121818236193, 1.000000000000000000, 0.9749279121818236193, 1.000000000000000000, 0.9749279121818236193, 1.000000000000000000, 0.9749279121818236193, 1.000000000000000000, 0.9749279121818236193, 1.000000000000000000, 0.9749279121818236193, 1.000000000000000000, 0.9749279121818236193, 1.000000000000000000, 0.9749279121818236193, 1.000000000000000000, 0.9874639560909117542, 0.9874639560909117542) ) ) 
 REPRESENTATION_ITEM ( '' )  SURFACE ( )  );
#7388=CARTESIAN_POINT ( 'NONE',  ( 14.28433602490915000, -1.478298951650544479, 34.35310228751642825 ) ) ;
#7393=CARTESIAN_POINT ( 'NONE',  ( -10.24623928997352351, -10.06191849875416899, 14.50404056962643651 ) ) ;
#7396=CARTESIAN_POINT ( 'NONE',  ( -12.08964793087886314, 7.750357176954159932, 21.78975485534072476 ) ) ;
#7398=CARTESIAN_POINT ( 'NONE',  ( 8.404922754268618235, 13.61519076058357491, 39.28167371608785174 ) ) ;
#7399=CARTESIAN_POINT ( 'NONE',  ( -0.3453160816774686892, 15.99627321608801367, 48.73000000000002530 ) ) ;
#7400=CARTESIAN_POINT ( 'NONE',  ( -8.841785722321695573, 13.82664651025757152, 8.210245144659282346 ) ) ;
#7406=CARTESIAN_POINT ( 'NONE',  ( 15.53355953199861794, 5.297344310588528060, 35.93261199819787066 ) ) ;
#7407=CARTESIAN_POINT ( 'NONE',  ( -7.639999817571787588, 12.15899005565156266, 24.21428571428571530 ) ) ;
#7408=CARTESIAN_POINT ( 'NONE',  ( 9.899494936611718643, -9.899494936611608509, 39.00000000000000000 ) ) ;
#7410=CARTESIAN_POINT ( 'NONE',  ( -5.420364854931999155, -15.49051278174644253, 46.07142857142856940 ) ) ;
#7412=CARTESIAN_POINT ( 'NONE',  ( -15.49051278174638036, -5.420364854932175902, 22.92857142857142705 ) ) ;
#7417=CARTESIAN_POINT ( 'NONE',  ( -1.917699372585823570, -15.88516839912900558, 7.861183426769288829 ) ) ;
#7418=CARTESIAN_POINT ( 'NONE',  ( -1.837501619626328297, 16.30827793483733856, 24.64285714285714235 ) ) ;
#7419=DIRECTION ( 'NONE',  ( 1.000000000000000000, 0.000000000000000000, 0.000000000000000000 ) ) ;
#7420=CARTESIAN_POINT ( 'NONE',  ( 1.707986654103998303, -16.32287076676380266, 7.646897712483577969 ) ) ;
#7422=CARTESIAN_POINT ( 'NONE',  ( -12.15899005565164792, 7.639999817571651697, 17.78571428571428115 ) ) ;
#7424=CARTESIAN_POINT ( 'NONE',  ( 15.49051278174638036, 5.420364854932175014, 7.928571428571430602 ) ) ;
#7427=CARTESIAN_POINT ( 'NONE',  ( 13.21436662431716869, -4.623906867372263640, 14.57142857142856940 ) ) ;
#7428=CARTESIAN_POINT ( 'NONE',  ( 15.89939535829187278, 1.791431617653015174, 26.14285714285714590 ) ) ;
#7431=CARTESIAN_POINT ( 'NONE',  ( 7.340858601237956194, 11.92174236212700045, 3.281673716087854409 ) ) ;
#7433=CARTESIAN_POINT ( 'NONE',  ( 1.607813917173037899, -14.26974319298267169, 9.642857142857144126 ) ) ;
#7437=CARTESIAN_POINT ( 'NONE',  ( -12.22833218042443271, 7.529642458189139909, 31.78167371608784819 ) ) ;
#7442=CARTESIAN_POINT ( 'NONE',  ( 12.22833218042443271, -7.529642458189144349, 46.78167371608785885 ) ) ;
#7448=CARTESIAN_POINT ( 'NONE',  ( -13.59724543428031573, -4.619798703722008959, 20.93261199819787066 ) ) ;
#7450=CARTESIAN_POINT ( 'NONE',  ( 5.297344310588354865, 15.53355953199867301, 45.06738800180215065 ) ) ;
#7453=CARTESIAN_POINT ( 'NONE',  ( -8.512513224245306986, -13.54758718765259218, 22.28571428571428470 ) ) ;
#7458=CARTESIAN_POINT ( 'NONE',  ( -13.61519076058348254, -8.404922754268771001, 38.71832628391214826 ) ) ;
#7459=CARTESIAN_POINT ( 'NONE',  ( 12.15899005565164792, -7.639999817571655250, 26.78571428571429536 ) ) ;
#7461=CARTESIAN_POINT ( 'NONE',  ( 11.85413878919593422, 7.448449071214774619, 43.71428571428572241 ) ) ;
#7463=CARTESIAN_POINT ( 'NONE',  ( -11.60466159355861926, -11.60466159355875249, 46.50000000000002132 ) ) ;
#7465=CARTESIAN_POINT ( 'NONE',  ( -1.791431617652833763, -15.89939535829188877, 9.857142857142855874 ) ) ;
#7467=CARTESIAN_POINT ( 'NONE',  ( -0.3453160816774686892, 15.99627321608801367, 48.73000000000002530 ) ) ;
#7470=CARTESIAN_POINT ( 'NONE',  ( -16.29368510291090288, 1.967016585148476215, 9.361183426769292382 ) ) ;
#7471=CARTESIAN_POINT ( 'NONE',  ( -1.791431617652833763, -15.89939535829188877, 27.85714285714285765 ) ) ;
#7473=CARTESIAN_POINT ( 'NONE',  ( 1.917699372585825790, 15.88516839912900203, 10.86118342676929238 ) ) ;
#7475=CARTESIAN_POINT ( 'NONE',  ( -14.26974319298268767, 1.607813917172874918, 23.35714285714286476 ) ) ;
#7476=CARTESIAN_POINT ( 'NONE',  ( 15.10213328493390783, -5.284464991282587398, 8.571428571428569398 ) ) ;
#7479=CARTESIAN_POINT ( 'NONE',  ( -7.448449071214644945, -11.85413878919601771, 10.28571428571428648 ) ) ;
#7481=CARTESIAN_POINT ( 'NONE',  ( 1.791431617652837316, 15.89939535829188877, 36.85714285714286120 ) ) ;
#7482=CARTESIAN_POINT ( 'NONE',  ( 1.665163862719847732, 15.91362231745477374, 44.85310228751641404 ) ) ;
#7486=CARTESIAN_POINT ( 'NONE',  ( -4.623906867372410190, 13.21436662431711895, 6.428571428571429713 ) ) ;
#7488=CARTESIAN_POINT ( 'NONE',  ( 13.51115193377584589, 4.865839792409294873, 21.92453085894500120 ) ) ;
#7493=CARTESIAN_POINT ( 'NONE',  ( 9.899494936611718643, -9.899494936611608509, 3.000000000000002665 ) ) ;
#7497=CARTESIAN_POINT ( 'NONE',  ( 11.92174236212692229, 7.340858601238088532, 29.71832628391214826 ) ) ;
#7499=CARTESIAN_POINT ( 'NONE',  ( -4.865839792409144771, -13.51115193377589740, 26.07546914105500235 ) ) ;
#7501=CARTESIAN_POINT ( 'NONE',  ( -15.88516839912898071, -1.917699372586004980, 37.13881657323070584 ) ) ;
#7502=CARTESIAN_POINT ( 'NONE',  ( -9.131464984045058131, 12.92800615877343517, 48.72999999999997556 ) ) ;
#7503=CARTESIAN_POINT ( 'NONE',  ( 1.791431617652837316, 15.89939535829188877, 24.85714285714285765 ) ) ;
#7505=CARTESIAN_POINT ( 'NONE',  ( 1.737328882695370558, -14.25515036105620581, 17.63881657323070939 ) ) ;
#7510=CARTESIAN_POINT ( 'NONE',  ( 11.69682198916835070, 11.51250119794901394, 35.50404056962644006 ) ) ;
#7511=CARTESIAN_POINT ( 'NONE',  ( 11.85413878919593422, 7.448449071214774619, 31.71428571428571530 ) ) ;
#7512=CARTESIAN_POINT ( 'NONE',  ( -14.26974319298268767, 1.607813917172874918, 41.35714285714286120 ) ) ;
#7514=CARTESIAN_POINT ( 'NONE',  ( -15.89939535829186923, -1.791431617653016062, 47.14285714285714590 ) ) ;
#7515=CARTESIAN_POINT ( 'NONE',  ( -8.776584015271360784, 13.37184113485863790, -7.619501960618503881E-17 ) ) ;
#7516=CARTESIAN_POINT ( 'NONE',  ( -11.31370849898482156, 11.31370849898469544, 36.00000000000000711 ) ) ;
#7522=PRODUCT_DEFINITION_CONTEXT ( 'detailed design', #6245, 'design' ) ;
#7524=CARTESIAN_POINT ( 'NONE',  ( 13.82664651025767100, -8.841785722321541030, 6.789754855340717654 ) ) ;
#7525=CARTESIAN_POINT ( 'NONE',  ( 1.791431617652837316, 15.89939535829188877, 30.85714285714286120 ) ) ;
#7526=CARTESIAN_POINT ( 'NONE',  ( 11.22385875690717683, -11.40355824106234373, 13.00404056962644006 ) ) ;
#7527=CARTESIAN_POINT ( 'NONE',  ( 13.91197093850538380, 1.567502665446386390, 20.14285714285714235 ) ) ;
#7528=CARTESIAN_POINT ( 'NONE',  ( 1.837501619626330074, -16.30827793483733501, 3.642857142857144126 ) ) ;
#7529=CARTESIAN_POINT ( 'NONE',  ( -15.89939535829186923, -1.791431617653016062, 41.14285714285714590 ) ) ;
#7531=CARTESIAN_POINT ( 'NONE',  ( -4.623906867372410190, 13.21436662431711895, 18.42857142857143415 ) ) ;
#7533=CARTESIAN_POINT ( 'NONE',  ( 15.49051278174637858, 5.420364854932174126, 37.92857142857143060 ) ) ;
#7534=CARTESIAN_POINT ( 'NONE',  ( -1.441234910513241818, -13.92619789766829008, 5.853102287516418478 ) ) ;
#7537=CARTESIAN_POINT ( 'NONE',  ( -12.15899005565164792, 7.639999817571650809, 5.785714285714282923 ) ) ;
#7538=AXIS2_PLACEMENT_3D ( 'NONE', #2548, #8124, #904 ) ;
#7539=CARTESIAN_POINT ( 'NONE',  ( -7.750357176954294935, 12.08964793087877787, 26.21024514465928945 ) ) ;
#7547=CARTESIAN_POINT ( 'NONE',  ( 9.809645194534072132, -9.989344678689256796, 31.00404056962644006 ) ) ;
#7550=CARTESIAN_POINT ( 'NONE',  ( 15.44746603149413922, 5.543385399275817527, 45.92453085894500475 ) ) ;
#7555=CARTESIAN_POINT ( 'NONE',  ( -13.25633410266679313, 4.503970704919840529, 19.56738800180213644 ) ) ;
#7559=CARTESIAN_POINT ( 'NONE',  ( -8.621071003556675549, 13.96533075980314642, 40.21832628391215536 ) ) ;
#7560=CARTESIAN_POINT ( 'NONE',  ( -4.503970704919988854, 13.25633410266674517, -1.567388001802134223 ) ) ;
#7561=CARTESIAN_POINT ( 'NONE',  ( 1.607813917173038121, -14.26974319298267346, 39.64285714285716722 ) ) ;
#7564=CARTESIAN_POINT ( 'NONE',  ( 11.60466159355862104, 11.60466159355875071, 43.50000000000000711 ) ) ;
#7566=CARTESIAN_POINT ( 'NONE',  ( -5.420364854931999155, -15.49051278174644253, 34.07142857142859071 ) ) ;
#7574=CARTESIAN_POINT ( 'NONE',  ( -13.61519076058348254, -8.404922754268771001, 14.71832628391215003 ) ) ;
#7575=CARTESIAN_POINT ( 'NONE',  ( 15.89939535829187278, 1.791431617653015174, 44.14285714285714590 ) ) ;
#7576=CARTESIAN_POINT ( 'NONE',  ( 11.22385875690717683, -11.40355824106234373, 7.004040569626434731 ) ) ;
#7577=CARTESIAN_POINT ( 'NONE',  ( -13.21436662431716869, 4.623906867372262752, 17.57142857142856940 ) ) ;
#7578=CARTESIAN_POINT ( 'NONE',  ( 11.31370849898482334, -11.31370849898469366, 3.000000000000002665 ) ) ;
#7579=CARTESIAN_POINT ( 'NONE',  ( -5.284464991282755264, 15.10213328493384743, 48.42857142857143060 ) ) ;
#7583=CARTESIAN_POINT ( 'NONE',  ( 11.60466159355861926, 11.60466159355874716, 25.50000000000000355 ) ) ;
#7584=CARTESIAN_POINT ( 'NONE',  ( -15.14410076328353227, 5.164528828830164287, 49.56738800180214355 ) ) ;
#7587=CARTESIAN_POINT ( 'NONE',  ( -1.607813917173034124, 14.26974319298267346, 24.64285714285714235 ) ) ;
#7589=ORIENTED_EDGE ( 'NONE', *, *, #5165, .F. ) ;
#7590=CARTESIAN_POINT ( 'NONE',  ( -13.51115193377584589, -4.865839792409295761, 36.92453085894499765 ) ) ;
#7594=CARTESIAN_POINT ( 'NONE',  ( 15.44746603149413922, 5.543385399275817527, 9.924530858944988765 ) ) ;
#7597=CARTESIAN_POINT ( 'NONE',  ( -1.441234910513241818, -13.92619789766829008, 47.85310228751642114 ) ) ;
#7601=CARTESIAN_POINT ( 'NONE',  ( 7.529642458189280241, -12.22833218042435099, 31.21832628391215536 ) ) ;
#7608=CARTESIAN_POINT ( 'NONE',  ( 11.51250119794888249, 11.69682198916847682, 33.49595943037355994 ) ) ;
#7609=CARTESIAN_POINT ( 'NONE',  ( -13.19169480182751464, 7.515308610800390809, 48.73000000000003951 ) ) ;
#7612=CARTESIAN_POINT ( 'NONE',  ( -7.750357176954294935, 12.08964793087877787, 14.21024514465927702 ) ) ;
#7616=CARTESIAN_POINT ( 'NONE',  ( 13.55419868402807992, 4.742819248065648807, 43.92857142857143060 ) ) ;
#7618=CARTESIAN_POINT ( 'NONE',  ( 4.503970704919991519, -13.25633410266674517, 1.432611998197868219 ) ) ;
#7620=CARTESIAN_POINT ( 'NONE',  ( 13.89598863503046111, -8.731428362939032795, 44.78571428571428470 ) ) ;
#7621=CARTESIAN_POINT ( 'NONE',  ( -7.654268191094239171, 14.02309213130659593, -7.619501960615842708E-17 ) ) ;
#7623=CARTESIAN_POINT ( 'NONE',  ( -11.31370849898482156, 11.31370849898469544, 24.00000000000000000 ) ) ;
#7632=CARTESIAN_POINT ( 'NONE',  ( -15.10213328493390961, 5.284464991282586510, 41.57142857142856940 ) ) ;
#7633=CARTESIAN_POINT ( 'NONE',  ( -5.543385399275643444, -15.44746603149420494, 26.07546914105500235 ) ) ;
#7635=CARTESIAN_POINT ( 'NONE',  ( -12.15899005565164792, 7.639999817571651697, 23.78571428571429536 ) ) ;
#7636=CARTESIAN_POINT ( 'NONE',  ( -16.30827793483735988, 1.837501619626141780, 5.357142857142856762 ) ) ;
#7637=CARTESIAN_POINT ( 'NONE',  ( -5.420364854931999155, -15.49051278174644253, 46.07142857142856940 ) ) ;
#7642=CARTESIAN_POINT ( 'NONE',  ( 8.404922754268618235, 13.61519076058357491, 51.28167371608785174 ) ) ;
#7644=CARTESIAN_POINT ( 'NONE',  ( -5.284464991282755264, 15.10213328493384743, 0.4285714285714309346 ) ) ;
#7645=CARTESIAN_POINT ( 'NONE',  ( 5.543385399275644332, 15.44746603149420494, 47.07546914105501656 ) ) ;
#7648=CARTESIAN_POINT ( 'NONE',  ( 12.15899005565164792, -7.639999817571654361, 20.78571428571428825 ) ) ;
#7650=CARTESIAN_POINT ( 'NONE',  ( 12.22833218042443271, -7.529642458189144349, 34.78167371608785885 ) ) ;
#7653=CARTESIAN_POINT ( 'NONE',  ( -1.967016585148659846, 16.29368510291087091, 20.63881657323070939 ) ) ;
#7654=CARTESIAN_POINT ( 'NONE',  ( -13.54758718765249625, -8.512513224245459753, 4.714285714285712636 ) ) ;
#7658=CARTESIAN_POINT ( 'NONE',  ( -10.06191849875405531, -10.24623928997363542, 48.49595943037355994 ) ) ;
#7662=CARTESIAN_POINT ( 'NONE',  ( 7.529642458189280241, -12.22833218042435099, 25.21832628391215181 ) ) ;
#7666=CARTESIAN_POINT ( 'NONE',  ( 1.665163862719847732, 15.91362231745477374, 50.85310228751642825 ) ) ;
#7668=CARTESIAN_POINT ( 'NONE',  ( -13.54758718765249625, -8.512513224245459753, 28.71428571428571530 ) ) ;
#7671=CARTESIAN_POINT ( 'NONE',  ( -12.22833218042443271, 7.529642458189139909, 19.78167371608784819 ) ) ;
#7675=CARTESIAN_POINT ( 'NONE',  ( 11.69682198916835070, 11.51250119794901394, 41.50404056962644006 ) ) ;
#7676=CARTESIAN_POINT ( 'NONE',  ( 13.91197093850538380, 1.567502665446386390, 44.14285714285714590 ) ) ;
#7677=CARTESIAN_POINT ( 'NONE',  ( 4.742819248065503146, 13.55419868402813677, 49.07142857142859071 ) ) ;
#7679=CARTESIAN_POINT ( 'NONE',  ( 13.96533075980324234, -8.621071003556521006, 10.78167371608784819 ) ) ;
#7681=CARTESIAN_POINT ( 'NONE',  ( -5.284464991282755264, 15.10213328493384743, 36.42857142857143060 ) ) ;
#7688=CARTESIAN_POINT ( 'NONE',  ( -13.54758718765249625, -8.512513224245459753, 46.71428571428571530 ) ) ;
#7689=CARTESIAN_POINT ( 'NONE',  ( -15.06016580658428694, 5.404401153735006957, 21.57546914105500946 ) ) ;
#7690=CARTESIAN_POINT ( 'NONE',  ( 11.85413878919593422, 7.448449071214774619, 31.71428571428571530 ) ) ;
#7691=CARTESIAN_POINT ( 'NONE',  ( 5.284464991282756152, -15.10213328493384743, 15.42857142857143060 ) ) ;
#7692=CARTESIAN_POINT ( 'NONE',  ( -11.60466159355861926, -11.60466159355875249, 46.50000000000002132 ) ) ;
#7696=CARTESIAN_POINT ( 'NONE',  ( 8.731428362939189114, -13.89598863503035986, 39.21428571428571530 ) ) ;
#7699=CARTESIAN_POINT ( 'NONE',  ( 5.420364854932001819, 15.49051278174644430, 7.071428571428569398 ) ) ;
#7700=CARTESIAN_POINT ( 'NONE',  ( 1.707986654103998303, -16.32287076676380266, 43.64689771248358596 ) ) ;
#7702=CARTESIAN_POINT ( 'NONE',  ( -1.607813917173034124, 14.26974319298267346, 18.64285714285715301 ) ) ;
#7703=CARTESIAN_POINT ( 'NONE',  ( 1.737328882695370558, -14.25515036105620581, 47.63881657323071295 ) ) ;
#7706=CARTESIAN_POINT ( 'NONE',  ( 8.404922754268618235, 13.61519076058357491, 21.28167371608785530 ) ) ;
#7707=CARTESIAN_POINT ( 'NONE',  ( -11.31370849898482156, 11.31370849898469544, 0.000000000000000000 ) ) ;
#7709=CARTESIAN_POINT ( 'NONE',  ( 13.47998361472151529, 8.620103694222146729, 27.71024514465928235 ) ) ;
#7713=CARTESIAN_POINT ( 'NONE',  ( -4.503970704919988854, 13.25633410266674517, 28.43261199819786356 ) ) ;
#7715=CARTESIAN_POINT ( 'NONE',  ( -7.340858601237953529, -11.92174236212700222, 6.281673716087846415 ) ) ;
#7718=CARTESIAN_POINT ( 'NONE',  ( -13.89598863503046111, 8.731428362939027465, 29.78571428571428825 ) ) ;
#7721=CARTESIAN_POINT ( 'NONE',  ( 7.340858601237956194, 11.92174236212700045, 21.28167371608785530 ) ) ;
#7725=CARTESIAN_POINT ( 'NONE',  ( 14.26974319298268767, -1.607813917172876916, 44.35714285714287541 ) ) ;
#7727=CARTESIAN_POINT ( 'NONE',  ( -9.899494936611716867, 9.899494936611610285, 48.00000000000000000 ) ) ;
#7729=CARTESIAN_POINT ( 'NONE',  ( 13.47998361472151529, 8.620103694222146729, 3.710245144659281458 ) ) ;
#7731=CARTESIAN_POINT ( 'NONE',  ( 15.49051278174638036, 5.420364854932175014, 25.92857142857142705 ) ) ;
#7739=CARTESIAN_POINT ( 'NONE',  ( -11.31370849898482156, 11.31370849898469544, 48.00000000000000000 ) ) ;
#7740=CARTESIAN_POINT ( 'NONE',  ( 1.707986654103998303, -16.32287076676380266, 13.64689771248357708 ) ) ;
#7741=CARTESIAN_POINT ( 'NONE',  ( 8.512513224245308763, 13.54758718765259040, 13.28571428571429003 ) ) ;
#7746=CARTESIAN_POINT ( 'NONE',  ( -15.49051278174637858, -5.420364854932175014, 40.92857142857143771 ) ) ;
#7748=CARTESIAN_POINT ( 'NONE',  ( 15.49051278174638036, 5.420364854932175014, 1.928571428571430380 ) ) ;
#7749=CARTESIAN_POINT ( 'NONE',  ( 4.623906867372411078, -13.21436662431711717, 27.42857142857143060 ) ) ;
#7752=CARTESIAN_POINT ( 'NONE',  ( 12.22833218042443271, -7.529642458189144349, 40.78167371608785885 ) ) ;
#7755=CARTESIAN_POINT ( 'NONE',  ( 15.44746603149413922, 5.543385399275817527, 21.92453085894500120 ) ) ;
#7757=CARTESIAN_POINT ( 'NONE',  ( -13.47998361472151174, -8.620103694222146729, 18.71024514465927879 ) ) ;
#7761=CARTESIAN_POINT ( 'NONE',  ( -1.693770420379220099, -13.89774397934251837, 43.86118342676930126 ) ) ;
#7765=CARTESIAN_POINT ( 'NONE',  ( -11.78653521626494793, -7.556039541191465148, 6.710245144659284122 ) ) ;
#7767=CARTESIAN_POINT ( 'NONE',  ( 15.89939535829187278, 1.791431617653015174, 26.14285714285714590 ) ) ;
#7769=CARTESIAN_POINT ( 'NONE',  ( 10.06191849875406064, 10.24623928997363187, 27.49595943037356705 ) ) ;
#7775=CARTESIAN_POINT ( 'NONE',  ( -1.917699372585823570, -15.88516839912900558, 43.86118342676930126 ) ) ;
#7776=CARTESIAN_POINT ( 'NONE',  ( -13.55419868402807992, -4.742819248065651472, 46.92857142857142350 ) ) ;
#7777=CARTESIAN_POINT ( 'NONE',  ( -13.21436662431716869, 4.623906867372262752, 47.57142857142857650 ) ) ;
#7780=CARTESIAN_POINT ( 'NONE',  ( -13.96533075980324234, 8.621071003556515677, 13.78167371608785174 ) ) ;
#7783=CARTESIAN_POINT ( 'NONE',  ( 16.30827793483735633, -1.837501619626142890, 38.35714285714287541 ) ) ;
#7790=CARTESIAN_POINT ( 'NONE',  ( 8.620103694221997515, 13.47998361472160767, 17.28975485534072121 ) ) ;
#7791=CARTESIAN_POINT ( 'NONE',  ( 15.49051278174638036, 5.420364854932175014, 43.92857142857143060 ) ) ;
#7793=CARTESIAN_POINT ( 'NONE',  ( 8.621071003556677326, -13.96533075980314287, 13.21832628391215181 ) ) ;
#7794=CARTESIAN_POINT ( 'NONE',  ( -15.10213328493390961, 5.284464991282586510, 23.57142857142857650 ) ) ;
#7798=CARTESIAN_POINT ( 'NONE',  ( -1.791431617652833763, -15.89939535829188877, 45.85714285714286120 ) ) ;
#7800=CARTESIAN_POINT ( 'NONE',  ( 8.620103694221997515, 13.47998361472160767, 47.28975485534072476 ) ) ;
#7801=CARTESIAN_POINT ( 'NONE',  ( 4.742819248065502258, 13.55419868402813499, 31.07142857142857295 ) ) ;
#7802=CARTESIAN_POINT ( 'NONE',  ( -14.25515036105622890, 1.737328882695209575, 33.36118342676929416 ) ) ;
#7804=CARTESIAN_POINT ( 'NONE',  ( -4.619798703721853528, -13.59724543428036725, 36.06738800180213644 ) ) ;
#7806=DIRECTION ( 'NONE',  ( 0.7071067811865519026, -0.7071067811865431318, 0.000000000000000000 ) ) ;
#7807=CARTESIAN_POINT ( 'NONE',  ( -8.404922754268618235, -13.61519076058357491, 18.28167371608785174 ) ) ;
#7809=CARTESIAN_POINT ( 'NONE',  ( -11.40355824106246807, 11.22385875690704715, 19.99595943037356349 ) ) ;
#7813=CARTESIAN_POINT ( 'NONE',  ( 10.06191849875406064, 10.24623928997363187, 9.495959430373563492 ) ) ;
#7816=CARTESIAN_POINT ( 'NONE',  ( -13.89774397934249706, -1.693770420379375974, 31.13881657323070939 ) ) ;
#7820=CARTESIAN_POINT ( 'NONE',  ( 8.620103694221997515, 13.47998361472160767, 47.28975485534072476 ) ) ;
#7821=CARTESIAN_POINT ( 'NONE',  ( -1.693770420379220099, -13.89774397934251837, 7.861183426769288829 ) ) ;
#7822=CARTESIAN_POINT ( 'NONE',  ( -4.503970704919988854, 13.25633410266674517, 4.432611998197859116 ) ) ;
#7824=CARTESIAN_POINT ( 'NONE',  ( 13.47998361472151529, 8.620103694222146729, 15.71024514465927879 ) ) ;
#7826=CARTESIAN_POINT ( 'NONE',  ( 5.420364854932001819, 15.49051278174644430, 37.07142857142857650 ) ) ;
#7832=CARTESIAN_POINT ( 'NONE',  ( 11.69682198916835070, 11.51250119794901394, 23.50404056962643295 ) ) ;
#7833=CARTESIAN_POINT ( 'NONE',  ( 8.512513224245308763, 13.54758718765259040, 19.28571428571428825 ) ) ;
#7835=CARTESIAN_POINT ( 'NONE',  ( -16.30827793483735988, 1.837501619626141780, 5.357142857142856762 ) ) ;
#7837=CARTESIAN_POINT ( 'NONE',  ( 16.30827793483735633, -1.837501619626142890, 44.35714285714286831 ) ) ;
#7840=CARTESIAN_POINT ( 'NONE',  ( 1.791431617652837316, 15.89939535829188877, 6.857142857142860315 ) ) ;
#7841=CARTESIAN_POINT ( 'NONE',  ( -15.10213328493390961, 5.284464991282586510, 11.57142857142857295 ) ) ;
#7843=CARTESIAN_POINT ( 'NONE',  ( 12.15899005565164792, -7.639999817571654361, 44.78571428571429180 ) ) ;
#7844=CARTESIAN_POINT ( 'NONE',  ( -13.92619789766827054, -1.441234910513399470, 33.14689771248357886 ) ) ;
#7848=CARTESIAN_POINT ( 'NONE',  ( 14.26974319298268767, -1.607813917172876916, 8.357142857142855874 ) ) ;
#7850=LINE ( 'NONE', #205, #1034 ) ;
#7851=CARTESIAN_POINT ( 'NONE',  ( 15.88516839912898071, 1.917699372586004092, 22.13881657323070939 ) ) ;
#7852=CARTESIAN_POINT ( 'NONE',  ( -16.30827793483735988, 1.837501619626141558, 5.357142857142856762 ) ) ;
#7854=CARTESIAN_POINT ( 'NONE',  ( -11.51250119794888072, -11.69682198916848037, 30.49595943037356349 ) ) ;
#7857=CARTESIAN_POINT ( 'NONE',  ( -10.15407889436378852, -10.15407889436390398, 4.500000000000003553 ) ) ;
#7860=CARTESIAN_POINT ( 'NONE',  ( 11.78653521626494793, 7.556039541191463371, 3.710245144659281458 ) ) ;
#7866=CARTESIAN_POINT ( 'NONE',  ( -1.478298951650703019, 14.28433602490913579, 4.646897712483579745 ) ) ;
#7868=CARTESIAN_POINT ( 'NONE',  ( 11.92174236212692229, 7.340858601238088532, 17.71832628391214826 ) ) ;
#7870=CARTESIAN_POINT ( 'NONE',  ( -15.14410076328353227, 5.164528828830164287, 7.567388001802139108 ) ) ;
#7872=CARTESIAN_POINT ( 'NONE',  ( -11.31370849898482156, 11.31370849898469544, 42.00000000000000000 ) ) ;
#7877=CARTESIAN_POINT ( 'NONE',  ( -11.60466159355861926, -11.60466159355875249, 34.50000000000000000 ) ) ;
#7879=CARTESIAN_POINT ( 'NONE',  ( -15.91362231745475597, -1.665163862720028254, 33.14689771248357886 ) ) ;
#7881=CARTESIAN_POINT ( 'NONE',  ( -15.91362231745475597, -1.665163862720028254, 33.14689771248357886 ) ) ;
#7883=CARTESIAN_POINT ( 'NONE',  ( 15.10213328493390783, -5.284464991282587398, 14.57142857142856940 ) ) ;
#7885=CARTESIAN_POINT ( 'NONE',  ( 15.10213328493390783, -5.284464991282587398, 2.571428571428571619 ) ) ;
#7890=CARTESIAN_POINT ( 'NONE',  ( -14.25515036105622890, 1.737328882695209575, 45.36118342676930837 ) ) ;
#7891=CARTESIAN_POINT ( 'NONE',  ( -16.30827793483735988, 1.837501619626141780, 11.35714285714285943 ) ) ;
#7892=CARTESIAN_POINT ( 'NONE',  ( 1.607813917173037899, -14.26974319298267169, 39.64285714285715301 ) ) ;
#7893=CARTESIAN_POINT ( 'NONE',  ( 13.17239914596754424, -4.743843029824685864, 30.57546914105500946 ) ) ;
#7897=CARTESIAN_POINT ( 'NONE',  ( -7.340858601237953529, -11.92174236212700222, 48.28167371608785174 ) ) ;
#7900=CARTESIAN_POINT ( 'NONE',  ( -5.404401153735176599, 15.06016580658422477, 32.42453085894499054 ) ) ;
#7901=CARTESIAN_POINT ( 'NONE',  ( 13.89598863503045933, -8.731428362939032795, 20.78571428571428825 ) ) ;
#7902=CARTESIAN_POINT ( 'NONE',  ( -15.44746603149413922, -5.543385399275820191, 18.92453085894499409 ) ) ;
#7910=CARTESIAN_POINT ( 'NONE',  ( 11.31370849898482334, -11.31370849898469366, 15.00000000000000000 ) ) ;
#7915=CARTESIAN_POINT ( 'NONE',  ( 11.92174236212692229, 7.340858601238088532, 11.71832628391215181 ) ) ;
#7917=CARTESIAN_POINT ( 'NONE',  ( -13.59724543428031573, -4.619798703722008959, 8.932611998197868886 ) ) ;
#7920=CARTESIAN_POINT ( 'NONE',  ( -8.841785722321695573, 13.82664651025757152, 2.210245144659280569 ) ) ;
#7929=CARTESIAN_POINT ( 'NONE',  ( -13.82664651025767100, 8.841785722321537477, 27.78975485534072121 ) ) ;
#7931=CARTESIAN_POINT ( 'NONE',  ( -5.164528828830334817, 15.14410076328347543, 34.43261199819786356 ) ) ;
#7935=CARTESIAN_POINT ( 'NONE',  ( 15.10213328493390783, -5.284464991282587398, 32.57142857142856940 ) ) ;
#7943=CARTESIAN_POINT ( 'NONE',  ( 5.543385399275644332, 15.44746603149420494, -0.9245308589449906522 ) ) ;
#7944=CARTESIAN_POINT ( 'NONE',  ( 11.31370849898482334, -11.31370849898469366, 15.00000000000000000 ) ) ;
#7946=CARTESIAN_POINT ( 'NONE',  ( -13.21436662431716869, 4.623906867372262752, 35.57142857142857650 ) ) ;
#7947=CARTESIAN_POINT ( 'NONE',  ( -13.59724543428031573, -4.619798703722008959, 44.93261199819787777 ) ) ;
#7948=CARTESIAN_POINT ( 'NONE',  ( 10.24623928997352884, 10.06191849875416899, 35.50404056962644006 ) ) ;
#7952=CARTESIAN_POINT ( 'NONE',  ( -13.51115193377584589, -4.865839792409295761, 48.92453085894499054 ) ) ;
#7955=CARTESIAN_POINT ( 'NONE',  ( 13.54758718765249803, 8.512513224245457977, 13.71428571428571352 ) ) ;
#7956=CARTESIAN_POINT ( 'NONE',  ( -11.51250119794888072, -11.69682198916848037, 42.49595943037355994 ) ) ;
#7960=PRESENTATION_STYLE_ASSIGNMENT (( #831 ) ) ;
#7962=CARTESIAN_POINT ( 'NONE',  ( 11.78653521626494793, 7.556039541191463371, 15.71024514465927879 ) ) ;
#7964=CARTESIAN_POINT ( 'NONE',  ( 5.284464991282756152, -15.10213328493384743, 15.42857142857143060 ) ) ;
#7966=CARTESIAN_POINT ( 'NONE',  ( 13.25633410266679313, -4.503970704919842305, 28.56738800180213644 ) ) ;
#7970=CARTESIAN_POINT ( 'NONE',  ( 7.556039541191335474, 11.78653521626503320, 5.289754855340725648 ) ) ;
#7972=CARTESIAN_POINT ( 'NONE',  ( -13.17239914596754424, 4.743843029824683200, 15.57546914105500413 ) ) ;
#7977=CARTESIAN_POINT ( 'NONE',  ( 16.30827793483735633, -1.837501619626142890, 44.35714285714287541 ) ) ;
#7983=CARTESIAN_POINT ( 'NONE',  ( -11.22385875690717327, 11.40355824106234550, 28.00404056962643651 ) ) ;
#7985=CARTESIAN_POINT ( 'NONE',  ( 11.22385875690717683, -11.40355824106234373, 31.00404056962644006 ) ) ;
#7987=CARTESIAN_POINT ( 'NONE',  ( -11.31370849898482156, 11.31370849898469544, 30.00000000000000355 ) ) ;
#7989=CARTESIAN_POINT ( 'NONE',  ( -15.89939535829186923, -1.791431617653016062, 5.142857142857143238 ) ) ;
#7993=CARTESIAN_POINT ( 'NONE',  ( -16.29368510291090288, 1.967016585148476215, 3.361183426769288385 ) ) ;
#7994=CARTESIAN_POINT ( 'NONE',  ( 8.731428362939190890, -13.89598863503036164, 21.21428571428571885 ) ) ;
#7995=CARTESIAN_POINT ( 'NONE',  ( -1.607813917173034124, 14.26974319298267346, 42.64285714285714590 ) ) ;
#7996=CARTESIAN_POINT ( 'NONE',  ( -4.865839792409144771, -13.51115193377589740, 38.07546914105502367 ) ) ;
#7997=CARTESIAN_POINT ( 'NONE',  ( 1.607813917173038121, -14.26974319298267346, 9.642857142857147679 ) ) ;
#8001=CARTESIAN_POINT ( 'NONE',  ( -13.21436662431716869, 4.623906867372262752, 5.571428571428574728 ) ) ;
#8003=CARTESIAN_POINT ( 'NONE',  ( -16.30827793483735988, 1.837501619626141558, 23.35714285714286120 ) ) ;
#8004=CARTESIAN_POINT ( 'NONE',  ( -5.404401153735176599, 15.06016580658422477, 44.42453085894499765 ) ) ;
#8009=CARTESIAN_POINT ( 'NONE',  ( -11.78653521626494793, -7.556039541191465148, 12.71024514465927879 ) ) ;
#8011=PRODUCT_DEFINITION ( 'UNKNOWN', '', #1132, #7522 ) ;
#8013=CARTESIAN_POINT ( 'NONE',  ( 1.441234910513245149, 13.92619789766829008, 32.85310228751642114 ) ) ;
#8017=CARTESIAN_POINT ( 'NONE',  ( 1.693770420379222319, 13.89774397934251837, 22.86118342676929061 ) ) ;
#8019=CARTESIAN_POINT ( 'NONE',  ( 10.24623928997352884, 10.06191849875416899, 17.50404056962643651 ) ) ;
#8022=CARTESIAN_POINT ( 'NONE',  ( 13.96533075980324234, -8.621071003556521006, 10.78167371608784819 ) ) ;
#8029=CARTESIAN_POINT ( 'NONE',  ( -16.29368510291090288, 1.967016585148476215, 27.36118342676929416 ) ) ;
#8031=CARTESIAN_POINT ( 'NONE',  ( -1.917699372585823570, -15.88516839912900558, 31.86118342676929416 ) ) ;
#8036=CARTESIAN_POINT ( 'NONE',  ( 5.420364854932001819, 15.49051278174644430, 37.07142857142857650 ) ) ;
#8037=CARTESIAN_POINT ( 'NONE',  ( -5.543139917359588331, 12.94619968565320711, 3.300085072504093742E-16 ) ) ;
#8038=CARTESIAN_POINT ( 'NONE',  ( 15.49051278174638036, 5.420364854932175014, 1.928571428571430380 ) ) ;
#8042=CARTESIAN_POINT ( 'NONE',  ( 16.29368510291089223, -1.967016585148476882, 0.3611834267692887734 ) ) ;
#8043=CARTESIAN_POINT ( 'NONE',  ( -8.731428362939189114, 13.89598863503036341, 12.21428571428571885 ) ) ;
#8044=CARTESIAN_POINT ( 'NONE',  ( 10.15407889436379030, 10.15407889436390221, 43.50000000000000711 ) ) ;
#8045=CARTESIAN_POINT ( 'NONE',  ( -11.22385875690717327, 11.40355824106234550, -1.995959430373561272 ) ) ;
#8046=CARTESIAN_POINT ( 'NONE',  ( -13.55419868402807992, -4.742819248065651472, 10.92857142857142883 ) ) ;
#8050=CARTESIAN_POINT ( 'NONE',  ( -4.623906867372410190, 13.21436662431711895, 6.428571428571429713 ) ) ;
#8052=CARTESIAN_POINT ( 'NONE',  ( -5.284464991282755264, 15.10213328493384743, 24.42857142857143060 ) ) ;
#8053=CARTESIAN_POINT ( 'NONE',  ( 8.841785722321695573, -13.82664651025757152, 41.21024514465928235 ) ) ;
#8060=CARTESIAN_POINT ( 'NONE',  ( -7.750357176954294935, 12.08964793087877787, 14.21024514465927702 ) ) ;
#8062=CARTESIAN_POINT ( 'NONE',  ( -15.10213328493390961, 5.284464991282586510, 11.57142857142857295 ) ) ;
#8064=CARTESIAN_POINT ( 'NONE',  ( 12.22833218042443271, -7.529642458189144349, 40.78167371608785885 ) ) ;
#8069=CARTESIAN_POINT ( 'NONE',  ( 13.92619789766827587, 1.441234910513398582, 18.14689771248357530 ) ) ;
#8071=CARTESIAN_POINT ( 'NONE',  ( 4.503970704919991519, -13.25633410266674517, 13.43261199819786711 ) ) ;
#8074=CARTESIAN_POINT ( 'NONE',  ( -15.44746603149413922, -5.543385399275820191, 6.924530858944994982 ) ) ;
#8080=CARTESIAN_POINT ( 'NONE',  ( 7.448449071214646722, 11.85413878919601594, 31.28571428571428470 ) ) ;
#8081=CARTESIAN_POINT ( 'NONE',  ( 1.917699372585825790, 15.88516839912900203, 28.86118342676929416 ) ) ;
#8084=CARTESIAN_POINT ( 'NONE',  ( -15.49051278174638036, -5.420364854932175902, 34.92857142857145192 ) ) ;
#8086=CARTESIAN_POINT ( 'NONE',  ( -15.89939535829186923, -1.791431617653016062, 17.14285714285713880 ) ) ;
#8092=CARTESIAN_POINT ( 'NONE',  ( 13.61519076058348254, 8.404922754268771001, -0.2816737160878517443 ) ) ;
#8094=CARTESIAN_POINT ( 'NONE',  ( -16.30827793483735988, 1.837501619626141780, 35.35714285714285410 ) ) ;
#8097=CARTESIAN_POINT ( 'NONE',  ( -7.448449071214644945, -11.85413878919601771, 46.28571428571429180 ) ) ;
#8098=CARTESIAN_POINT ( 'NONE',  ( 4.503970704919991519, -13.25633410266674517, 37.43261199819787066 ) ) ;
#8099=CARTESIAN_POINT ( 'NONE',  ( 16.30827793483735633, -1.837501619626142890, 38.35714285714287541 ) ) ;
#8100=CARTESIAN_POINT ( 'NONE',  ( -13.55419868402807992, -4.742819248065651472, 4.928571428571430602 ) ) ;
#8104=CARTESIAN_POINT ( 'NONE',  ( 13.55419868402807992, 4.742819248065648807, 13.92857142857143238 ) ) ;
#8109=CARTESIAN_POINT ( 'NONE',  ( -8.512513224245306986, -13.54758718765259218, 22.28571428571428470 ) ) ;
#8110=CARTESIAN_POINT ( 'NONE',  ( 1.967016585148662289, -16.29368510291087091, 41.63881657323070584 ) ) ;
#8113=CARTESIAN_POINT ( 'NONE',  ( -7.639999817571786700, 12.15899005565156266, 18.21428571428572241 ) ) ;
#8115=CARTESIAN_POINT ( 'NONE',  ( 13.89774397934249706, 1.693770420379375308, 16.13881657323070584 ) ) ;
#8119=CARTESIAN_POINT ( 'NONE',  ( -7.750357176954294935, 12.08964793087877787, 38.21024514465928235 ) ) ;
#8123=CARTESIAN_POINT ( 'NONE',  ( 4.503970704919991519, -13.25633410266674517, 13.43261199819786711 ) ) ;
#8124=DIRECTION ( 'NONE',  ( -0.7056782240951970930, 0.7056782240951883223, -0.06353336191096801977 ) ) ;
#8125=CARTESIAN_POINT ( 'NONE',  ( -8.841785722321695573, 13.82664651025757152, 14.21024514465927702 ) ) ;
#8131=CARTESIAN_POINT ( 'NONE',  ( -14.26974319298268767, 1.607813917172874918, 35.35714285714285410 ) ) ;
#8132=CARTESIAN_POINT ( 'NONE',  ( -1.607813917173034124, 14.26974319298267524, 36.64285714285714590 ) ) ;
#8134=CARTESIAN_POINT ( 'NONE',  ( -16.30827793483735988, 1.837501619626141780, 35.35714285714285410 ) ) ;
#8136=CARTESIAN_POINT ( 'NONE',  ( 8.731428362939190890, -13.89598863503036164, 15.21428571428571530 ) ) ;
#8139=CARTESIAN_POINT ( 'NONE',  ( 8.731428362939190890, -13.89598863503036164, 39.21428571428571530 ) ) ;
#8142=CARTESIAN_POINT ( 'NONE',  ( -15.06016580658428694, 5.404401153735006957, 15.57546914105500413 ) ) ;
#8143=CARTESIAN_POINT ( 'NONE',  ( -8.731428362939189114, 13.89598863503036341, 24.21428571428571530 ) ) ;
#8144=CARTESIAN_POINT ( 'NONE',  ( -13.91197093850538380, -1.567502665446387278, 47.14285714285714590 ) ) ;
#8145=CARTESIAN_POINT ( 'NONE',  ( -16.29368510291090288, 1.967016585148476215, 3.361183426769288385 ) ) ;
#8146=CARTESIAN_POINT ( 'NONE',  ( 12.15899005565164792, -7.639999817571655250, 8.785714285714293581 ) ) ;
#8150=CARTESIAN_POINT ( 'NONE',  ( -11.85413878919593422, -7.448449071214776396, 10.71428571428571708 ) ) ;
#8153=CARTESIAN_POINT ( 'NONE',  ( -1.837501619626327853, 16.30827793483733856, 30.64285714285714946 ) ) ;
#8154=CARTESIAN_POINT ( 'NONE',  ( 11.40355824106246985, -11.22385875690704538, 34.99595943037355994 ) ) ;
#8157=CARTESIAN_POINT ( 'NONE',  ( -9.899494936611716867, 9.899494936611610285, 11.99999999999999645 ) ) ;
#8158=CARTESIAN_POINT ( 'NONE',  ( 7.340858601237956194, 11.92174236212700045, 27.28167371608785174 ) ) ;
#8161=CARTESIAN_POINT ( 'NONE',  ( 10.06191849875406064, 10.24623928997363187, 33.49595943037355994 ) ) ;
#8166=CARTESIAN_POINT ( 'NONE',  ( -13.59724543428031573, -4.619798703722008959, 26.93261199819786356 ) ) ;
#8168=CARTESIAN_POINT ( 'NONE',  ( 8.841785722321695573, -13.82664651025757152, 41.21024514465928235 ) ) ;
#8170=CARTESIAN_POINT ( 'NONE',  ( -13.20632197976503086, 7.391146522708670119, 48.73000000000002530 ) ) ;
#8172=CARTESIAN_POINT ( 'NONE',  ( 5.420364854932001819, 15.49051278174644430, 19.07142857142856940 ) ) ;
#8173=CARTESIAN_POINT ( 'NONE',  ( 8.404922754268618235, 13.61519076058357491, 9.281673716087846415 ) ) ;
#8179=CARTESIAN_POINT ( 'NONE',  ( -8.621071003556675549, 13.96533075980314642, 34.21832628391215536 ) ) ;
#8180=CARTESIAN_POINT ( 'NONE',  ( -4.623906867372410190, 13.21436662431711895, 36.42857142857143060 ) ) ;
#8182=CARTESIAN_POINT ( 'NONE',  ( -4.623906867372410190, 13.21436662431711895, 36.42857142857143060 ) ) ;
#8184=CARTESIAN_POINT ( 'NONE',  ( 5.420364854932001819, 15.49051278174644430, 49.07142857142859071 ) ) ;
#8186=CARTESIAN_POINT ( 'NONE',  ( 1.837501619626330074, -16.30827793483733501, 9.642857142857147679 ) ) ;
#8190=CARTESIAN_POINT ( 'NONE',  ( 16.29368510291089223, -1.967016585148476882, 6.361183426769297711 ) ) ;
#8191=CARTESIAN_POINT ( 'NONE',  ( 11.60466159355862104, 11.60466159355875071, 25.50000000000000711 ) ) ;
#8193=CARTESIAN_POINT ( 'NONE',  ( -8.620103694221995738, -13.47998361472161299, 8.289754855340721207 ) ) ;
#8194=CARTESIAN_POINT ( 'NONE',  ( -13.55419868402807992, -4.742819248065651472, 16.92857142857143771 ) ) ;
#8198=CARTESIAN_POINT ( 'NONE',  ( -11.85413878919593422, -7.448449071214776396, 22.71428571428571530 ) ) ;
#8201=CARTESIAN_POINT ( 'NONE',  ( -11.60466159355861748, -11.60466159355874893, 34.50000000000000000 ) ) ;
#8202=CARTESIAN_POINT ( 'NONE',  ( -8.841785722321695573, 13.82664651025757152, 50.21024514465927524 ) ) ;
#8204=CARTESIAN_POINT ( 'NONE',  ( -10.15407889436378852, -10.15407889436390398, 10.50000000000000355 ) ) ;
#8206=CARTESIAN_POINT ( 'NONE',  ( 13.25633410266679313, -4.503970704919842305, 28.56738800180213644 ) ) ;
#8211=CARTESIAN_POINT ( 'NONE',  ( 11.78653521626494793, 7.556039541191463371, 39.71024514465927524 ) ) ;
#8214=CARTESIAN_POINT ( 'NONE',  ( 12.15899005565164792, -7.639999817571655250, 2.785714285714284255 ) ) ;
#8216=CARTESIAN_POINT ( 'NONE',  ( -1.693770420379220099, -13.89774397934251837, 19.86118342676929416 ) ) ;
#8219=CARTESIAN_POINT ( 'NONE',  ( 4.865839792409144771, 13.51115193377589740, 29.07546914105501301 ) ) ;
#8221=CARTESIAN_POINT ( 'NONE',  ( -8.404922754268618235, -13.61519076058357491, 42.28167371608785174 ) ) ;
#8222=CARTESIAN_POINT ( 'NONE',  ( -12.22926675870659174, 9.593933423190343035, 48.73000000000001819 ) ) ;
#8223=CARTESIAN_POINT ( 'NONE',  ( 8.731428362939190890, -13.89598863503036164, 21.21428571428571885 ) ) ;
#8224=CARTESIAN_POINT ( 'NONE',  ( -13.96533075980324234, 8.621071003556515677, 13.78167371608785174 ) ) ;
#8230=CARTESIAN_POINT ( 'NONE',  ( -11.69682198916834892, -11.51250119794901394, 38.50404056962644006 ) ) ;
#8231=CARTESIAN_POINT ( 'NONE',  ( -13.55419868402807992, -4.742819248065651472, 28.92857142857143771 ) ) ;
#8232=CARTESIAN_POINT ( 'NONE',  ( -7.448449071214644945, -11.85413878919601771, 40.28571428571428470 ) ) ;
#8234=CARTESIAN_POINT ( 'NONE',  ( 5.297344310588354865, 15.53355953199867301, 3.067388001802140884 ) ) ;
#8236=CARTESIAN_POINT ( 'NONE',  ( -15.89939535829186923, -1.791431617653016062, 11.14285714285714235 ) ) ;
#8241=CARTESIAN_POINT ( 'NONE',  ( 1.917699372585825790, 15.88516839912900203, 16.86118342676929061 ) ) ;
#8242=CARTESIAN_POINT ( 'NONE',  ( -15.89939535829186923, -1.791431617653016062, 35.14285714285713880 ) ) ;
#8245=CARTESIAN_POINT ( 'NONE',  ( 8.621071003556677326, -13.96533075980314287, 7.218326283912148256 ) ) ;
#8246=CARTESIAN_POINT ( 'NONE',  ( -7.448449071214644945, -11.85413878919601771, 22.28571428571428470 ) ) ;
#8247=CARTESIAN_POINT ( 'NONE',  ( -15.10213328493390961, 5.284464991282586510, 11.57142857142857295 ) ) ;
#8250=CARTESIAN_POINT ( 'NONE',  ( 13.91197093850538380, 1.567502665446386390, 20.14285714285714235 ) ) ;
#8252=CARTESIAN_POINT ( 'NONE',  ( -11.31370849898482156, 11.31370849898469544, 36.00000000000000711 ) ) ;
#8255=CARTESIAN_POINT ( 'NONE',  ( 15.88516839912898071, 1.917699372586004092, 46.13881657323070584 ) ) ;
#8258=CARTESIAN_POINT ( 'NONE',  ( -13.21436662431716869, 4.623906867372262752, 17.57142857142856940 ) ) ;
#8263=CARTESIAN_POINT ( 'NONE',  ( -13.89774397934249706, -1.693770420379375974, 25.13881657323070939 ) ) ;
#8267=CARTESIAN_POINT ( 'NONE',  ( 13.91197093850538380, 1.567502665446386390, 2.142857142857140573 ) ) ;
#8272=CARTESIAN_POINT ( 'NONE',  ( -13.17239914596754424, 4.743843029824683200, 33.57546914105500946 ) ) ;
#8274=CARTESIAN_POINT ( 'NONE',  ( -1.693770420379220099, -13.89774397934251837, 19.86118342676929416 ) ) ;
#8276=CARTESIAN_POINT ( 'NONE',  ( 5.404401153735178376, -15.06016580658422477, 35.42453085894499765 ) ) ;
#8277=CARTESIAN_POINT ( 'NONE',  ( -9.891020467832197127, 12.31459401221520800, 48.72999999999998977 ) ) ;
#8278=CARTESIAN_POINT ( 'NONE',  ( -13.89598863503046111, 8.731428362939027465, 17.78571428571428115 ) ) ;
#8280=CARTESIAN_POINT ( 'NONE',  ( 7.340858601237956194, 11.92174236212700045, 15.28167371608785174 ) ) ;
#8284=CARTESIAN_POINT ( 'NONE',  ( -1.707986654103994528, 16.32287076676380266, 34.64689771248358596 ) ) ;
#8285=CARTESIAN_POINT ( 'NONE',  ( -7.639999817571787588, 12.15899005565156266, 30.21428571428572596 ) ) ;
#8287=CARTESIAN_POINT ( 'NONE',  ( -4.742819248065502258, -13.55419868402813677, 40.07142857142857650 ) ) ;
#8289=CARTESIAN_POINT ( 'NONE',  ( 11.31370849898482334, -11.31370849898469366, 45.00000000000000711 ) ) ;
#8291=CARTESIAN_POINT ( 'NONE',  ( 15.10213328493390783, -5.284464991282587398, 14.57142857142856940 ) ) ;
#8299=CARTESIAN_POINT ( 'NONE',  ( 15.91362231745475597, 1.665163862720026255, 6.146897712483580634 ) ) ;
#8300=CARTESIAN_POINT ( 'NONE',  ( 5.284464991282756152, -15.10213328493384743, 27.42857142857143060 ) ) ;
#8302=CARTESIAN_POINT ( 'NONE',  ( 16.29368510291089223, -1.967016585148476882, 6.361183426769297711 ) ) ;
#8304=CARTESIAN_POINT ( 'NONE',  ( 4.623906867372411078, -13.21436662431711717, 21.42857142857142705 ) ) ;
#8305=CARTESIAN_POINT ( 'NONE',  ( 8.512513224245308763, 13.54758718765259040, 1.285714285714285809 ) ) ;
#8306=CARTESIAN_POINT ( 'NONE',  ( -15.10213328493390961, 5.284464991282586510, 47.57142857142857650 ) ) ;
#8308=CARTESIAN_POINT ( 'NONE',  ( -13.91197093850538380, -1.567502665446387278, 11.14285714285714235 ) ) ;
#8310=CARTESIAN_POINT ( 'NONE',  ( 8.731428362939189114, -13.89598863503035986, 27.21428571428571885 ) ) ;
#8312=CARTESIAN_POINT ( 'NONE',  ( 13.89774397934249706, 1.693770420379375308, 4.138816573230708507 ) ) ;
#8316=CARTESIAN_POINT ( 'NONE',  ( -12.15899005565164792, 7.639999817571650809, 17.78571428571428825 ) ) ;
#8317=CARTESIAN_POINT ( 'NONE',  ( -9.989344678689363377, 9.809645194533960222, 25.99595943037356349 ) ) ;
#8322=CARTESIAN_POINT ( 'NONE',  ( -13.25633410266679313, 4.503970704919840529, 49.56738800180214355 ) ) ;
#8326=CARTESIAN_POINT ( 'NONE',  ( -13.59724543428031573, -4.619798703722008959, 32.93261199819787777 ) ) ;
#8328=CARTESIAN_POINT ( 'NONE',  ( 13.47998361472151529, 8.620103694222146729, 45.71024514465928235 ) ) ;
#8329=CARTESIAN_POINT ( 'NONE',  ( -13.20330265076414911, 7.287341860736131771, 48.72999999999998977 ) ) ;
#8331=CARTESIAN_POINT ( 'NONE',  ( 9.989344678689365153, -9.809645194533958446, 10.99595943037356882 ) ) ;
#8335=CARTESIAN_POINT ( 'NONE',  ( 12.15899005565164792, -7.639999817571655250, 38.78571428571429180 ) ) ;
#8336=CARTESIAN_POINT ( 'NONE',  ( 7.448449071214646722, 11.85413878919601594, 37.28571428571429180 ) ) ;
#8338=CARTESIAN_POINT ( 'NONE',  ( 1.791431617652837316, 15.89939535829188877, 48.85714285714286120 ) ) ;
#8339=CARTESIAN_POINT ( 'NONE',  ( -3.974304365018271223, 15.37125927611797493, 1.442806492371165318E-14 ) ) ;
#8340=CARTESIAN_POINT ( 'NONE',  ( 13.89598863503046111, -8.731428362939032795, 26.78571428571429536 ) ) ;
#8349=CARTESIAN_POINT ( 'NONE',  ( 13.61519076058348254, 8.404922754268771001, 11.71832628391215181 ) ) ;
#8350=CARTESIAN_POINT ( 'NONE',  ( -1.791431617652833763, -15.89939535829188877, 39.85714285714286120 ) ) ;
#8351=CARTESIAN_POINT ( 'NONE',  ( 13.61519076058348254, 8.404922754268771001, -0.2816737160878517443 ) ) ;
#8352=CARTESIAN_POINT ( 'NONE',  ( 13.55419868402807992, 4.742819248065648807, 19.92857142857143771 ) ) ;
#8353=CARTESIAN_POINT ( 'NONE',  ( 11.60466159355862104, 11.60466159355875071, 1.500000000000003553 ) ) ;
#8354=CARTESIAN_POINT ( 'NONE',  ( -8.731428362939189114, 13.89598863503036341, 48.21428571428570820 ) ) ;
#8358=CARTESIAN_POINT ( 'NONE',  ( -5.284464991282755264, 15.10213328493384743, 30.42857142857143060 ) ) ;
#8359=CARTESIAN_POINT ( 'NONE',  ( 10.06191849875406064, 10.24623928997363187, 3.495959430373559940 ) ) ;
#8361=PRODUCT_CONTEXT ( 'NONE', #8904, 'mechanical' ) ;
#8362=CARTESIAN_POINT ( 'NONE',  ( -7.639999817571786700, 12.15899005565156266, 30.21428571428572241 ) ) ;
#8363=CARTESIAN_POINT ( 'NONE',  ( 9.989344678689365153, -9.809645194533958446, 22.99595943037356705 ) ) ;
#8374=CARTESIAN_POINT ( 'NONE',  ( 13.17239914596754424, -4.743843029824685864, 24.57546914105500946 ) ) ;
#8377=CARTESIAN_POINT ( 'NONE',  ( 13.96533075980324234, -8.621071003556521006, 34.78167371608785885 ) ) ;
#8378=CARTESIAN_POINT ( 'NONE',  ( -13.10821530951307778, 7.834963172504977535, 48.73000000000001108 ) ) ;
#8380=CARTESIAN_POINT ( 'NONE',  ( -1.737328882695368115, 14.25515036105620581, 20.63881657323070939 ) ) ;
#8385=CARTESIAN_POINT ( 'NONE',  ( -11.85413878919593422, -7.448449071214776396, 40.71428571428571530 ) ) ;
#8386=CARTESIAN_POINT ( 'NONE',  ( -13.92619789766827054, -1.441234910513399470, 3.146897712483577969 ) ) ;
#8388=CARTESIAN_POINT ( 'NONE',  ( 13.54758718765249803, 8.512513224245457977, 43.71428571428572241 ) ) ;
#8389=CARTESIAN_POINT ( 'NONE',  ( -1.045875314801341771, 15.69722212429930330, -1.227588689168360484E-16 ) ) ;
#8390=CARTESIAN_POINT ( 'NONE',  ( -15.89939535829186923, -1.791431617653016062, 35.14285714285713880 ) ) ;
#8396=CARTESIAN_POINT ( 'NONE',  ( 15.10213328493390783, -5.284464991282587398, 38.57142857142857650 ) ) ;
#8398=CARTESIAN_POINT ( 'NONE',  ( 8.621071003556677326, -13.96533075980314287, 25.21832628391215181 ) ) ;
#8399=CARTESIAN_POINT ( 'NONE',  ( -4.742819248065502258, -13.55419868402813677, 22.07142857142858006 ) ) ;
#8400=CARTESIAN_POINT ( 'NONE',  ( 1.791431617652837316, 15.89939535829188877, 0.8571428571428549859 ) ) ;
#8401=CARTESIAN_POINT ( 'NONE',  ( 11.60466159355862104, 11.60466159355875071, 43.50000000000000711 ) ) ;
#8406=CARTESIAN_POINT ( 'NONE',  ( 11.60466159355861926, 11.60466159355874716, 43.50000000000000711 ) ) ;
#8407=CARTESIAN_POINT ( 'NONE',  ( -11.78653521626494793, -7.556039541191465148, 6.710245144659284122 ) ) ;
#8409=CARTESIAN_POINT ( 'NONE',  ( 15.89939535829187278, 1.791431617653015174, 2.142857142857140573 ) ) ;
#8411=CARTESIAN_POINT ( 'NONE',  ( 15.49051278174638036, 5.420364854932175014, 7.928571428571430602 ) ) ;
#8412=CARTESIAN_POINT ( 'NONE',  ( -7.448449071214644945, -11.85413878919601771, 22.28571428571428470 ) ) ;
#8414=CARTESIAN_POINT ( 'NONE',  ( -13.51115193377584589, -4.865839792409295761, 42.92453085894499054 ) ) ;
#8418=CARTESIAN_POINT ( 'NONE',  ( 16.32287076676382043, -1.707986654103810897, 28.35310228751642825 ) ) ;
#8430=CARTESIAN_POINT ( 'NONE',  ( 1.967016585148662289, -16.29368510291087091, 47.63881657323071295 ) ) ;
#8432=CARTESIAN_POINT ( 'NONE',  ( -5.420364854931999155, -15.49051278174644253, 28.07142857142857295 ) ) ;
#8437=CARTESIAN_POINT ( 'NONE',  ( -4.743843029824828861, 13.17239914596749450, 20.42453085894499054 ) ) ;
#8441=CARTESIAN_POINT ( 'NONE',  ( -10.15407889436378852, -10.15407889436390576, 40.50000000000000711 ) ) ;
#8442=CARTESIAN_POINT ( 'NONE',  ( 13.59724543428031573, 4.619798703722006294, 5.932611998197868886 ) ) ;
#8444=CARTESIAN_POINT ( 'NONE',  ( -16.32287076676382398, 1.707986654103809343, 7.353102287516419366 ) ) ;
#8446=CARTESIAN_POINT ( 'NONE',  ( 11.60466159355862104, 11.60466159355875071, 25.50000000000000711 ) ) ;
#8454=CARTESIAN_POINT ( 'NONE',  ( 5.420364854932001819, 15.49051278174644430, 49.07142857142859071 ) ) ;
#8457=CARTESIAN_POINT ( 'NONE',  ( -1.707986654103994528, 16.32287076676380266, 16.64689771248358596 ) ) ;
#8458=CARTESIAN_POINT ( 'NONE',  ( 1.567502665446232957, 13.91197093850540156, 30.85714285714286120 ) ) ;
#8459=CARTESIAN_POINT ( 'NONE',  ( -8.512513224245306986, -13.54758718765259218, 4.285714285714288252 ) ) ;
#8460=CARTESIAN_POINT ( 'NONE',  ( -1.791431617652833763, -15.89939535829188877, 45.85714285714286120 ) ) ;
#8464=CARTESIAN_POINT ( 'NONE',  ( -15.10213328493390961, 5.284464991282586510, 47.57142857142857650 ) ) ;
#8466=CARTESIAN_POINT ( 'NONE',  ( 10.06191849875406064, 10.24623928997363187, 9.495959430373563492 ) ) ;
#8468=CARTESIAN_POINT ( 'NONE',  ( 11.60466159355862104, 11.60466159355875071, 1.500000000000003553 ) ) ;
#8469=CARTESIAN_POINT ( 'NONE',  ( 13.54758718765249803, 8.512513224245457977, 1.714285714285716855 ) ) ;
#8471=CARTESIAN_POINT ( 'NONE',  ( -11.85413878919593422, -7.448449071214776396, 22.71428571428571530 ) ) ;
#8472=CARTESIAN_POINT ( 'NONE',  ( -10.24623928997352351, -10.06191849875416899, 20.50404056962644006 ) ) ;
#8475=CARTESIAN_POINT ( 'NONE',  ( -4.743843029824828861, 13.17239914596749450, 38.42453085894499054 ) ) ;
#8477=CARTESIAN_POINT ( 'NONE',  ( -13.96533075980324234, 8.621071003556515677, 25.78167371608785530 ) ) ;
#8481=CARTESIAN_POINT ( 'NONE',  ( 7.448449071214646722, 11.85413878919601594, 1.285714285714285809 ) ) ;
#8485=CARTESIAN_POINT ( 'NONE',  ( -10.24623928997352351, -10.06191849875416899, 26.50404056962643651 ) ) ;
#8487=CARTESIAN_POINT ( 'NONE',  ( 4.743843029824831525, -13.17239914596749095, 5.424530858944991429 ) ) ;
#8489=CARTESIAN_POINT ( 'NONE',  ( -11.60466159355861926, -11.60466159355875249, 28.50000000000001066 ) ) ;
#8491=CARTESIAN_POINT ( 'NONE',  ( 14.28433602490915000, -1.478298951650544479, 16.35310228751641759 ) ) ;
#8495=CARTESIAN_POINT ( 'NONE',  ( 7.448449071214646722, 11.85413878919601594, 43.28571428571429180 ) ) ;
#8496=CARTESIAN_POINT ( 'NONE',  ( -1.478298951650703019, 14.28433602490913579, -1.353102287516420921 ) ) ;
#8498=CARTESIAN_POINT ( 'NONE',  ( -1.967016585148659846, 16.29368510291087091, 8.638816573230704066 ) ) ;
#8500=CARTESIAN_POINT ( 'NONE',  ( -5.284464991282755264, 15.10213328493384743, 30.42857142857143060 ) ) ;
#8507=CARTESIAN_POINT ( 'NONE',  ( 11.31370849898469899, 11.31370849898481978, 49.50000000000000711 ) ) ;
#8509=CARTESIAN_POINT ( 'NONE',  ( -16.29368510291090288, 1.967016585148476215, 21.36118342676929771 ) ) ;
#8510=CARTESIAN_POINT ( 'NONE',  ( 5.284464991282756152, -15.10213328493384743, 21.42857142857142705 ) ) ;
#8515=CARTESIAN_POINT ( 'NONE',  ( 15.89939535829187278, 1.791431617653015174, 44.14285714285714590 ) ) ;
#8516=SHAPE_REPRESENTATION_RELATIONSHIP ( 'NONE' , 'NONE' ,  #3956, #939 ) ;
#8519=CARTESIAN_POINT ( 'NONE',  ( 15.49051278174638036, 5.420364854932175014, 1.928571428571430380 ) ) ;
#8520=CARTESIAN_POINT ( 'NONE',  ( -1.837501619626328297, 16.30827793483733856, 0.6428571428571432378 ) ) ;
#8522=CARTESIAN_POINT ( 'NONE',  ( 13.55419868402807992, 4.742819248065649695, 19.92857142857143415 ) ) ;
#8524=CARTESIAN_POINT ( 'NONE',  ( -14.28433602490915000, 1.478298951650542481, 43.35310228751642825 ) ) ;
#8527=CARTESIAN_POINT ( 'NONE',  ( -13.96533075980324234, 8.621071003556515677, 19.78167371608784819 ) ) ;
#8528=CARTESIAN_POINT ( 'NONE',  ( 1.837501619626329630, -16.30827793483733501, 3.642857142857143238 ) ) ;
#8530=CARTESIAN_POINT ( 'NONE',  ( 13.96533075980324234, -8.621071003556521006, 22.78167371608784464 ) ) ;
#8534=CARTESIAN_POINT ( 'NONE',  ( -8.621071003556675549, 13.96533075980314642, -1.781673716087850634 ) ) ;
#8537=CARTESIAN_POINT ( 'NONE',  ( 1.737328882695370558, -14.25515036105620581, 5.638816573230711171 ) ) ;
#8539=CARTESIAN_POINT ( 'NONE',  ( -1.837501619626328297, 16.30827793483733856, 30.64285714285715301 ) ) ;
#8546=CARTESIAN_POINT ( 'NONE',  ( -12.15899005565164792, 7.639999817571651697, 41.78571428571430602 ) ) ;
#8547=CARTESIAN_POINT ( 'NONE',  ( -14.25515036105622890, 1.737328882695209575, 3.361183426769288385 ) ) ;
#8549=CARTESIAN_POINT ( 'NONE',  ( 5.404401153735178376, -15.06016580658422477, 11.42453085894499587 ) ) ;
#8551=CARTESIAN_POINT ( 'NONE',  ( -15.49051278174638036, -5.420364854932175902, 34.92857142857145192 ) ) ;
#8557=CARTESIAN_POINT ( 'NONE',  ( -1.837501619626328297, 16.30827793483733856, 42.64285714285715301 ) ) ;
#8559=CARTESIAN_POINT ( 'NONE',  ( -11.69682198916834892, -11.51250119794901394, 14.50404056962643651 ) ) ;
#8560=CARTESIAN_POINT ( 'NONE',  ( -15.49051278174638036, -5.420364854932175902, 16.92857142857143771 ) ) ;
#8564=CARTESIAN_POINT ( 'NONE',  ( -15.89939535829186923, -1.791431617653016062, 47.14285714285714590 ) ) ;
#8568=CARTESIAN_POINT ( 'NONE',  ( 13.54758718765249803, 8.512513224245457977, 7.714285714285715301 ) ) ;
#8569=CARTESIAN_POINT ( 'NONE',  ( -13.82664651025767100, 8.841785722321537477, 45.78975485534073897 ) ) ;
#8571=CARTESIAN_POINT ( 'NONE',  ( 1.607813917173037899, -14.26974319298267169, 27.64285714285714590 ) ) ;
#8574=CARTESIAN_POINT ( 'NONE',  ( -9.989344678689363377, 9.809645194533960222, 37.99595943037355994 ) ) ;
#8576=DIRECTION ( 'NONE',  ( -0.7056782240951883223, -0.7056782240951970930, -0.06353336191096711771 ) ) ;
#8577=CARTESIAN_POINT ( 'NONE',  ( -8.404922754268618235, -13.61519076058357491, 24.28167371608785530 ) ) ;
#8578=CARTESIAN_POINT ( 'NONE',  ( 15.10213328493390783, -5.284464991282587398, 8.571428571428569398 ) ) ;
#8580=CARTESIAN_POINT ( 'NONE',  ( -1.967016585148659846, 16.29368510291087091, 26.63881657323070939 ) ) ;
#8587=CARTESIAN_POINT ( 'NONE',  ( 4.619798703721856192, 13.59724543428036725, 9.067388001802141773 ) ) ;
#8590=CARTESIAN_POINT ( 'NONE',  ( 13.54758718765249803, 8.512513224245457977, 25.71428571428571885 ) ) ;
#8597=CARTESIAN_POINT ( 'NONE',  ( 1.917699372585825790, 15.88516839912900203, 46.86118342676930126 ) ) ;
#8598=CARTESIAN_POINT ( 'NONE',  ( 4.865839792409144771, 13.51115193377589740, 11.07546914105500768 ) ) ;
#8599=CARTESIAN_POINT ( 'NONE',  ( 14.25515036105622535, -1.737328882695210241, 0.3611834267692887734 ) ) ;
#8601=CARTESIAN_POINT ( 'NONE',  ( 11.51250119794888249, 11.69682198916847682, 15.49595943037356882 ) ) ;
#8605=CARTESIAN_POINT ( 'NONE',  ( -1.837501619626328297, 16.30827793483733856, 42.64285714285715301 ) ) ;
#8606=LINE ( 'NONE', #7153, #5631 ) ;
#8612=CARTESIAN_POINT ( 'NONE',  ( 8.621071003556677326, -13.96533075980314287, 19.21832628391215181 ) ) ;
#8615=CARTESIAN_POINT ( 'NONE',  ( -1.917699372585823570, -15.88516839912900558, 13.86118342676929416 ) ) ;
#8616=CARTESIAN_POINT ( 'NONE',  ( -5.284464991282755264, 15.10213328493384743, 12.42857142857142705 ) ) ;
#8619=CARTESIAN_POINT ( 'NONE',  ( 11.31370849898482334, -11.31370849898469366, 3.000000000000002665 ) ) ;
#8621=CARTESIAN_POINT ( 'NONE',  ( -11.60466159355861748, -11.60466159355874893, 46.50000000000001421 ) ) ;
#8625=CARTESIAN_POINT ( 'NONE',  ( -15.89939535829186923, -1.791431617653016062, 5.142857142857143238 ) ) ;
#8626=CARTESIAN_POINT ( 'NONE',  ( 13.89598863503046111, -8.731428362939032795, 2.785714285714284255 ) ) ;
#8628=CARTESIAN_POINT ( 'NONE',  ( 9.899494936611718643, -9.899494936611608509, 45.00000000000000711 ) ) ;
#8632=CARTESIAN_POINT ( 'NONE',  ( 13.91197093850538380, 1.567502665446386390, 8.142857142857145902 ) ) ;
#8635=CARTESIAN_POINT ( 'NONE',  ( -16.32287076676382398, 1.707986654103809343, 19.35310228751642825 ) ) ;
#8638=CARTESIAN_POINT ( 'NONE',  ( 11.51250119794888249, 11.69682198916847682, 21.49595943037356705 ) ) ;
#8642=CARTESIAN_POINT ( 'NONE',  ( 12.15899005565164792, -7.639999817571654361, 2.785714285714283367 ) ) ;
#8644=CARTESIAN_POINT ( 'NONE',  ( -11.51250119794888072, -11.69682198916848037, 48.49595943037355994 ) ) ;
#8647=CARTESIAN_POINT ( 'NONE',  ( 1.737328882695370558, -14.25515036105620581, 23.63881657323070939 ) ) ;
#8651=CARTESIAN_POINT ( 'NONE',  ( -1.478298951650703019, 14.28433602490913579, 10.64689771248357886 ) ) ;
#8653=CARTESIAN_POINT ( 'NONE',  ( -7.529642458189277576, 12.22833218042435455, 16.21832628391214470 ) ) ;
#8655=CARTESIAN_POINT ( 'NONE',  ( 15.88516839912898071, 1.917699372586004092, 10.13881657323070762 ) ) ;
#8657=CARTESIAN_POINT ( 'NONE',  ( -15.49051278174638036, -5.420364854932175902, 46.92857142857142350 ) ) ;
#8663=CARTESIAN_POINT ( 'NONE',  ( -11.69682198916834892, -11.51250119794901394, 32.50404056962644006 ) ) ;
#8665=CARTESIAN_POINT ( 'NONE',  ( -13.61519076058348254, -8.404922754268771001, 32.71832628391215536 ) ) ;
#8666=CARTESIAN_POINT ( 'NONE',  ( -11.60466159355861926, -11.60466159355875249, 16.50000000000000000 ) ) ;
#8675=CARTESIAN_POINT ( 'NONE',  ( -7.556039541191334585, -11.78653521626503320, 44.28975485534073186 ) ) ;
#8676=CARTESIAN_POINT ( 'NONE',  ( 5.420364854932001819, 15.49051278174644430, 13.07142857142857295 ) ) ;
#8677=CARTESIAN_POINT ( 'NONE',  ( 12.15899005565164792, -7.639999817571654361, 38.78571428571429180 ) ) ;
#8681=CARTESIAN_POINT ( 'NONE',  ( 1.607813917173038121, -14.26974319298267346, 9.642857142857147679 ) ) ;
#8683=CARTESIAN_POINT ( 'NONE',  ( -13.47998361472151174, -8.620103694222146729, 30.71024514465928235 ) ) ;
#8684=CARTESIAN_POINT ( 'NONE',  ( 13.54758718765249803, 8.512513224245457977, 19.71428571428571175 ) ) ;
#8685=CARTESIAN_POINT ( 'NONE',  ( -5.404401153735176599, 15.06016580658422477, 26.42453085894499765 ) ) ;
#8689=SURFACE_SIDE_STYLE ('',( #4810 ) ) ;
#8691=CARTESIAN_POINT ( 'NONE',  ( -11.78653521626494793, -7.556039541191465148, 18.71024514465927879 ) ) ;
#8695=CARTESIAN_POINT ( 'NONE',  ( 13.51115193377584589, 4.865839792409294873, 27.92453085894499054 ) ) ;
#8700=CARTESIAN_POINT ( 'NONE',  ( 10.24623928997352884, 10.06191849875416899, 11.50404056962644006 ) ) ;
#8701=CARTESIAN_POINT ( 'NONE',  ( 7.529642458189280241, -12.22833218042435099, 19.21832628391215181 ) ) ;
#8704=CARTESIAN_POINT ( 'NONE',  ( 8.512513224245308763, 13.54758718765259040, 49.28571428571428470 ) ) ;
#8710=CARTESIAN_POINT ( 'NONE',  ( 15.06016580658428694, -5.404401153735007846, 24.57546914105500946 ) ) ;
#8712=CARTESIAN_POINT ( 'NONE',  ( -1.707986654103994528, 16.32287076676380266, 34.64689771248358596 ) ) ;
#8714=CARTESIAN_POINT ( 'NONE',  ( 15.10213328493390783, -5.284464991282587398, 26.57142857142857295 ) ) ;
#8715=CARTESIAN_POINT ( 'NONE',  ( 0.7290266316634184118, 15.99096059591463614, 48.73000000000001108 ) ) ;
#8716=CARTESIAN_POINT ( 'NONE',  ( 15.89939535829187278, 1.791431617653015174, 2.142857142857140573 ) ) ;
#8718=SURFACE_STYLE_FILL_AREA ( #5558 ) ;
#8722=CARTESIAN_POINT ( 'NONE',  ( 7.529642458189280241, -12.22833218042435099, 43.21832628391217668 ) ) ;
#8723=CARTESIAN_POINT ( 'NONE',  ( -8.512513224245306986, -13.54758718765259218, 10.28571428571428648 ) ) ;
#8725=CARTESIAN_POINT ( 'NONE',  ( -13.55419868402807992, -4.742819248065651472, 40.92857142857143771 ) ) ;
#8726=CARTESIAN_POINT ( 'NONE',  ( 13.17239914596754424, -4.743843029824685864, 42.57546914105501656 ) ) ;
#8727=CARTESIAN_POINT ( 'NONE',  ( -11.92174236212692051, -7.340858601238089420, 32.71832628391215536 ) ) ;
#8731=CARTESIAN_POINT ( 'NONE',  ( 9.899494936611718643, -9.899494936611608509, 3.000000000000002665 ) ) ;
#8734=CARTESIAN_POINT ( 'NONE',  ( 11.31370849898482334, -11.31370849898469366, 21.00000000000000355 ) ) ;
#8735=CARTESIAN_POINT ( 'NONE',  ( -11.40355824106246807, 11.22385875690704715, 25.99595943037356349 ) ) ;
#8738=CARTESIAN_POINT ( 'NONE',  ( -4.623906867372410190, 13.21436662431711895, 0.4285714285714309346 ) ) ;
#8741=CARTESIAN_POINT ( 'NONE',  ( 12.22833218042443271, -7.529642458189144349, 10.78167371608784819 ) ) ;
#8743=CARTESIAN_POINT ( 'NONE',  ( 8.731428362939190890, -13.89598863503036164, 15.21428571428571530 ) ) ;
#8748=CARTESIAN_POINT ( 'NONE',  ( 14.25515036105622535, -1.737328882695210241, 6.361183426769297711 ) ) ;
#8750=CARTESIAN_POINT ( 'NONE',  ( -11.92174236212692051, -7.340858601238089420, 14.71832628391215003 ) ) ;
#8753=CARTESIAN_POINT ( 'NONE',  ( -11.60466159355861926, -11.60466159355875249, 40.50000000000000711 ) ) ;
#8760=CARTESIAN_POINT ( 'NONE',  ( 16.29368510291089223, -1.967016585148476882, 24.36118342676929416 ) ) ;
#8762=CARTESIAN_POINT ( 'NONE',  ( 13.61519076058348254, 8.404922754268771001, 29.71832628391214826 ) ) ;
#8766=ORIENTED_EDGE ( 'NONE', *, *, #6657, .F. ) ;
#8767=CARTESIAN_POINT ( 'NONE',  ( 1.791431617652837316, 15.89939535829188877, 36.85714285714286120 ) ) ;
#8768=CARTESIAN_POINT ( 'NONE',  ( 3.924309341735328527, 14.50897616450780170, 2.434022981070398477E-13 ) ) ;
#8772=( LENGTH_UNIT ( ) NAMED_UNIT ( * ) SI_UNIT ( .MILLI., .METRE. ) );
#8780=CARTESIAN_POINT ( 'NONE',  ( -11.69682198916834892, -11.51250119794901394, 2.504040569626438728 ) ) ;
#8781=CARTESIAN_POINT ( 'NONE',  ( -15.89939535829186923, -1.791431617653016062, 11.14285714285714235 ) ) ;
#8782=CARTESIAN_POINT ( 'NONE',  ( 1.567502665446232957, 13.91197093850540156, 42.85714285714285410 ) ) ;
#8783=CARTESIAN_POINT ( 'NONE',  ( -14.25515036105622890, 1.737328882695209575, 39.36118342676930837 ) ) ;
#8784=CARTESIAN_POINT ( 'NONE',  ( 7.639999817571789364, -12.15899005565156266, 9.214285714285717077 ) ) ;
#8789=CARTESIAN_POINT ( 'NONE',  ( -1.607813917173034124, 14.26974319298267524, 6.642857142857143238 ) ) ;
#8791=CARTESIAN_POINT ( 'NONE',  ( -13.89598863503045933, 8.731428362939027465, 17.78571428571428825 ) ) ;
#8792=CARTESIAN_POINT ( 'NONE',  ( 13.96533075980324234, -8.621071003556521006, 40.78167371608785885 ) ) ;
#8799=CARTESIAN_POINT ( 'NONE',  ( 10.06191849875406064, 10.24623928997363187, 15.49595943037356882 ) ) ;
#8803=CARTESIAN_POINT ( 'NONE',  ( -1.837501619626328297, 16.30827793483733856, 36.64285714285714590 ) ) ;
#8804=CARTESIAN_POINT ( 'NONE',  ( 4.619798703721856192, 13.59724543428036725, 45.06738800180215065 ) ) ;
#8809=CARTESIAN_POINT ( 'NONE',  ( 13.59724543428031573, 4.619798703722006294, 5.932611998197868886 ) ) ;
#8812=CARTESIAN_POINT ( 'NONE',  ( 14.25515036105622535, -1.737328882695210241, 6.361183426769297711 ) ) ;
#8815=CARTESIAN_POINT ( 'NONE',  ( 5.404401153735178376, -15.06016580658422477, 11.42453085894499587 ) ) ;
#8821=CARTESIAN_POINT ( 'NONE',  ( -15.91362231745475597, -1.665163862720028254, 27.14689771248358241 ) ) ;
#8823=CARTESIAN_POINT ( 'NONE',  ( -15.06016580658428694, 5.404401153735006957, 27.57546914105500946 ) ) ;
#8825=CARTESIAN_POINT ( 'NONE',  ( 15.49051278174638036, 5.420364854932175014, 31.92857142857143415 ) ) ;
#8826=CARTESIAN_POINT ( 'NONE',  ( 3.654384819347590962, 14.75870095501612944, 2.020632658447807793E-13 ) ) ;
#8827=CARTESIAN_POINT ( 'NONE',  ( 1.791431617652837316, 15.89939535829188877, 6.857142857142860315 ) ) ;
#8829=CARTESIAN_POINT ( 'NONE',  ( 10.19143222367002366, 10.12210786732603474, 48.73000000000001819 ) ) ;
#8832=CARTESIAN_POINT ( 'NONE',  ( -7.529642458189277576, 12.22833218042435455, 46.21832628391216247 ) ) ;
#8833=CARTESIAN_POINT ( 'NONE',  ( 13.89598863503046111, -8.731428362939032795, 14.78571428571429358 ) ) ;
#8834=CARTESIAN_POINT ( 'NONE',  ( -7.639999817571786700, 12.15899005565156266, 42.21428571428571530 ) ) ;
#8835=CARTESIAN_POINT ( 'NONE',  ( 14.25515036105622535, -1.737328882695210241, 42.36118342676930126 ) ) ;
#8836=CARTESIAN_POINT ( 'NONE',  ( 14.26974319298268767, -1.607813917172876916, 14.35714285714285587 ) ) ;
#8840=CARTESIAN_POINT ( 'NONE',  ( 4.742819248065503146, 13.55419868402813677, 1.071428571428570287 ) ) ;
#8844=CARTESIAN_POINT ( 'NONE',  ( -13.54758718765249625, -8.512513224245459753, 16.71428571428571530 ) ) ;
#8846=CARTESIAN_POINT ( 'NONE',  ( -16.32287076676382398, 1.707986654103809343, 37.35310228751641404 ) ) ;
#8849=CARTESIAN_POINT ( 'NONE',  ( 7.448449071214646722, 11.85413878919601594, 1.285714285714285809 ) ) ;
#8851=CARTESIAN_POINT ( 'NONE',  ( 13.25633410266679313, -4.503970704919842305, 10.56738800180213644 ) ) ;
#8854=CARTESIAN_POINT ( 'NONE',  ( 1.737328882695370558, -14.25515036105620581, 35.63881657323071295 ) ) ;
#8858=CARTESIAN_POINT ( 'NONE',  ( 4.865839792409144771, 13.51115193377589740, 23.07546914105501301 ) ) ;
#8861=CARTESIAN_POINT ( 'NONE',  ( -15.88516839912898071, -1.917699372586004980, 13.13881657323070584 ) ) ;
#8867=CARTESIAN_POINT ( 'NONE',  ( 9.899494936611718643, -9.899494936611608509, 33.00000000000000000 ) ) ;
#8868=CARTESIAN_POINT ( 'NONE',  ( -11.69682198916834892, -11.51250119794901394, 32.50404056962644006 ) ) ;
#8871=CARTESIAN_POINT ( 'NONE',  ( 1.837501619626330074, -16.30827793483733501, 33.64285714285715301 ) ) ;
#8873=CARTESIAN_POINT ( 'NONE',  ( -15.10213328493390961, 5.284464991282586510, 17.57142857142856940 ) ) ;
#8876=CARTESIAN_POINT ( 'NONE',  ( 13.89598863503046111, -8.731428362939032795, 38.78571428571429180 ) ) ;
#8878=UNCERTAINTY_MEASURE_WITH_UNIT (LENGTH_MEASURE( 1.000000000000000082E-05 ), #8772, 'distance_accuracy_value', 'NONE');
#8879=CARTESIAN_POINT ( 'NONE',  ( -10.24623928997352351, -10.06191849875416899, 44.50404056962644006 ) ) ;
#8880=CARTESIAN_POINT ( 'NONE',  ( -5.284464991282755264, 15.10213328493384743, 18.42857142857143415 ) ) ;
#8881=CARTESIAN_POINT ( 'NONE',  ( 11.92174236212692229, 7.340858601238088532, 35.71832628391214115 ) ) ;
#8882=CARTESIAN_POINT ( 'NONE',  ( -7.448449071214644945, -11.85413878919601771, 4.285714285714288252 ) ) ;
#8886=CARTESIAN_POINT ( 'NONE',  ( -7.448449071214644945, -11.85413878919601771, 16.28571428571428470 ) ) ;
#8888=DIRECTION ( 'NONE',  ( 0.7056782240951884333, 0.7056782240951970930, 0.06353336191096713159 ) ) ;
#8890=CARTESIAN_POINT ( 'NONE',  ( 15.10213328493390783, -5.284464991282587398, 20.57142857142857295 ) ) ;
#8891=CARTESIAN_POINT ( 'NONE',  ( 5.297344310588354865, 15.53355953199867301, 33.06738800180213644 ) ) ;
#8894=CARTESIAN_POINT ( 'NONE',  ( -1.567502665446231180, -13.91197093850540334, 15.85714285714286120 ) ) ;
#8899=CARTESIAN_POINT ( 'NONE',  ( 10.06191849875406064, 10.24623928997363187, 39.49595943037357415 ) ) ;
#8903=CARTESIAN_POINT ( 'NONE',  ( 1.693770420379222319, 13.89774397934251837, 16.86118342676929061 ) ) ;
#8904=APPLICATION_CONTEXT ( 'automotive_design' ) ;
#8905=CARTESIAN_POINT ( 'NONE',  ( 4.503970704919991519, -13.25633410266674517, 19.43261199819785645 ) ) ;
#8908=CARTESIAN_POINT ( 'NONE',  ( 13.96533075980324234, -8.621071003556521006, 4.781673716087850856 ) ) ;
#8914=CARTESIAN_POINT ( 'NONE',  ( -7.448449071214644945, -11.85413878919601771, 34.28571428571428470 ) ) ;
#8915=CARTESIAN_POINT ( 'NONE',  ( 11.22385875690717683, -11.40355824106234373, 43.00404056962644717 ) ) ;
#8918=CARTESIAN_POINT ( 'NONE',  ( 11.60466159355862104, 11.60466159355875071, 31.50000000000001421 ) ) ;
#8919=CARTESIAN_POINT ( 'NONE',  ( 3.856535827843035946, 14.61332904867485816, 3.589645083303631449E-17 ) ) ;
#8920=CARTESIAN_POINT ( 'NONE',  ( 8.512513224245308763, 13.54758718765259040, 19.28571428571428825 ) ) ;
#8925=CARTESIAN_POINT ( 'NONE',  ( -1.707986654103994528, 16.32287076676380266, 10.64689771248357886 ) ) ;
#8927=CARTESIAN_POINT ( 'NONE',  ( -8.512513224245306986, -13.54758718765259218, 28.28571428571428825 ) ) ;
#8930=DIRECTION ( 'NONE',  ( 0.000000000000000000, 0.000000000000000000, 1.000000000000000000 ) ) ;
#8931=CARTESIAN_POINT ( 'NONE',  ( 15.53355953199861794, 5.297344310588528060, -0.06738800180213055935 ) ) ;
#8932=CARTESIAN_POINT ( 'NONE',  ( 15.10213328493390783, -5.284464991282587398, 38.57142857142857650 ) ) ;
#8933=CARTESIAN_POINT ( 'NONE',  ( 4.623906867372411078, -13.21436662431711717, 15.42857142857143060 ) ) ;
#8937=CARTESIAN_POINT ( 'NONE',  ( -10.15407889436378852, -10.15407889436390576, 16.50000000000000000 ) ) ;
#8943=CARTESIAN_POINT ( 'NONE',  ( 15.49051278174637858, 5.420364854932174126, 25.92857142857143060 ) ) ;
#8944=CARTESIAN_POINT ( 'NONE',  ( -5.404401153735176599, 15.06016580658422477, 32.42453085894499054 ) ) ;
#8947=CARTESIAN_POINT ( 'NONE',  ( 10.15407889436379030, 10.15407889436390221, 13.50000000000000355 ) ) ;
#8949=CARTESIAN_POINT ( 'NONE',  ( 1.441234910513245149, 13.92619789766829008, 26.85310228751642470 ) ) ;
#8954=CARTESIAN_POINT ( 'NONE',  ( -13.51115193377584589, -4.865839792409295761, 42.92453085894499054 ) ) ;
#8960=CARTESIAN_POINT ( 'NONE',  ( 9.809645194534072132, -9.989344678689256796, 19.00404056962642940 ) ) ;
#8962=CARTESIAN_POINT ( 'NONE',  ( -13.92619789766827054, -1.441234910513399470, 21.14689771248358241 ) ) ;
#8964=CARTESIAN_POINT ( 'NONE',  ( 1.665163862719847732, 15.91362231745477374, 44.85310228751641404 ) ) ;
#8967=CARTESIAN_POINT ( 'NONE',  ( -1.967016585148659846, 16.29368510291087091, 8.638816573230704066 ) ) ;
#8975=CARTESIAN_POINT ( 'NONE',  ( -16.29368510291090288, 1.967016585148476215, 39.36118342676930837 ) ) ;
#8976=CARTESIAN_POINT ( 'NONE',  ( -4.623906867372410190, 13.21436662431711895, 30.42857142857143060 ) ) ;
#8977=CARTESIAN_POINT ( 'NONE',  ( -12.15899005565164792, 7.639999817571651697, 35.78571428571429180 ) ) ;
#8979=CARTESIAN_POINT ( 'NONE',  ( -15.49051278174638036, -5.420364854932175902, 46.92857142857142350 ) ) ;
#8980=CARTESIAN_POINT ( 'NONE',  ( 3.732286808396943822, 14.38075913893019653, -9.697396257098258182E-17 ) ) ;
#8981=CARTESIAN_POINT ( 'NONE',  ( 15.89939535829187278, 1.791431617653015174, 20.14285714285714235 ) ) ;
#8985=CARTESIAN_POINT ( 'NONE',  ( 8.620103694221997515, 13.47998361472160767, 5.289754855340725648 ) ) ;
#8986=CARTESIAN_POINT ( 'NONE',  ( 15.89939535829187278, 1.791431617653015174, 32.14285714285714590 ) ) ;
#8988=CARTESIAN_POINT ( 'NONE',  ( 11.69682198916835070, 11.51250119794901394, 5.504040569626439172 ) ) ;
#8989=CARTESIAN_POINT ( 'NONE',  ( -4.623906867372410190, 13.21436662431711895, 6.428571428571429713 ) ) ;
#8993=CARTESIAN_POINT ( 'NONE',  ( -13.21436662431716869, 4.623906867372262752, 11.57142857142857295 ) ) ;
#8997=CARTESIAN_POINT ( 'NONE',  ( 1.837501619626329630, -16.30827793483733501, 33.64285714285714590 ) ) ;
#8998=CARTESIAN_POINT ( 'NONE',  ( -5.404401153735176599, 15.06016580658422477, 50.42453085894499765 ) ) ;
#9000=CARTESIAN_POINT ( 'NONE',  ( 11.85413878919593422, 7.448449071214774619, 13.71428571428571352 ) ) ;
#9001=CARTESIAN_POINT ( 'NONE',  ( 12.22833218042443271, -7.529642458189144349, 28.78167371608785174 ) ) ;
#9003=CARTESIAN_POINT ( 'NONE',  ( 0.6500995950961804271, 14.01729557978340956, 48.73000000000002530 ) ) ;
#9004=CARTESIAN_POINT ( 'NONE',  ( -13.25633410266679313, 4.503970704919840529, 37.56738800180213644 ) ) ;
#9008=CARTESIAN_POINT ( 'NONE',  ( 7.529642458189280241, -12.22833218042435099, 13.21832628391215181 ) ) ;
#9011=CARTESIAN_POINT ( 'NONE',  ( -7.529642458189277576, 12.22833218042435455, 28.21832628391215181 ) ) ;
#9013=CARTESIAN_POINT ( 'NONE',  ( 15.44746603149413922, 5.543385399275817527, 39.92453085894499054 ) ) ;
#9015=CARTESIAN_POINT ( 'NONE',  ( 8.512513224245308763, 13.54758718765259040, 19.28571428571428825 ) ) ;
#9016=CARTESIAN_POINT ( 'NONE',  ( 15.88516839912898071, 1.917699372586004092, 10.13881657323070762 ) ) ;
#9022=CARTESIAN_POINT ( 'NONE',  ( -8.620103694221995738, -13.47998361472161299, 38.28975485534072476 ) ) ;
#9023=CARTESIAN_POINT ( 'NONE',  ( -11.85413878919593422, -7.448449071214776396, 34.71428571428571530 ) ) ;
#9025=CARTESIAN_POINT ( 'NONE',  ( -1.791431617652833763, -15.89939535829188877, 45.85714285714286120 ) ) ;
#9027=CARTESIAN_POINT ( 'NONE',  ( -11.31370849898482156, 11.31370849898469544, 11.99999999999999645 ) ) ;
#9031=CARTESIAN_POINT ( 'NONE',  ( -8.621071003556675549, 13.96533075980314642, 4.218326283912150032 ) ) ;
#9032=CARTESIAN_POINT ( 'NONE',  ( 11.31370849898482334, -11.31370849898469366, 27.00000000000000355 ) ) ;
#9034=CARTESIAN_POINT ( 'NONE',  ( -14.26974319298268767, 1.607813917172874696, 47.35714285714286120 ) ) ;
#9035=CARTESIAN_POINT ( 'NONE',  ( 5.543385399275644332, 15.44746603149420494, 5.075469141055008571 ) ) ;
#9036=CARTESIAN_POINT ( 'NONE',  ( 4.623906867372411078, -13.21436662431711717, 27.42857142857143060 ) ) ;
#9040=CARTESIAN_POINT ( 'NONE',  ( -13.55419868402807992, -4.742819248065651472, 10.92857142857142883 ) ) ;
#9043=CARTESIAN_POINT ( 'NONE',  ( -13.89598863503045933, 8.731428362939027465, 35.78571428571429180 ) ) ;
#9044=CARTESIAN_POINT ( 'NONE',  ( 4.619798703721856192, 13.59724543428036725, 3.067388001802140884 ) ) ;
#9047=CARTESIAN_POINT ( 'NONE',  ( -7.448449071214644945, -11.85413878919601771, 10.28571428571428648 ) ) ;
#9048=ORIENTED_EDGE ( 'NONE', *, *, #10187, .T. ) ;
#9049=CARTESIAN_POINT ( 'NONE',  ( -1.441234910513241818, -13.92619789766829008, 23.85310228751642825 ) ) ;
#9055=CARTESIAN_POINT ( 'NONE',  ( 10.15407889436379030, 10.15407889436390576, 1.500000000000003553 ) ) ;
#9060=CARTESIAN_POINT ( 'NONE',  ( -14.25515036105622890, 1.737328882695209575, 21.36118342676929771 ) ) ;
#9061=CARTESIAN_POINT ( 'NONE',  ( -13.92619789766827054, -1.441234910513399470, 27.14689771248358241 ) ) ;
#9063=CARTESIAN_POINT ( 'NONE',  ( -13.47998361472151174, -8.620103694222146729, 36.71024514465928235 ) ) ;
#9064=CARTESIAN_POINT ( 'NONE',  ( -4.874503691416085971, 13.19452956797008802, 48.73000000000003951 ) ) ;
#9065=CARTESIAN_POINT ( 'NONE',  ( -15.10213328493390961, 5.284464991282586510, 23.57142857142857650 ) ) ;
#9067=CARTESIAN_POINT ( 'NONE',  ( -13.89774397934249706, -1.693770420379375974, 19.13881657323070584 ) ) ;
#9071=CARTESIAN_POINT ( 'NONE',  ( -13.91197093850538380, -1.567502665446387278, 29.14285714285714235 ) ) ;
#9072=CARTESIAN_POINT ( 'NONE',  ( -7.639999817571787588, 12.15899005565156266, 36.21428571428573662 ) ) ;
#9074=CARTESIAN_POINT ( 'NONE',  ( -2.030095817397326030, 15.65302214768666467, 5.081489463560611418E-16 ) ) ;
#9075=CARTESIAN_POINT ( 'NONE',  ( 11.60466159355862104, 11.60466159355875071, 19.50000000000000355 ) ) ;
#9081=CARTESIAN_POINT ( 'NONE',  ( -15.06016580658428694, 5.404401153735006957, 3.575469141055005462 ) ) ;
#9082=CARTESIAN_POINT ( 'NONE',  ( -5.420364854931999155, -15.49051278174644253, 28.07142857142857295 ) ) ;
#9084=CARTESIAN_POINT ( 'NONE',  ( 8.620103694221997515, 13.47998361472160767, 5.289754855340725648 ) ) ;
#9086=CARTESIAN_POINT ( 'NONE',  ( -13.21436662431716869, 4.623906867372262752, 29.57142857142857650 ) ) ;
#9089=CARTESIAN_POINT ( 'NONE',  ( -11.85413878919593422, -7.448449071214776396, 16.71428571428571530 ) ) ;
#9091=CARTESIAN_POINT ( 'NONE',  ( 11.60466159355861926, 11.60466159355874716, 37.50000000000001421 ) ) ;
#9094=CARTESIAN_POINT ( 'NONE',  ( -15.44746603149413922, -5.543385399275820191, 48.92453085894499054 ) ) ;
#9097=CARTESIAN_POINT ( 'NONE',  ( -13.91197093850538380, -1.567502665446387278, 11.14285714285714235 ) ) ;
#9101=ORIENTED_EDGE ( 'NONE', *, *, #5165, .T. ) ;
#9102=CARTESIAN_POINT ( 'NONE',  ( 11.78653521626494793, 7.556039541191463371, 21.71024514465928235 ) ) ;
#9107=CARTESIAN_POINT ( 'NONE',  ( -9.899494936611716867, 9.899494936611610285, 0.000000000000000000 ) ) ;
#9111=CARTESIAN_POINT ( 'NONE',  ( 1.478298951650704351, -14.28433602490913579, 25.64689771248357886 ) ) ;
#9115=CARTESIAN_POINT ( 'NONE',  ( 13.47998361472151529, 8.620103694222146729, 39.71024514465927524 ) ) ;
#9117=CARTESIAN_POINT ( 'NONE',  ( -2.607279028132698961, 15.78019693191412287, 48.73000000000003951 ) ) ;
#9118=CARTESIAN_POINT ( 'NONE',  ( -11.60466159355861926, -11.60466159355875249, 22.50000000000000000 ) ) ;
#9122=CARTESIAN_POINT ( 'NONE',  ( 13.51115193377584589, 4.865839792409294873, 9.924530858944988765 ) ) ;
#9126=CARTESIAN_POINT ( 'NONE',  ( 11.22385875690717683, -11.40355824106234373, 37.00404056962644006 ) ) ;
#9127=CARTESIAN_POINT ( 'NONE',  ( 8.784089738577305795, 11.01490013464600892, 49.39149694378009769 ) ) ;
#9128=CARTESIAN_POINT ( 'NONE',  ( 4.623906867372411078, -13.21436662431711717, 39.42857142857143060 ) ) ;
#9130=CARTESIAN_POINT ( 'NONE',  ( -13.89598863503046111, 8.731428362939027465, 41.78571428571430602 ) ) ;
#9132=CARTESIAN_POINT ( 'NONE',  ( -8.512513224245306986, -13.54758718765259218, 28.28571428571428825 ) ) ;
#9133=PLANE ( 'NONE',  #369 ) ;
#9139=CARTESIAN_POINT ( 'NONE',  ( 15.91362231745475597, 1.665163862720026255, 12.14689771248358063 ) ) ;
#9140=CARTESIAN_POINT ( 'NONE',  ( 15.49051278174638036, 5.420364854932175014, 31.92857142857143415 ) ) ;
#9141=CARTESIAN_POINT ( 'NONE',  ( -1.917699372585823570, -15.88516839912900558, 1.861183426769295490 ) ) ;
#9143=CARTESIAN_POINT ( 'NONE',  ( 8.731428362939190890, -13.89598863503036164, 9.214285714285717077 ) ) ;
#9144=CARTESIAN_POINT ( 'NONE',  ( 15.89939535829187278, 1.791431617653015174, 44.14285714285714590 ) ) ;
#9148=CARTESIAN_POINT ( 'NONE',  ( -15.10213328493390961, 5.284464991282586510, 29.57142857142857650 ) ) ;
#9149=CARTESIAN_POINT ( 'NONE',  ( -11.40355824106246807, 11.22385875690704715, 49.99595943037357415 ) ) ;
#9151=PRODUCT ( 'main spring', 'main spring', '', ( #8361 ) ) ;
#9152=CARTESIAN_POINT ( 'NONE',  ( -11.85413878919593422, -7.448449071214776396, 28.71428571428571530 ) ) ;
#9153=CARTESIAN_POINT ( 'NONE',  ( -1.737328882695368115, 14.25515036105620581, 26.63881657323070939 ) ) ;
#9160=CARTESIAN_POINT ( 'NONE',  ( -14.28433602490915000, 1.478298951650542481, 49.35310228751642114 ) ) ;
#9164=CARTESIAN_POINT ( 'NONE',  ( -13.92619789766827054, -1.441234910513399470, 33.14689771248357886 ) ) ;
#9169=CARTESIAN_POINT ( 'NONE',  ( -13.06814903599441280, 7.205911594201809045, 48.73000000000001108 ) ) ;
#9170=CARTESIAN_POINT ( 'NONE',  ( 11.60466159355862104, 11.60466159355875071, 25.50000000000000711 ) ) ;
#9172=CARTESIAN_POINT ( 'NONE',  ( -12.22833218042443271, 7.529642458189139909, 13.78167371608785174 ) ) ;
#9176=CARTESIAN_POINT ( 'NONE',  ( 7.639999817571789364, -12.15899005565156266, 39.21428571428571530 ) ) ;
#9177=CARTESIAN_POINT ( 'NONE',  ( -7.639999817571787588, 12.15899005565156266, 42.21428571428572241 ) ) ;
#9179=CARTESIAN_POINT ( 'NONE',  ( -1.791431617652833763, -15.89939535829188877, 39.85714285714286120 ) ) ;
#9180=CARTESIAN_POINT ( 'NONE',  ( 0.5828906444166439549, 15.62646852646394713, 9.306676823330757431E-17 ) ) ;
#9181=CARTESIAN_POINT ( 'NONE',  ( -8.512513224245306986, -13.54758718765259218, 34.28571428571428470 ) ) ;
#9188=CARTESIAN_POINT ( 'NONE',  ( -15.91362231745475597, -1.665163862720028254, 21.14689771248358241 ) ) ;
#9189=CARTESIAN_POINT ( 'NONE',  ( -5.284464991282755264, 15.10213328493384743, 42.42857142857143060 ) ) ;
#9190=CARTESIAN_POINT ( 'NONE',  ( -13.61519076058348254, -8.404922754268771001, 20.71832628391214826 ) ) ;
#9191=CARTESIAN_POINT ( 'NONE',  ( -7.639999817571787588, 12.15899005565156266, 24.21428571428571530 ) ) ;
#9192=CARTESIAN_POINT ( 'NONE',  ( 13.54758718765249803, 8.512513224245457977, 1.714285714285716855 ) ) ;
#9193=CARTESIAN_POINT ( 'NONE',  ( -8.512513224245306986, -13.54758718765259218, 40.28571428571428470 ) ) ;
#9197=CARTESIAN_POINT ( 'NONE',  ( 5.284464991282756152, -15.10213328493384743, 39.42857142857143060 ) ) ;
#9198=CARTESIAN_POINT ( 'NONE',  ( -10.06191849875405531, -10.24623928997363542, 6.495959430373559051 ) ) ;
#9200=CARTESIAN_POINT ( 'NONE',  ( 11.60466159355862104, 11.60466159355875071, 7.500000000000005329 ) ) ;
#9202=CARTESIAN_POINT ( 'NONE',  ( 1.607813917173037899, -14.26974319298267169, 21.64285714285714590 ) ) ;
#9204=CARTESIAN_POINT ( 'NONE',  ( -11.78653521626494793, -7.556039541191465148, 36.71024514465928235 ) ) ;
#9207=CARTESIAN_POINT ( 'NONE',  ( 15.88516839912898071, 1.917699372586004092, 28.13881657323070939 ) ) ;
#9214=CARTESIAN_POINT ( 'NONE',  ( -13.47998361472151174, -8.620103694222146729, 48.71024514465926814 ) ) ;
#9217=CARTESIAN_POINT ( 'NONE',  ( 9.989344678689365153, -9.809645194533958446, 22.99595943037356705 ) ) ;
#9221=CARTESIAN_POINT ( 'NONE',  ( -13.55419868402807992, -4.742819248065651472, 40.92857142857145192 ) ) ;
#9222=CARTESIAN_POINT ( 'NONE',  ( -4.503970704919988854, 13.25633410266674517, -1.567388001802134223 ) ) ;
#9224=CARTESIAN_POINT ( 'NONE',  ( -15.44746603149413922, -5.543385399275820191, 6.924530858944994982 ) ) ;
#9225=CARTESIAN_POINT ( 'NONE',  ( -7.071314881512976491, 14.31301652532476076, -4.192871190346640879E-15 ) ) ;
#9226=CARTESIAN_POINT ( 'NONE',  ( 15.89939535829187278, 1.791431617653015174, 26.14285714285714590 ) ) ;
#9233=CARTESIAN_POINT ( 'NONE',  ( -13.82664651025767100, 8.841785722321537477, 21.78975485534072476 ) ) ;
#9234=CARTESIAN_POINT ( 'NONE',  ( -15.89939535829186923, -1.791431617653016062, 47.14285714285714590 ) ) ;
#9236=CARTESIAN_POINT ( 'NONE',  ( -13.82664651025767100, 8.841785722321537477, 15.78975485534072121 ) ) ;
#9237=CARTESIAN_POINT ( 'NONE',  ( -13.55419868402807992, -4.742819248065651472, 28.92857142857143771 ) ) ;
#9238=CARTESIAN_POINT ( 'NONE',  ( 5.420364854932001819, 15.49051278174644430, 7.071428571428569398 ) ) ;
#9239=CARTESIAN_POINT ( 'NONE',  ( -5.284464991282755264, 15.10213328493384743, 42.42857142857143060 ) ) ;
#9243=CARTESIAN_POINT ( 'NONE',  ( -13.54758718765249625, -8.512513224245459753, 40.71428571428571530 ) ) ;
#9245=CARTESIAN_POINT ( 'NONE',  ( 7.340858601237956194, 11.92174236212700045, 9.281673716087846415 ) ) ;
#9247=CARTESIAN_POINT ( 'NONE',  ( -5.284464991282755264, 15.10213328493384743, 6.428571428571429713 ) ) ;
#9248=CARTESIAN_POINT ( 'NONE',  ( -16.29368510291090288, 1.967016585148476215, 45.36118342676930837 ) ) ;
#9250=CARTESIAN_POINT ( 'NONE',  ( -4.742819248065500481, -13.55419868402813499, 22.07142857142858006 ) ) ;
#9251=CARTESIAN_POINT ( 'NONE',  ( 7.529642458189280241, -12.22833218042435099, 25.21832628391215181 ) ) ;
#9253=CARTESIAN_POINT ( 'NONE',  ( 4.743843029824831525, -13.17239914596749095, 35.42453085894499765 ) ) ;
#9257=CARTESIAN_POINT ( 'NONE',  ( -5.297344310588352201, -15.53355953199867301, 30.06738800180214355 ) ) ;
#9260=CARTESIAN_POINT ( 'NONE',  ( -9.989344678689363377, 9.809645194533960222, 49.99595943037357415 ) ) ;
#9268=CARTESIAN_POINT ( 'NONE',  ( 1.441234910513245149, 13.92619789766829008, 2.853102287516426916 ) ) ;
#9271=CARTESIAN_POINT ( 'NONE',  ( -8.512513224245306986, -13.54758718765259218, 28.28571428571428825 ) ) ;
#9275=CARTESIAN_POINT ( 'NONE',  ( -14.28433602490915000, 1.478298951650542481, 13.35310228751641937 ) ) ;
#9279=CARTESIAN_POINT ( 'NONE',  ( -15.91362231745475597, -1.665163862720028254, 45.14689771248358596 ) ) ;
#9280=CARTESIAN_POINT ( 'NONE',  ( 4.742819248065503146, 13.55419868402813677, 49.07142857142859071 ) ) ;
#9281=CARTESIAN_POINT ( 'NONE',  ( 7.448449071214646722, 11.85413878919601594, 49.28571428571428470 ) ) ;
#9283=CARTESIAN_POINT ( 'NONE',  ( 1.967016585148662289, -16.29368510291087091, 5.638816573230711171 ) ) ;
#9286=CARTESIAN_POINT ( 'NONE',  ( 1.791431617652837316, 15.89939535829188877, 36.85714285714286120 ) ) ;
#9293=CARTESIAN_POINT ( 'NONE',  ( -15.06016580658428694, 5.404401153735006957, 21.57546914105500946 ) ) ;
#9294=CARTESIAN_POINT ( 'NONE',  ( 1.791431617652837316, 15.89939535829188877, 42.85714285714285410 ) ) ;
#9295=CARTESIAN_POINT ( 'NONE',  ( -5.164528828830334817, 15.14410076328347543, 22.43261199819786356 ) ) ;
#9296=CARTESIAN_POINT ( 'NONE',  ( 8.731428362939190890, -13.89598863503036164, 15.21428571428571530 ) ) ;
#9297=CARTESIAN_POINT ( 'NONE',  ( 3.909482873968459948, 15.52014209590646310, 48.73000000000003951 ) ) ;
#9301=CARTESIAN_POINT ( 'NONE',  ( -13.89598863503045933, 8.731428362939027465, 41.78571428571429180 ) ) ;
#9303=CARTESIAN_POINT ( 'NONE',  ( -15.89939535829186923, -1.791431617653016062, 5.142857142857143238 ) ) ;
#9305=CARTESIAN_POINT ( 'NONE',  ( -1.567502665446231180, -13.91197093850540334, 21.85714285714286120 ) ) ;
#9307=CARTESIAN_POINT ( 'NONE',  ( 13.59724543428031573, 4.619798703722006294, 35.93261199819787066 ) ) ;
#9309=CARTESIAN_POINT ( 'NONE',  ( 12.22833218042443271, -7.529642458189144349, 46.78167371608785885 ) ) ;
#9312=CARTESIAN_POINT ( 'NONE',  ( 1.665163862719847732, 15.91362231745477374, 26.85310228751642470 ) ) ;
#9313=CARTESIAN_POINT ( 'NONE',  ( -15.89939535829186923, -1.791431617653016062, 5.142857142857143238 ) ) ;
#9315=CARTESIAN_POINT ( 'NONE',  ( -8.404922754268618235, -13.61519076058357491, 24.28167371608785530 ) ) ;
#9319=CARTESIAN_POINT ( 'NONE',  ( 4.865839792409144771, 13.51115193377589740, 35.07546914105501656 ) ) ;
#9323=CARTESIAN_POINT ( 'NONE',  ( 13.89774397934249706, 1.693770420379375308, 4.138816573230708507 ) ) ;
#9326=CARTESIAN_POINT ( 'NONE',  ( 1.737328882695370558, -14.25515036105620581, 29.63881657323071295 ) ) ;
#9330=CARTESIAN_POINT ( 'NONE',  ( -7.639999817571787588, 12.15899005565156266, 48.21428571428570820 ) ) ;
#9331=CARTESIAN_POINT ( 'NONE',  ( 8.784089738577305795, 11.01490013464600892, 49.39149694378009769 ) ) ;
#9333=CARTESIAN_POINT ( 'NONE',  ( 11.51250119794888249, 11.69682198916847682, 9.495959430373563492 ) ) ;
#9336=CARTESIAN_POINT ( 'NONE',  ( -1.791431617652833763, -15.89939535829188877, 33.85714285714285410 ) ) ;
#9344=CARTESIAN_POINT ( 'NONE',  ( -8.620103694221995738, -13.47998361472161299, 14.28975485534072298 ) ) ;
#9345=CARTESIAN_POINT ( 'NONE',  ( 15.49051278174638036, 5.420364854932175014, 13.92857142857143238 ) ) ;
#9352=CARTESIAN_POINT ( 'NONE',  ( -8.731428362939189114, 13.89598863503036341, 6.214285714285717965 ) ) ;
#9353=CARTESIAN_POINT ( 'NONE',  ( -15.91362231745475597, -1.665163862720028254, 45.14689771248358596 ) ) ;
#9355=CARTESIAN_POINT ( 'NONE',  ( 7.448449071214646722, 11.85413878919601594, 19.28571428571428825 ) ) ;
#9356=CARTESIAN_POINT ( 'NONE',  ( -10.24623928997352351, -10.06191849875416899, 38.50404056962644006 ) ) ;
#9359=CARTESIAN_POINT ( 'NONE',  ( 11.78653521626494793, 7.556039541191463371, 39.71024514465927524 ) ) ;
#9361=CARTESIAN_POINT ( 'NONE',  ( 15.14410076328353227, -5.164528828830166063, 16.56738800180213289 ) ) ;
#9362=CARTESIAN_POINT ( 'NONE',  ( -5.284464991282755264, 15.10213328493384743, 6.428571428571429713 ) ) ;
#9364=CARTESIAN_POINT ( 'NONE',  ( -15.14410076328353227, 5.164528828830164287, 19.56738800180213644 ) ) ;
#9368=CARTESIAN_POINT ( 'NONE',  ( 10.24623928997352884, 10.06191849875416899, 41.50404056962644006 ) ) ;
#9371=CARTESIAN_POINT ( 'NONE',  ( -10.06191849875405531, -10.24623928997363542, 6.495959430373559051 ) ) ;
#9379=CARTESIAN_POINT ( 'NONE',  ( -15.06016580658428694, 5.404401153735006957, 45.57546914105501656 ) ) ;
#9380=CARTESIAN_POINT ( 'NONE',  ( -4.865839792409144771, -13.51115193377589740, 8.075469141055007682 ) ) ;
#9381=CARTESIAN_POINT ( 'NONE',  ( 9.899494936611610285, 9.899494936611718643, 49.50000000000000711 ) ) ;
#9383=CARTESIAN_POINT ( 'NONE',  ( 8.404922754268618235, 13.61519076058357491, 15.28167371608785174 ) ) ;
#9385=CARTESIAN_POINT ( 'NONE',  ( -1.791431617652833763, -15.89939535829188877, 39.85714285714286120 ) ) ;
#9395=CARTESIAN_POINT ( 'NONE',  ( 15.53355953199861794, 5.297344310588528060, 17.93261199819786711 ) ) ;
#9397=CARTESIAN_POINT ( 'NONE',  ( -5.284464991282755264, 15.10213328493384743, 24.42857142857143060 ) ) ;
#9401=CARTESIAN_POINT ( 'NONE',  ( -0.3453160816774686892, 15.99627321608801367, 48.73000000000002530 ) ) ;
#9403=CARTESIAN_POINT ( 'NONE',  ( -11.31370849898482156, 11.31370849898469544, 0.000000000000000000 ) ) ;
#9405=CARTESIAN_POINT ( 'NONE',  ( 13.21436662431716869, -4.623906867372263640, 44.57142857142857650 ) ) ;
#9406=CARTESIAN_POINT ( 'NONE',  ( 14.25515036105622535, -1.737328882695210241, 30.36118342676929771 ) ) ;
#9410=CARTESIAN_POINT ( 'NONE',  ( -13.25633410266679313, 4.503970704919840529, 43.56738800180213644 ) ) ;
#9412=CARTESIAN_POINT ( 'NONE',  ( -8.841785722321695573, 13.82664651025757152, 20.21024514465928235 ) ) ;
#9413=CARTESIAN_POINT ( 'NONE',  ( -11.60466159355861748, -11.60466159355874893, 10.50000000000000355 ) ) ;
#9416=CARTESIAN_POINT ( 'NONE',  ( 15.88516839912898071, 1.917699372586004092, 22.13881657323070939 ) ) ;
#9423=CARTESIAN_POINT ( 'NONE',  ( -1.967016585148659846, 16.29368510291087091, 50.63881657323071295 ) ) ;
#9426=CARTESIAN_POINT ( 'NONE',  ( -13.51115193377584589, -4.865839792409295761, 24.92453085894499765 ) ) ;
#9432=CARTESIAN_POINT ( 'NONE',  ( 13.92619789766827587, 1.441234910513398582, 6.146897712483580634 ) ) ;
#9433=CARTESIAN_POINT ( 'NONE',  ( 4.865839792409144771, 13.51115193377589740, 5.075469141055008571 ) ) ;
#9436=CARTESIAN_POINT ( 'NONE',  ( 5.297344310588354865, 15.53355953199867301, 9.067388001802141773 ) ) ;
#9437=STYLED_ITEM ( 'NONE', ( #6375 ), #7077 ) ;
#9441=CARTESIAN_POINT ( 'NONE',  ( 5.284464991282756152, -15.10213328493384743, 45.42857142857143060 ) ) ;
#9448=CARTESIAN_POINT ( 'NONE',  ( -5.543385399275643444, -15.44746603149420494, 32.07546914105502367 ) ) ;
#9451=CARTESIAN_POINT ( 'NONE',  ( -8.620103694221995738, -13.47998361472161299, 38.28975485534072476 ) ) ;
#9452=CARTESIAN_POINT ( 'NONE',  ( -8.731428362939189114, 13.89598863503036341, 18.21428571428571885 ) ) ;
#9454=CARTESIAN_POINT ( 'NONE',  ( -5.284464991282755264, 15.10213328493384743, 0.4285714285714309346 ) ) ;
#9457=CIRCLE ( 'NONE', #3170, 1.000000000000000000 ) ;
#9460=CARTESIAN_POINT ( 'NONE',  ( 15.49051278174638036, 5.420364854932175014, 7.928571428571430602 ) ) ;
#9461=CARTESIAN_POINT ( 'NONE',  ( 1.791431617652837316, 15.89939535829188877, 18.85714285714285765 ) ) ;
#9462=CARTESIAN_POINT ( 'NONE',  ( 4.623906867372411078, -13.21436662431711717, 33.42857142857143060 ) ) ;
#9464=CARTESIAN_POINT ( 'NONE',  ( -13.59724543428031573, -4.619798703722008959, 32.93261199819787777 ) ) ;
#9467=CARTESIAN_POINT ( 'NONE',  ( 7.639999817571789364, -12.15899005565156266, 9.214285714285717077 ) ) ;
#9470=CARTESIAN_POINT ( 'NONE',  ( -1.967016585148659846, 16.29368510291087091, 32.63881657323070584 ) ) ;
#9472=CARTESIAN_POINT ( 'NONE',  ( -5.420364854931998266, -15.49051278174643898, 10.07142857142856940 ) ) ;
#9474=CARTESIAN_POINT ( 'NONE',  ( -13.47998361472151174, -8.620103694222146729, 30.71024514465928235 ) ) ;
#9480=CARTESIAN_POINT ( 'NONE',  ( 1.441234910513245149, 13.92619789766829008, 14.85310228751642470 ) ) ;
#9482=CARTESIAN_POINT ( 'NONE',  ( 11.60466159355862104, 11.60466159355875071, 13.50000000000000178 ) ) ;
#9487=CARTESIAN_POINT ( 'NONE',  ( 9.809645194534072132, -9.989344678689256796, 1.004040569626440726 ) ) ;
#9489=CARTESIAN_POINT ( 'NONE',  ( 13.96533075980324234, -8.621071003556521006, 16.78167371608784819 ) ) ;
#9491=CARTESIAN_POINT ( 'NONE',  ( -15.10213328493390961, 5.284464991282586510, 47.57142857142857650 ) ) ;
#9497=CARTESIAN_POINT ( 'NONE',  ( 5.543385399275644332, 15.44746603149420494, 23.07546914105501301 ) ) ;
#9499=CARTESIAN_POINT ( 'NONE',  ( 8.620103694221997515, 13.47998361472160767, 35.28975485534072476 ) ) ;
#9501=CARTESIAN_POINT ( 'NONE',  ( 8.731428362939190890, -13.89598863503036164, 21.21428571428571885 ) ) ;
#9504=CARTESIAN_POINT ( 'NONE',  ( -5.420364854931999155, -15.49051278174644253, 4.071428571428569398 ) ) ;
#9509=CARTESIAN_POINT ( 'NONE',  ( 8.621071003556677326, -13.96533075980314287, 1.218326283912148922 ) ) ;
#9510=CARTESIAN_POINT ( 'NONE',  ( 15.89939535829187278, 1.791431617653015174, 20.14285714285714235 ) ) ;
#9511=CARTESIAN_POINT ( 'NONE',  ( -4.623906867372410190, 13.21436662431711895, 36.42857142857143060 ) ) ;
#9512=CARTESIAN_POINT ( 'NONE',  ( 13.59724543428031573, 4.619798703722006294, 29.93261199819786356 ) ) ;
#9516=CARTESIAN_POINT ( 'NONE',  ( 13.91197093850538380, 1.567502665446386390, 2.142857142857140573 ) ) ;
#9519=CARTESIAN_POINT ( 'NONE',  ( -16.30827793483735988, 1.837501619626141558, 17.35714285714286120 ) ) ;
#9520=CARTESIAN_POINT ( 'NONE',  ( -11.51250119794888072, -11.69682198916848037, 18.49595943037356705 ) ) ;
#9523=CARTESIAN_POINT ( 'NONE',  ( 13.21436662431716869, -4.623906867372263640, 2.571428571428571619 ) ) ;
#9524=CARTESIAN_POINT ( 'NONE',  ( 5.284464991282756152, -15.10213328493384743, 33.42857142857143060 ) ) ;
#9526=CARTESIAN_POINT ( 'NONE',  ( 13.51115193377584589, 4.865839792409294873, 9.924530858944988765 ) ) ;
#9528=CARTESIAN_POINT ( 'NONE',  ( 15.10213328493390783, -5.284464991282587398, 14.57142857142856940 ) ) ;
#9530=CARTESIAN_POINT ( 'NONE',  ( -13.89774397934249706, -1.693770420379375974, 25.13881657323070939 ) ) ;
#9534=CARTESIAN_POINT ( 'NONE',  ( 7.556039541191335474, 11.78653521626503320, -0.7102451446592792372 ) ) ;
#9535=CARTESIAN_POINT ( 'NONE',  ( 13.17239914596754424, -4.743843029824685864, 6.575469141055007682 ) ) ;
#9538=CARTESIAN_POINT ( 'NONE',  ( 5.420364854932001819, 15.49051278174644430, 49.07142857142859071 ) ) ;
#9544=CARTESIAN_POINT ( 'NONE',  ( -11.69682198916834892, -11.51250119794901394, 26.50404056962643651 ) ) ;
#9546=CARTESIAN_POINT ( 'NONE',  ( -16.29368510291090288, 1.967016585148476215, 33.36118342676929416 ) ) ;
#9549=CARTESIAN_POINT ( 'NONE',  ( -8.731428362939189114, 13.89598863503036341, 36.21428571428573662 ) ) ;
#9550=CARTESIAN_POINT ( 'NONE',  ( 1.259487257818240558, 14.39292736161286079, 2.773985284965513663E-17 ) ) ;
#9552=CARTESIAN_POINT ( 'NONE',  ( -8.731428362939189114, 13.89598863503036341, 0.2142857142857168273 ) ) ;
#9557=CARTESIAN_POINT ( 'NONE',  ( 1.693770420379222319, 13.89774397934251837, 46.86118342676930126 ) ) ;
#9558=CARTESIAN_POINT ( 'NONE',  ( -11.60466159355861926, -11.60466159355875249, 16.50000000000000000 ) ) ;
#9559=CARTESIAN_POINT ( 'NONE',  ( -11.85413878919593422, -7.448449071214776396, 40.71428571428571530 ) ) ;
#9560=CARTESIAN_POINT ( 'NONE',  ( -1.478298951650703019, 14.28433602490913579, 40.64689771248358596 ) ) ;
#9561=CARTESIAN_POINT ( 'NONE',  ( -1.607813917173034124, 14.26974319298267524, 12.64285714285714235 ) ) ;
#9565=CARTESIAN_POINT ( 'NONE',  ( -9.899494936611716867, 9.899494936611610285, 5.999999999999998224 ) ) ;
#9567=DIRECTION ( 'NONE',  ( -0.7071067811865519026, 0.7071067811865432429, -6.110863319087399810E-17 ) ) ;
#9568=CARTESIAN_POINT ( 'NONE',  ( -16.30827793483735988, 1.837501619626141558, 11.35714285714285765 ) ) ;
#9569=CARTESIAN_POINT ( 'NONE',  ( -13.96533075980324234, 8.621071003556515677, 43.78167371608784464 ) ) ;
#9572=CARTESIAN_POINT ( 'NONE',  ( -9.899494936611716867, 9.899494936611610285, 0.000000000000000000 ) ) ;
#9575=CARTESIAN_POINT ( 'NONE',  ( -13.89774397934249706, -1.693770420379375974, 19.13881657323070584 ) ) ;
#9578=CARTESIAN_POINT ( 'NONE',  ( -13.25633410266679313, 4.503970704919840529, 43.56738800180213644 ) ) ;
#9582=CARTESIAN_POINT ( 'NONE',  ( 13.59724543428031573, 4.619798703722006294, -0.06738800180213055935 ) ) ;
#9585=CARTESIAN_POINT ( 'NONE',  ( 11.92174236212692229, 7.340858601238088532, 11.71832628391215181 ) ) ;
#9588=CARTESIAN_POINT ( 'NONE',  ( 13.89598863503046111, -8.731428362939032795, 44.78571428571428470 ) ) ;
#9596=CARTESIAN_POINT ( 'NONE',  ( 5.164528828830335705, -15.14410076328347543, 31.43261199819787421 ) ) ;
#9598=CARTESIAN_POINT ( 'NONE',  ( 13.82664651025767100, -8.841785722321541030, 36.78975485534072476 ) ) ;
#9604=CARTESIAN_POINT ( 'NONE',  ( -16.30827793483735988, 1.837501619626141780, 29.35714285714285765 ) ) ;
#9605=CARTESIAN_POINT ( 'NONE',  ( 3.725403445246824319, 14.71619381621854927, 7.152024097607907747E-17 ) ) ;
#9606=CARTESIAN_POINT ( 'NONE',  ( -1.837501619626328297, 16.30827793483733856, 6.642857142857143238 ) ) ;
#9613=CARTESIAN_POINT ( 'NONE',  ( 14.25515036105622535, -1.737328882695210241, 42.36118342676930126 ) ) ;
#9614=CARTESIAN_POINT ( 'NONE',  ( -5.420364854931999155, -15.49051278174644253, 22.07142857142858006 ) ) ;
#9615=CARTESIAN_POINT ( 'NONE',  ( 13.91197093850538380, 1.567502665446386390, 38.14285714285714590 ) ) ;
#9616=CARTESIAN_POINT ( 'NONE',  ( 1.693770420379222319, 13.89774397934251837, 46.86118342676930126 ) ) ;
#9617=CARTESIAN_POINT ( 'NONE',  ( 4.742819248065503146, 13.55419868402813677, 7.071428571428569398 ) ) ;
#9621=CARTESIAN_POINT ( 'NONE',  ( -1.737328882695368115, 14.25515036105620581, 50.63881657323071295 ) ) ;
#9624=CARTESIAN_POINT ( 'NONE',  ( -15.10213328493390961, 5.284464991282586510, 23.57142857142857650 ) ) ;
#9625=CARTESIAN_POINT ( 'NONE',  ( -13.47998361472151174, -8.620103694222146729, 36.71024514465928235 ) ) ;
#9630=CARTESIAN_POINT ( 'NONE',  ( -4.743843029824828861, 13.17239914596749450, 20.42453085894499054 ) ) ;
#9632=CARTESIAN_POINT ( 'NONE',  ( -1.791431617652833763, -15.89939535829188877, 9.857142857142855874 ) ) ;
#9634=CARTESIAN_POINT ( 'NONE',  ( -4.619798703721853528, -13.59724543428036725, 42.06738800180214355 ) ) ;
#9638=CARTESIAN_POINT ( 'NONE',  ( 1.478298951650704351, -14.28433602490913579, 19.64689771248358596 ) ) ;
#9640=CARTESIAN_POINT ( 'NONE',  ( 13.17239914596754424, -4.743843029824685864, 12.57546914105500768 ) ) ;
#9643=CARTESIAN_POINT ( 'NONE',  ( -1.967016585148659846, 16.29368510291087091, 14.63881657323070939 ) ) ;
#9649=CARTESIAN_POINT ( 'NONE',  ( 14.26974319298268767, -1.607813917172876916, 32.35714285714286120 ) ) ;
#9650=CARTESIAN_POINT ( 'NONE',  ( 1.917699372585825790, 15.88516839912900203, 34.86118342676929416 ) ) ;
#9654=CARTESIAN_POINT ( 'NONE',  ( 16.30827793483735633, -1.837501619626142890, 26.35714285714285765 ) ) ;
#9656=CARTESIAN_POINT ( 'NONE',  ( 5.284464991282756152, -15.10213328493384743, 15.42857142857143060 ) ) ;
#9659=CARTESIAN_POINT ( 'NONE',  ( -4.503970704919988854, 13.25633410266674517, 46.43261199819787066 ) ) ;
#9660=CARTESIAN_POINT ( 'NONE',  ( -1.791431617652833763, -15.89939535829188877, 15.85714285714286120 ) ) ;
#9662=CARTESIAN_POINT ( 'NONE',  ( 7.556039541191335474, 11.78653521626503320, 41.28975485534072476 ) ) ;
#9663=CARTESIAN_POINT ( 'NONE',  ( 10.15407889436379030, 10.15407889436390576, 13.50000000000000178 ) ) ;
#9667=CARTESIAN_POINT ( 'NONE',  ( 7.639999817571789364, -12.15899005565156266, 3.214285714285716633 ) ) ;
#9669=DIRECTION ( 'NONE',  ( 0.7071067811865519026, -0.7071067811865431318, 0.000000000000000000 ) ) ;
#9670=CARTESIAN_POINT ( 'NONE',  ( 15.89939535829187278, 1.791431617653015174, 14.14285714285714413 ) ) ;
#9671=CARTESIAN_POINT ( 'NONE',  ( 15.88516839912898071, 1.917699372586004092, 34.13881657323070584 ) ) ;
#9675=CARTESIAN_POINT ( 'NONE',  ( -4.619798703721853528, -13.59724543428036725, 12.06738800180214000 ) ) ;
#9678=CARTESIAN_POINT ( 'NONE',  ( -15.49051278174638036, -5.420364854932175902, 16.92857142857143771 ) ) ;
#9680=CARTESIAN_POINT ( 'NONE',  ( 9.989344678689365153, -9.809645194533958446, 40.99595943037355994 ) ) ;
#9687=CARTESIAN_POINT ( 'NONE',  ( 15.88516839912898071, 1.917699372586004092, 4.138816573230708507 ) ) ;
#9694=CARTESIAN_POINT ( 'NONE',  ( 12.15899005565164792, -7.639999817571655250, 32.78571428571430602 ) ) ;
#9695=CARTESIAN_POINT ( 'NONE',  ( 15.06016580658428694, -5.404401153735007846, 42.57546914105501656 ) ) ;
#9698=CARTESIAN_POINT ( 'NONE',  ( -1.791431617652833763, -15.89939535829188877, 27.85714285714285765 ) ) ;
#9699=CARTESIAN_POINT ( 'NONE',  ( 3.907812701641489639, 14.44795834638319398, 1.336143574212688912E-16 ) ) ;
#9700=CARTESIAN_POINT ( 'NONE',  ( -13.54758718765249625, -8.512513224245459753, 16.71428571428571530 ) ) ;
#9701=DIRECTION ( 'NONE',  ( -2.311115933264683708E-33, 1.040834085586086106E-16, 1.000000000000000000 ) ) ;
#9705=CARTESIAN_POINT ( 'NONE',  ( 1.917699372585825790, 15.88516839912900203, 10.86118342676929238 ) ) ;
#9706=CARTESIAN_POINT ( 'NONE',  ( -13.89598863503046111, 8.731428362939027465, 29.78571428571428825 ) ) ;
#9709=CARTESIAN_POINT ( 'NONE',  ( 13.82664651025767100, -8.841785722321541030, 0.7897548553407187644 ) ) ;
#9710=CARTESIAN_POINT ( 'NONE',  ( -14.26974319298268767, 1.607813917172874918, 17.35714285714286476 ) ) ;
#9715=CARTESIAN_POINT ( 'NONE',  ( -13.55419868402807992, -4.742819248065651472, 22.92857142857142705 ) ) ;
#9718=CARTESIAN_POINT ( 'NONE',  ( -1.791431617652833763, -15.89939535829188877, 27.85714285714285765 ) ) ;
#9719=CARTESIAN_POINT ( 'NONE',  ( 8.404922754268618235, 13.61519076058357491, 39.28167371608785174 ) ) ;
#9722=CARTESIAN_POINT ( 'NONE',  ( 12.15899005565164792, -7.639999817571654361, 14.78571428571429180 ) ) ;
#9725=CARTESIAN_POINT ( 'NONE',  ( -9.989344678689363377, 9.809645194533960222, 31.99595943037357060 ) ) ;
#9728=CARTESIAN_POINT ( 'NONE',  ( -11.60466159355861926, -11.60466159355875249, 16.50000000000000000 ) ) ;
#9731=CARTESIAN_POINT ( 'NONE',  ( 14.28433602490915000, -1.478298951650544479, 40.35310228751642825 ) ) ;
#9735=CARTESIAN_POINT ( 'NONE',  ( -1.693770420379220099, -13.89774397934251837, 13.86118342676929416 ) ) ;
#9736=CARTESIAN_POINT ( 'NONE',  ( 11.92174236212692229, 7.340858601238088532, 23.71832628391215181 ) ) ;
#9738=CARTESIAN_POINT ( 'NONE',  ( 11.09109556827038467, 11.02177121192640818, 48.73000000000001819 ) ) ;
#9739=CARTESIAN_POINT ( 'NONE',  ( -5.404401153735176599, 15.06016580658422477, 8.424530858944992318 ) ) ;
#9745=CARTESIAN_POINT ( 'NONE',  ( -13.21436662431716869, 4.623906867372262752, 35.57142857142857650 ) ) ;
#9747=CARTESIAN_POINT ( 'NONE',  ( 12.15899005565164792, -7.639999817571655250, 32.78571428571430602 ) ) ;
#9750=CARTESIAN_POINT ( 'NONE',  ( 11.31370849898482334, -11.31370849898469366, 33.00000000000000000 ) ) ;
#9753=CARTESIAN_POINT ( 'NONE',  ( -13.89598863503046111, 8.731428362939027465, 17.78571428571428115 ) ) ;
#9757=CARTESIAN_POINT ( 'NONE',  ( -15.53355953199861794, -5.297344310588530725, 14.93261199819787066 ) ) ;
#9759=CARTESIAN_POINT ( 'NONE',  ( -15.10213328493390961, 5.284464991282586510, 35.57142857142857650 ) ) ;
#9763=CARTESIAN_POINT ( 'NONE',  ( -11.69682198916834892, -11.51250119794901394, 2.504040569626438728 ) ) ;
#9764=CARTESIAN_POINT ( 'NONE',  ( -11.85413878919593422, -7.448449071214776396, 10.71428571428571708 ) ) ;
#9768=CARTESIAN_POINT ( 'NONE',  ( -14.26974319298268767, 1.607813917172874918, 17.35714285714286476 ) ) ;
#9771=CARTESIAN_POINT ( 'NONE',  ( -5.420364854931998266, -15.49051278174643898, 28.07142857142857295 ) ) ;
#9772=CARTESIAN_POINT ( 'NONE',  ( 1.967016585148662289, -16.29368510291087091, 35.63881657323071295 ) ) ;
#9775=CARTESIAN_POINT ( 'NONE',  ( -13.55419868402807992, -4.742819248065651472, 4.928571428571430602 ) ) ;
#9779=CARTESIAN_POINT ( 'NONE',  ( 4.743843029824831525, -13.17239914596749095, 29.42453085894499765 ) ) ;
#9782=CARTESIAN_POINT ( 'NONE',  ( 7.042703574009315126, 12.29825027030509865, 48.73000000000005372 ) ) ;
#9783=CARTESIAN_POINT ( 'NONE',  ( -9.989344678689363377, 9.809645194533960222, 37.99595943037355994 ) ) ;
#9788=CARTESIAN_POINT ( 'NONE',  ( -13.17239914596754424, 4.743843029824683200, 15.57546914105500413 ) ) ;
#9791=CARTESIAN_POINT ( 'NONE',  ( 1.665163862719847732, 15.91362231745477374, 38.85310228751641404 ) ) ;
#9793=CARTESIAN_POINT ( 'NONE',  ( -10.36771240197842303, 11.87284897423499785, 48.72999999999976239 ) ) ;
#9794=CARTESIAN_POINT ( 'NONE',  ( 5.404401153735178376, -15.06016580658422477, 5.424530858944991429 ) ) ;
#9799=CARTESIAN_POINT ( 'NONE',  ( 7.639999817571789364, -12.15899005565156266, 27.21428571428572241 ) ) ;
#9802=CARTESIAN_POINT ( 'NONE',  ( 15.49051278174638036, 5.420364854932175014, 43.92857142857143060 ) ) ;
#9804=CARTESIAN_POINT ( 'NONE',  ( -15.49051278174638036, -5.420364854932175902, 10.92857142857142883 ) ) ;
#9810=CARTESIAN_POINT ( 'NONE',  ( 11.22385875690717683, -11.40355824106234373, 13.00404056962644006 ) ) ;
#9811=CARTESIAN_POINT ( 'NONE',  ( 1.837501619626330074, -16.30827793483733501, 27.64285714285714590 ) ) ;
#9813=CARTESIAN_POINT ( 'NONE',  ( 11.69682198916835070, 11.51250119794901394, -0.4959594303735606058 ) ) ;
#9814=CARTESIAN_POINT ( 'NONE',  ( 7.639999817571789364, -12.15899005565156266, 27.21428571428572241 ) ) ;
#9815=CARTESIAN_POINT ( 'NONE',  ( -1.791431617652833763, -15.89939535829188877, 9.857142857142855874 ) ) ;
#9818=CARTESIAN_POINT ( 'NONE',  ( 4.742819248065503146, 13.55419868402813677, 13.07142857142857295 ) ) ;
#9820=CARTESIAN_POINT ( 'NONE',  ( -15.10213328493390961, 5.284464991282586510, 35.57142857142857650 ) ) ;
#9821=CARTESIAN_POINT ( 'NONE',  ( 14.28433602490915000, -1.478298951650544479, 4.353102287516421143 ) ) ;
#9824=CARTESIAN_POINT ( 'NONE',  ( -11.85413878919593422, -7.448449071214776396, 16.71428571428571530 ) ) ;
#9825=CARTESIAN_POINT ( 'NONE',  ( 10.06191849875406064, 10.24623928997363187, 27.49595943037356705 ) ) ;
#9826=ORIENTED_EDGE ( 'NONE', *, *, #4236, .F. ) ;
#9831=CARTESIAN_POINT ( 'NONE',  ( -11.78653521626494793, -7.556039541191465148, 48.71024514465926814 ) ) ;
#9836=CARTESIAN_POINT ( 'NONE',  ( -11.40355824106246807, 11.22385875690704715, 37.99595943037355994 ) ) ;
#9838=CARTESIAN_POINT ( 'NONE',  ( -13.18366518639671625, 7.227486437412175668, 48.73000000000003240 ) ) ;
#9839=CARTESIAN_POINT ( 'NONE',  ( -15.89939535829186923, -1.791431617653016062, 23.14285714285714590 ) ) ;
#9844=CARTESIAN_POINT ( 'NONE',  ( 1.707986654103998303, -16.32287076676380266, 37.64689771248358596 ) ) ;
#9845=CARTESIAN_POINT ( 'NONE',  ( 7.448449071214646722, 11.85413878919601594, 25.28571428571428470 ) ) ;
#9846=CARTESIAN_POINT ( 'NONE',  ( 13.91197093850538380, 1.567502665446386390, 44.14285714285714590 ) ) ;
#9848=CARTESIAN_POINT ( 'NONE',  ( 8.404922754268618235, 13.61519076058357491, 3.281673716087854409 ) ) ;
#9849=CARTESIAN_POINT ( 'NONE',  ( 2.826141341537784513, 15.12951547267378949, 6.336793937239309722E-15 ) ) ;
#9850=CARTESIAN_POINT ( 'NONE',  ( 15.89939535829187278, 1.791431617653015174, 14.14285714285714413 ) ) ;
#9854=CARTESIAN_POINT ( 'NONE',  ( -8.621071003556675549, 13.96533075980314642, 10.21832628391215358 ) ) ;
#9855=CARTESIAN_POINT ( 'NONE',  ( -15.49051278174638036, -5.420364854932175902, 34.92857142857145192 ) ) ;
#9857=CARTESIAN_POINT ( 'NONE',  ( 11.69682198916835070, 11.51250119794901394, 11.50404056962644006 ) ) ;
#9858=CARTESIAN_POINT ( 'NONE',  ( -10.15407889436378852, -10.15407889436390576, 22.50000000000000000 ) ) ;
#9859=CARTESIAN_POINT ( 'NONE',  ( 13.89598863503046111, -8.731428362939032795, 2.785714285714284255 ) ) ;
#9860=CARTESIAN_POINT ( 'NONE',  ( -8.731428362939189114, 13.89598863503036341, 42.21428571428572241 ) ) ;
#9862=CARTESIAN_POINT ( 'NONE',  ( -1.607813917173034124, 14.26974319298267524, 12.64285714285714235 ) ) ;
#9865=CARTESIAN_POINT ( 'NONE',  ( 5.420364854932000931, 15.49051278174644075, 37.07142857142857650 ) ) ;
#9866=CARTESIAN_POINT ( 'NONE',  ( 11.51250119794888249, 11.69682198916847682, 45.49595943037356705 ) ) ;
#9870=CARTESIAN_POINT ( 'NONE',  ( -11.85413878919593422, -7.448449071214776396, 10.71428571428571708 ) ) ;
#9872=CARTESIAN_POINT ( 'NONE',  ( 1.737328882695370558, -14.25515036105620581, 29.63881657323071295 ) ) ;
#9877=CARTESIAN_POINT ( 'NONE',  ( -7.750357176954294935, 12.08964793087877787, 50.21024514465927524 ) ) ;
#9881=CARTESIAN_POINT ( 'NONE',  ( -13.92619789766827054, -1.441234910513399470, 27.14689771248358241 ) ) ;
#9885=CARTESIAN_POINT ( 'NONE',  ( -11.51250119794888072, -11.69682198916848037, 36.49595943037355994 ) ) ;
#9887=CARTESIAN_POINT ( 'NONE',  ( -13.89598863503046111, 8.731428362939027465, 23.78571428571429536 ) ) ;
#9889=CARTESIAN_POINT ( 'NONE',  ( 11.78653521626494793, 7.556039541191463371, 9.710245144659278793 ) ) ;
#9893=CARTESIAN_POINT ( 'NONE',  ( 7.448449071214646722, 11.85413878919601594, 49.28571428571428470 ) ) ;
#9895=CARTESIAN_POINT ( 'NONE',  ( -13.21436662431716869, 4.623906867372262752, 41.57142857142856940 ) ) ;
#9897=CARTESIAN_POINT ( 'NONE',  ( 13.89598863503046111, -8.731428362939032795, 38.78571428571429180 ) ) ;
#9899=CARTESIAN_POINT ( 'NONE',  ( -8.731428362939189114, 13.89598863503036341, 30.21428571428572596 ) ) ;
#9907=CARTESIAN_POINT ( 'NONE',  ( -11.22385875690717327, 11.40355824106234550, 10.00404056962643651 ) ) ;
#9908=CARTESIAN_POINT ( 'NONE',  ( -11.31370849898482156, 11.31370849898469544, 24.00000000000000000 ) ) ;
#9911=CARTESIAN_POINT ( 'NONE',  ( -15.06016580658428694, 5.404401153735006957, 3.575469141055005462 ) ) ;
#9913=CARTESIAN_POINT ( 'NONE',  ( 12.15899005565164792, -7.639999817571655250, 26.78571428571429536 ) ) ;
#9914=CARTESIAN_POINT ( 'NONE',  ( 13.54758718765249803, 8.512513224245457977, 7.714285714285715301 ) ) ;
#9915=CARTESIAN_POINT ( 'NONE',  ( -11.60466159355861926, -11.60466159355875249, 40.50000000000000711 ) ) ;
#9917=CARTESIAN_POINT ( 'NONE',  ( -7.639999817571787588, 12.15899005565156266, 12.21428571428571885 ) ) ;
#9919=CARTESIAN_POINT ( 'NONE',  ( -15.49051278174637858, -5.420364854932175014, 28.92857142857143415 ) ) ;
#9923=CARTESIAN_POINT ( 'NONE',  ( -13.96533075980324234, 8.621071003556515677, 49.78167371608785885 ) ) ;
#9925=CARTESIAN_POINT ( 'NONE',  ( -4.623906867372410190, 13.21436662431711895, 30.42857142857143060 ) ) ;
#9926=AXIS2_PLACEMENT_3D ( 'NONE', #6523, #9701, #7365 ) ;
#9928=CARTESIAN_POINT ( 'NONE',  ( 9.989344678689365153, -9.809645194533958446, 28.99595943037357060 ) ) ;
#9931=CARTESIAN_POINT ( 'NONE',  ( 8.270439026029094975, 11.56191342138348332, 48.73000000000006082 ) ) ;
#9934=CARTESIAN_POINT ( 'NONE',  ( 4.623906867372411078, -13.21436662431711717, 3.428571428571426605 ) ) ;
#9939=CARTESIAN_POINT ( 'NONE',  ( -1.967016585148659846, 16.29368510291087091, 38.63881657323070584 ) ) ;
#9940=CARTESIAN_POINT ( 'NONE',  ( -11.94288718622185641, 8.325416427328844904, 48.73000000000002530 ) ) ;
#9943=CARTESIAN_POINT ( 'NONE',  ( 11.78653521626494793, 7.556039541191463371, 15.71024514465927879 ) ) ;
#9947=CARTESIAN_POINT ( 'NONE',  ( 4.865839792409144771, 13.51115193377589740, -0.9245308589449906522 ) ) ;
#9949=CARTESIAN_POINT ( 'NONE',  ( 7.639999817571789364, -12.15899005565156266, 33.21428571428571530 ) ) ;
#9951=CARTESIAN_POINT ( 'NONE',  ( 1.837501619626330074, -16.30827793483733501, 39.64285714285716722 ) ) ;
#9953=CARTESIAN_POINT ( 'NONE',  ( 8.512513224245308763, 13.54758718765259040, 31.28571428571428470 ) ) ;
#9961=CARTESIAN_POINT ( 'NONE',  ( -16.30827793483735988, 1.837501619626141780, 41.35714285714286120 ) ) ;
#9962=CARTESIAN_POINT ( 'NONE',  ( -1.707986654103994528, 16.32287076676380266, 22.64689771248357530 ) ) ;
#9963=CARTESIAN_POINT ( 'NONE',  ( -15.89939535829186923, -1.791431617653016062, 11.14285714285714235 ) ) ;
#9969=CARTESIAN_POINT ( 'NONE',  ( 1.967016585148662289, -16.29368510291087091, 47.63881657323071295 ) ) ;
#9971=CARTESIAN_POINT ( 'NONE',  ( -11.31370849898482156, 11.31370849898469544, 5.999999999999998224 ) ) ;
#9973=CARTESIAN_POINT ( 'NONE',  ( 4.623906867372411078, -13.21436662431711717, 21.42857142857142705 ) ) ;
#9974=CARTESIAN_POINT ( 'NONE',  ( 7.340858601237956194, 11.92174236212700045, 45.28167371608785174 ) ) ;
#9978=CARTESIAN_POINT ( 'NONE',  ( -11.40355824106246807, 11.22385875690704715, 13.99595943037356527 ) ) ;
#9981=CARTESIAN_POINT ( 'NONE',  ( -1.607813917173034124, 14.26974319298267524, 0.6428571428571432378 ) ) ;
#9985=CARTESIAN_POINT ( 'NONE',  ( 9.809645194534072132, -9.989344678689256796, 25.00404056962644006 ) ) ;
#9988=CARTESIAN_POINT ( 'NONE',  ( 11.40355824106246985, -11.22385875690704538, 46.99595943037356705 ) ) ;
#9989=CARTESIAN_POINT ( 'NONE',  ( -13.20914943391479390, 7.349713873783697338, 48.72999999999999687 ) ) ;
#9991=CARTESIAN_POINT ( 'NONE',  ( 13.89774397934249706, 1.693770420379375308, 22.13881657323070939 ) ) ;
#9995=CARTESIAN_POINT ( 'NONE',  ( 1.567502665446232957, 13.91197093850540156, 48.85714285714286120 ) ) ;
#9996=CARTESIAN_POINT ( 'NONE',  ( -9.809645194534070356, 9.989344678689256796, -1.995959430373561272 ) ) ;
#9998=CARTESIAN_POINT ( 'NONE',  ( 15.10213328493390783, -5.284464991282587398, 38.57142857142857650 ) ) ;
#10000=CARTESIAN_POINT ( 'NONE',  ( 8.731428362939190890, -13.89598863503036164, 27.21428571428572241 ) ) ;
#10006=CARTESIAN_POINT ( 'NONE',  ( -11.60466159355861926, -11.60466159355875249, 46.50000000000002132 ) ) ;
#10007=CARTESIAN_POINT ( 'NONE',  ( 8.620103694221997515, 13.47998361472160767, 23.28975485534072121 ) ) ;
#10008=CARTESIAN_POINT ( 'NONE',  ( -13.55419868402807992, -4.742819248065651472, 22.92857142857142705 ) ) ;
#10009=CARTESIAN_POINT ( 'NONE',  ( 8.731428362939190890, -13.89598863503036164, 3.214285714285716633 ) ) ;
#10010=CARTESIAN_POINT ( 'NONE',  ( -15.49051278174638036, -5.420364854932175902, 46.92857142857142350 ) ) ;
#10014=CARTESIAN_POINT ( 'NONE',  ( 8.512513224245308763, 13.54758718765259040, 43.28571428571429180 ) ) ;
#10015=CARTESIAN_POINT ( 'NONE',  ( -7.750357176954294935, 12.08964793087877787, 8.210245144659282346 ) ) ;
#10017=CARTESIAN_POINT ( 'NONE',  ( -8.620103694221995738, -13.47998361472161299, 44.28975485534073186 ) ) ;
#10019=CARTESIAN_POINT ( 'NONE',  ( -12.15899005565164792, 7.639999817571650809, 29.78571428571428825 ) ) ;
#10021=CARTESIAN_POINT ( 'NONE',  ( 13.17239914596754424, -4.743843029824685864, 24.57546914105500946 ) ) ;
#10024=CARTESIAN_POINT ( 'NONE',  ( -1.441234910513241818, -13.92619789766829008, 41.85310228751642825 ) ) ;
#10027=CARTESIAN_POINT ( 'NONE',  ( 5.404401153735178376, -15.06016580658422477, 29.42453085894499765 ) ) ;
#10028=CARTESIAN_POINT ( 'NONE',  ( 13.89598863503045933, -8.731428362939032795, 8.785714285714290028 ) ) ;
#10030=CARTESIAN_POINT ( 'NONE',  ( 13.51115193377584589, 4.865839792409294873, 45.92453085894500475 ) ) ;
#10035=CARTESIAN_POINT ( 'NONE',  ( 8.404922754268618235, 13.61519076058357491, 51.28167371608785174 ) ) ;
#10037=CARTESIAN_POINT ( 'NONE',  ( -11.31370849898482156, 11.31370849898469544, 0.000000000000000000 ) ) ;
#10038=CARTESIAN_POINT ( 'NONE',  ( -13.25633410266679313, 4.503970704919840529, 13.56738800180213822 ) ) ;
#10042=CARTESIAN_POINT ( 'NONE',  ( -5.543385399275643444, -15.44746603149420494, 44.07546914105503078 ) ) ;
#10043=CARTESIAN_POINT ( 'NONE',  ( -12.15899005565164792, 7.639999817571651697, 47.78571428571430602 ) ) ;
#10044=CARTESIAN_POINT ( 'NONE',  ( -4.742819248065502258, -13.55419868402813677, 46.07142857142856940 ) ) ;
#10046=CARTESIAN_POINT ( 'NONE',  ( 8.841785722321695573, -13.82664651025757152, 11.21024514465928235 ) ) ;
#10048=CARTESIAN_POINT ( 'NONE',  ( -13.89598863503046111, 8.731428362939027465, 35.78571428571429180 ) ) ;
#10056=CARTESIAN_POINT ( 'NONE',  ( -11.22385875690717327, 11.40355824106234550, 22.00404056962643651 ) ) ;
#10057=CARTESIAN_POINT ( 'NONE',  ( -5.284464991282755264, 15.10213328493384743, 48.42857142857143060 ) ) ;
#10058=CARTESIAN_POINT ( 'NONE',  ( 16.29368510291089223, -1.967016585148476882, 18.36118342676929771 ) ) ;
#10059=CARTESIAN_POINT ( 'NONE',  ( -13.54758718765249625, -8.512513224245459753, 22.71428571428571530 ) ) ;
#10064=CARTESIAN_POINT ( 'NONE',  ( -15.10213328493390961, 5.284464991282586510, 41.57142857142856940 ) ) ;
#10067=CARTESIAN_POINT ( 'NONE',  ( 8.621071003556677326, -13.96533075980314287, 43.21832628391217668 ) ) ;
#10069=CARTESIAN_POINT ( 'NONE',  ( 13.91197093850538380, 1.567502665446386390, 20.14285714285714235 ) ) ;
#10070=CARTESIAN_POINT ( 'NONE',  ( 9.809645194534072132, -9.989344678689256796, 37.00404056962644006 ) ) ;
#10072=CARTESIAN_POINT ( 'NONE',  ( 11.78653521626494793, 7.556039541191463371, 45.71024514465928235 ) ) ;
#10076=CARTESIAN_POINT ( 'NONE',  ( -15.88516839912898071, -1.917699372586004980, 25.13881657323070939 ) ) ;
#10080=CARTESIAN_POINT ( 'NONE',  ( -8.841785722321695573, 13.82664651025757152, 26.21024514465928945 ) ) ;
#10084=CARTESIAN_POINT ( 'NONE',  ( -7.529642458189277576, 12.22833218042435455, 34.21832628391215536 ) ) ;
#10089=CARTESIAN_POINT ( 'NONE',  ( 15.14410076328353227, -5.164528828830166063, 46.56738800180214355 ) ) ;
#10095=CARTESIAN_POINT ( 'NONE',  ( 11.78653521626494793, 7.556039541191463371, 21.71024514465928235 ) ) ;
#10099=CARTESIAN_POINT ( 'NONE',  ( -5.164528828830334817, 15.14410076328347543, 46.43261199819787066 ) ) ;
#10100=CARTESIAN_POINT ( 'NONE',  ( -14.26974319298268767, 1.607813917172874918, 47.35714285714286120 ) ) ;
#10101=CARTESIAN_POINT ( 'NONE',  ( -1.567502665446231180, -13.91197093850540334, 45.85714285714286120 ) ) ;
#10103=CARTESIAN_POINT ( 'NONE',  ( -16.32287076676382398, 1.707986654103809343, 13.35310228751641937 ) ) ;
#10105=CARTESIAN_POINT ( 'NONE',  ( -13.89598863503046111, 8.731428362939027465, 23.78571428571429536 ) ) ;
#10112=CARTESIAN_POINT ( 'NONE',  ( -5.284464991282755264, 15.10213328493384743, 36.42857142857143060 ) ) ;
#10113=CARTESIAN_POINT ( 'NONE',  ( 13.61519076058348254, 8.404922754268771001, 17.71832628391214826 ) ) ;
#10114=CARTESIAN_POINT ( 'NONE',  ( 16.30827793483735633, -1.837501619626142890, 20.35714285714286476 ) ) ;
#10118=CARTESIAN_POINT ( 'NONE',  ( -2.885895625854219215, 15.94142900571889143, 48.57768213684324365 ) ) ;
#10120=CARTESIAN_POINT ( 'NONE',  ( 1.791431617652837316, 15.89939535829188877, 6.857142857142860315 ) ) ;
#10121=CARTESIAN_POINT ( 'NONE',  ( 13.21436662431716869, -4.623906867372263640, 26.57142857142857295 ) ) ;
#10122=CARTESIAN_POINT ( 'NONE',  ( 7.529642458189280241, -12.22833218042435099, 31.21832628391215536 ) ) ;
#10125=CARTESIAN_POINT ( 'NONE',  ( -1.441234910513241818, -13.92619789766829008, 47.85310228751642114 ) ) ;
#10128=CARTESIAN_POINT ( 'NONE',  ( -8.841785722321695573, 13.82664651025757152, 26.21024514465928945 ) ) ;
#10129=CARTESIAN_POINT ( 'NONE',  ( 11.60466159355861926, 11.60466159355874716, 7.500000000000004441 ) ) ;
#10131=CARTESIAN_POINT ( 'NONE',  ( 11.40355824106246985, -11.22385875690704538, 28.99595943037357060 ) ) ;
#10135=CARTESIAN_POINT ( 'NONE',  ( -1.478298951650703019, 14.28433602490913579, 46.64689771248358596 ) ) ;
#10138=CARTESIAN_POINT ( 'NONE',  ( -9.989344678689363377, 9.809645194533960222, 7.995959430373565269 ) ) ;
#10140=CARTESIAN_POINT ( 'NONE',  ( 15.10213328493390783, -5.284464991282587398, 26.57142857142857295 ) ) ;
#10142=CARTESIAN_POINT ( 'NONE',  ( -9.989344678689363377, 9.809645194533960222, 25.99595943037356349 ) ) ;
#10147=CARTESIAN_POINT ( 'NONE',  ( 8.621071003556677326, -13.96533075980314287, 43.21832628391217668 ) ) ;
#10148=CARTESIAN_POINT ( 'NONE',  ( -13.92619789766827054, -1.441234910513399470, 9.146897712483580634 ) ) ;
#10149=CARTESIAN_POINT ( 'NONE',  ( -1.607813917173034124, 14.26974319298267524, 48.64285714285716011 ) ) ;
#10151=CARTESIAN_POINT ( 'NONE',  ( -1.967016585148659846, 16.29368510291087091, 14.63881657323070939 ) ) ;
#10153=CARTESIAN_POINT ( 'NONE',  ( -15.89939535829186923, -1.791431617653016062, 41.14285714285714590 ) ) ;
#10159=CARTESIAN_POINT ( 'NONE',  ( 15.53355953199861794, 5.297344310588528060, 17.93261199819786711 ) ) ;
#10160=CARTESIAN_POINT ( 'NONE',  ( 8.512513224245308763, 13.54758718765259040, 43.28571428571429180 ) ) ;
#10161=CARTESIAN_POINT ( 'NONE',  ( -5.543385399275643444, -15.44746603149420494, 20.07546914105500591 ) ) ;
#10162=CARTESIAN_POINT ( 'NONE',  ( -11.31370849898482156, 11.31370849898469544, 24.00000000000000000 ) ) ;
#10165=CARTESIAN_POINT ( 'NONE',  ( 11.31370849898482334, -11.31370849898469366, 9.000000000000001776 ) ) ;
#10166=CARTESIAN_POINT ( 'NONE',  ( -5.420364854931998266, -15.49051278174643898, 40.07142857142857650 ) ) ;
#10168=CARTESIAN_POINT ( 'NONE',  ( -1.791431617652833763, -15.89939535829188877, 3.857142857142857650 ) ) ;
#10169=CARTESIAN_POINT ( 'NONE',  ( 1.837501619626330074, -16.30827793483733501, 3.642857142857144126 ) ) ;
#10171=CARTESIAN_POINT ( 'NONE',  ( 13.91197093850538380, 1.567502665446386390, 44.14285714285714590 ) ) ;
#10172=CARTESIAN_POINT ( 'NONE',  ( -11.92174236212692051, -7.340858601238089420, 38.71832628391214826 ) ) ;
#10176=CARTESIAN_POINT ( 'NONE',  ( -11.78653521626494793, -7.556039541191465148, 42.71024514465928235 ) ) ;
#10179=CARTESIAN_POINT ( 'NONE',  ( 5.404401153735178376, -15.06016580658422477, 17.42453085894499409 ) ) ;
#10180=CARTESIAN_POINT ( 'NONE',  ( 5.284464991282756152, -15.10213328493384743, 9.428571428571425272 ) ) ;
#10182=CARTESIAN_POINT ( 'NONE',  ( 8.841785722321695573, -13.82664651025757152, 23.21024514465928235 ) ) ;
#10187=EDGE_CURVE ( 'NONE', #6566, #6853, #1375, .T. ) ;
#10189=CARTESIAN_POINT ( 'NONE',  ( 8.841785722321695573, -13.82664651025757152, 47.21024514465928235 ) ) ;
#10192=CARTESIAN_POINT ( 'NONE',  ( -8.731428362939189114, 13.89598863503036341, 12.21428571428571885 ) ) ;
#10194=CARTESIAN_POINT ( 'NONE',  ( -7.750357176954294935, 12.08964793087877787, 26.21024514465928945 ) ) ;
#10198=CARTESIAN_POINT ( 'NONE',  ( -10.24623928997352351, -10.06191849875416899, 2.504040569626438728 ) ) ;
#10199=CARTESIAN_POINT ( 'NONE',  ( 1.693770420379222319, 13.89774397934251837, 4.861183426769296823 ) ) ;
#10201=CARTESIAN_POINT ( 'NONE',  ( 5.404401153735178376, -15.06016580658422477, 5.424530858944991429 ) ) ;
#10203=CARTESIAN_POINT ( 'NONE',  ( 8.731428362939190890, -13.89598863503036164, 45.21428571428572951 ) ) ;
#10209=CARTESIAN_POINT ( 'NONE',  ( -13.89598863503046111, 8.731428362939027465, 35.78571428571429180 ) ) ;
#10211=CARTESIAN_POINT ( 'NONE',  ( 13.82664651025767100, -8.841785722321541030, 30.78975485534071765 ) ) ;
#10213=CARTESIAN_POINT ( 'NONE',  ( 15.91362231745475597, 1.665163862720026255, 30.14689771248358241 ) ) ;
#10215=CARTESIAN_POINT ( 'NONE',  ( -11.31370849898482156, 11.31370849898469544, 11.99999999999999645 ) ) ;
#10216=CARTESIAN_POINT ( 'NONE',  ( 10.73878802356280104, 11.43342105301867662, 48.73000000000003240 ) ) ;
#10218=CARTESIAN_POINT ( 'NONE',  ( 5.284464991282756152, -15.10213328493384743, 9.428571428571425272 ) ) ;
#10221=CARTESIAN_POINT ( 'NONE',  ( -13.54758718765249625, -8.512513224245459753, 4.714285714285712636 ) ) ;
#10222=CARTESIAN_POINT ( 'NONE',  ( -15.10213328493390961, 5.284464991282586510, 17.57142857142856940 ) ) ;
#10224=CARTESIAN_POINT ( 'NONE',  ( 1.607813917173037899, -14.26974319298267169, 33.64285714285714590 ) ) ;
#10225=CARTESIAN_POINT ( 'NONE',  ( 14.25515036105622535, -1.737328882695210241, 36.36118342676930126 ) ) ;
ENDSEC;
END-ISO-10303-21;
